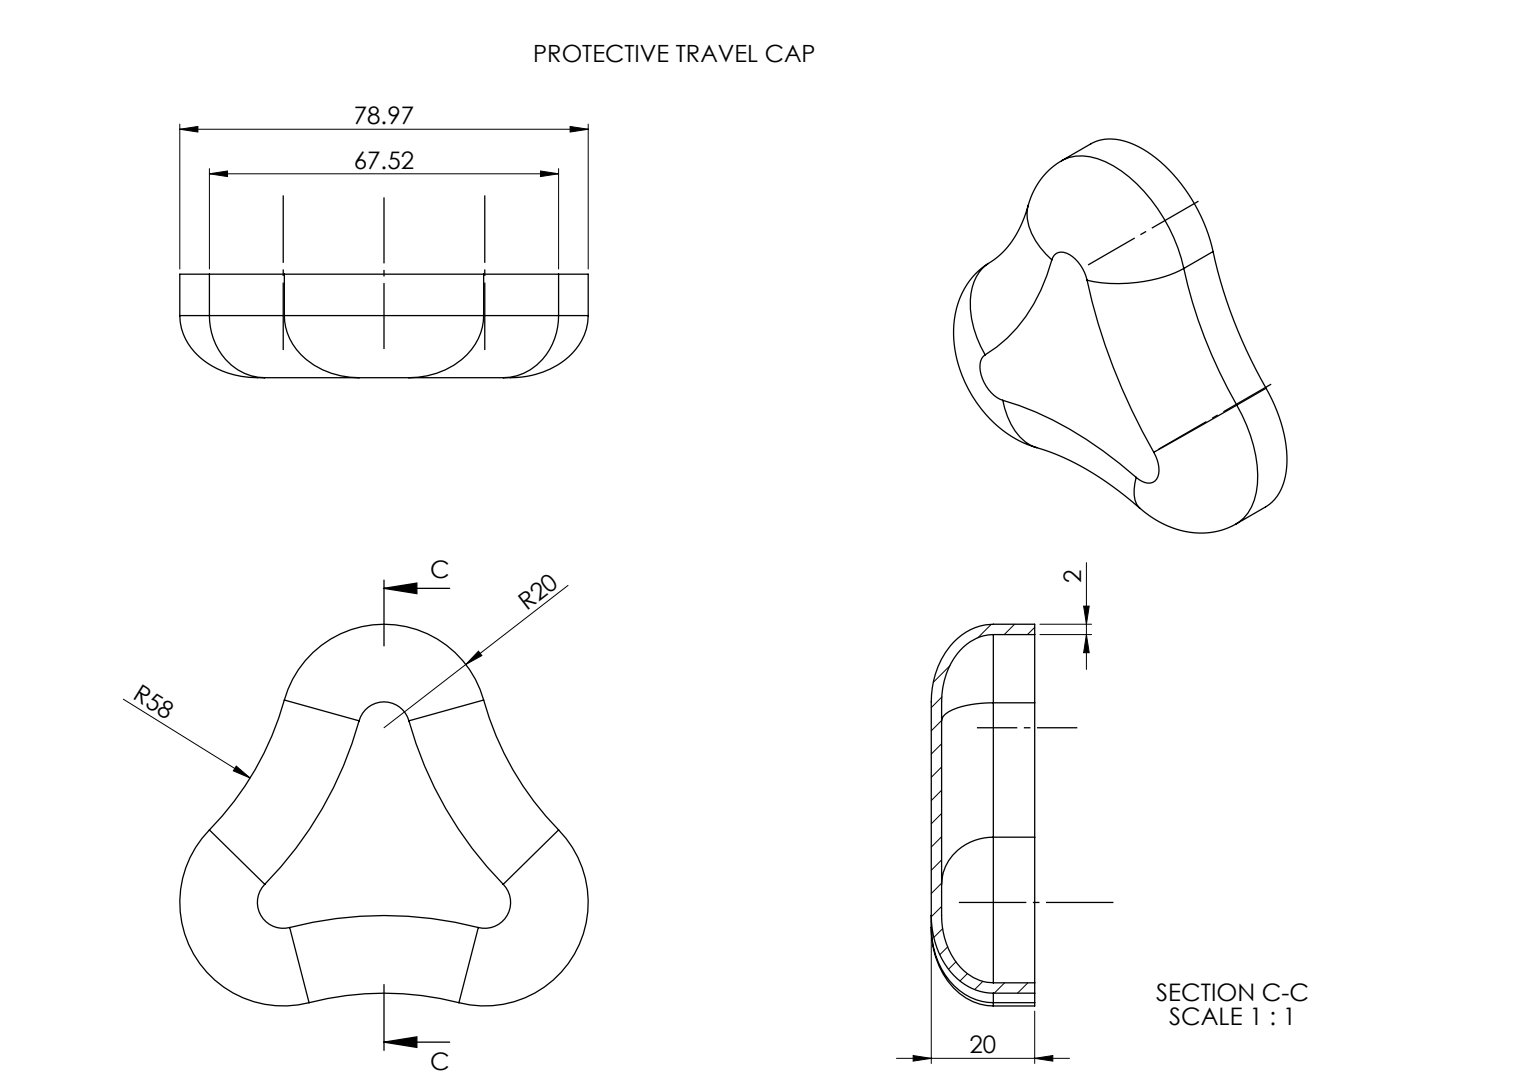
ISO-10303-21;
HEADER;
FILE_DESCRIPTION (('STEP AP214'),
    '1' );
FILE_NAME ('Protective Travel Cap.step',
    '2026-10-04T08:29:30',
    ( '' ),
    ( '' ),
    'SwSTEP 2.0',
    'SolidWorks 2026',
    '' );
FILE_SCHEMA (( 'AUTOMOTIVE_DESIGN' ));
ENDSEC;

DATA;
#17=CARTESIAN_POINT ( 'NONE',  ( 15.81286488304413318, 30.89881296429246760, 12.73282698324844375 ) ) ;
#18=CARTESIAN_POINT ( 'NONE',  ( 18.03924190088647705, -16.85603499720526344, 20.99999999999999645 ) ) ;
#20=CARTESIAN_POINT ( 'NONE',  ( -6.855490822441467458, 29.74656830693323073, 20.25080042701618765 ) ) ;
#37=CARTESIAN_POINT ( 'NONE',  ( -34.17506821248604609, -14.20748230372643484, 17.42190598798392642 ) ) ;
#45=CARTESIAN_POINT ( 'NONE',  ( 5.050662510305749642, -26.77689918168226768, 11.00000000000000178 ) ) ;
#48=PRODUCT_DEFINITION_CONTEXT ( 'detailed design', #8302, 'design' ) ;
#61=CARTESIAN_POINT ( 'NONE',  ( 25.28418022016654021, -25.06680681775964104, 17.42190598798393708 ) ) ;
#75=CARTESIAN_POINT ( 'NONE',  ( 32.33143948541893309, 1.358872982500734405, 11.55979286843934872 ) ) ;
#85=CARTESIAN_POINT ( 'NONE',  ( -20.14416558653889666, -20.32661669692040007, 20.50957957746029336 ) ) ;
#98=ORIENTED_EDGE ( 'NONE', *, *, #25945, .F. ) ;
#112=CARTESIAN_POINT ( 'NONE',  ( 19.16157041420283491, -20.39791322820700259, 20.50957957746027915 ) ) ;
#120=CARTESIAN_POINT ( 'NONE',  ( -33.75875814100324135, 2.759858869446477403, 22.99999999999999645 ) ) ;
#133=CARTESIAN_POINT ( 'NONE',  ( 29.92393930195780527, -26.04303208588360263, 11.00000000000002132 ) ) ;
#144=CARTESIAN_POINT ( 'NONE',  ( -35.54328883424743424, -18.34041411986772019, 13.92931973827826297 ) ) ;
#153=CARTESIAN_POINT ( 'NONE',  ( -20.57776646309937263, 11.88057900678980872, 17.42190598798392998 ) ) ;
#154=VECTOR ( 'NONE', #35200, 1000.000000000000000 ) ;
#161=CARTESIAN_POINT ( 'NONE',  ( 35.73872160561271727, -18.42674013420386459, 13.32518128616613140 ) ) ;
#182=CARTESIAN_POINT ( 'NONE',  ( -2.109373541296176047, 27.06550157850341520, 23.00000000000000000 ) ) ;
#217=CARTESIAN_POINT ( 'NONE',  ( 5.726446540400058183, 39.49945686212564055, 12.14047268033097460 ) ) ;
#221=CARTESIAN_POINT ( 'NONE',  ( 10.34254640628217992, 25.37474234120047001, 19.99202127657103389 ) ) ;
#240=CARTESIAN_POINT ( 'NONE',  ( -22.07435099023991043, -25.45711610480719145, 17.92354375535213151 ) ) ;
#256=DIRECTION ( 'NONE',  ( 0.000000000000000000, 0.000000000000000000, 1.000000000000000000 ) ) ;
#263=CARTESIAN_POINT ( 'NONE',  ( 33.08368474897510225, -6.388390677200520784, 17.92354375535212085 ) ) ;
#268=CARTESIAN_POINT ( 'NONE',  ( 4.441848239913406715, 24.85865334748807953, 21.00000000000000355 ) ) ;
#275=CARTESIAN_POINT ( 'NONE',  ( 17.89938016353245942, 22.15910768081766946, 14.53008259252595025 ) ) ;
#282=ORIENTED_EDGE ( 'NONE', *, *, #11860, .T. ) ;
#285=CARTESIAN_POINT ( 'NONE',  ( -27.67544922579230615, -7.282050787523742130, 20.50957957746029336 ) ) ;
#312=CARTESIAN_POINT ( 'NONE',  ( 27.76392016787571038, -12.00403709334112534, 20.69868183039782039 ) ) ;
#321=CARTESIAN_POINT ( 'NONE',  ( -19.26948696230206082, 27.85601271560033609, 11.00000000000000000 ) ) ;
#346=CARTESIAN_POINT ( 'NONE',  ( -15.07283634910000814, -28.35394831540519789, 13.32518128616608877 ) ) ;
#358=CARTESIAN_POINT ( 'NONE',  ( -13.22866120779437438, 26.17694675927630499, 18.42518152272108978 ) ) ;
#364=CARTESIAN_POINT ( 'NONE',  ( 15.12590024503159114, -28.14827041158712717, 13.92931973827808889 ) ) ;
#373=CARTESIAN_POINT ( 'NONE',  ( 27.36225479881369793, 10.16098284217389924, 11.00000000000000000 ) ) ;
#387=CARTESIAN_POINT ( 'NONE',  ( -8.437494165185018602, 40.76200631401457031, 11.00000000000000000 ) ) ;
#399=DIRECTION ( 'NONE',  ( -0.000000000000000000, -0.000000000000000000, -1.000000000000000000 ) ) ;
#419=CARTESIAN_POINT ( 'NONE',  ( 14.61820604905140897, 32.41591307681830614, 13.32518128616609765 ) ) ;
#423=CARTESIAN_POINT ( 'NONE',  ( 11.83264664767333052, 25.78892025138632604, 19.27171037444156454 ) ) ;
#435=CARTESIAN_POINT ( 'NONE',  ( 14.98890121934557129, -28.67928442654206833, 11.55979286843934517 ) ) ;
#440=CARTESIAN_POINT ( 'NONE',  ( -29.75773323547239002, -22.90830468393550845, 16.87380292611442201 ) ) ;
#448=CARTESIAN_POINT ( 'NONE',  ( -10.09822582592840767, -27.41751403068705883, 11.00000000001392308 ) ) ;
#464=CARTESIAN_POINT ( 'NONE',  ( 32.73576105632422184, -2.961849131989182204, 16.87380292611480215 ) ) ;
#469=CARTESIAN_POINT ( 'NONE',  ( -4.672335726382759624, 24.36080358023105674, 20.99999999999999645 ) ) ;
#484=CARTESIAN_POINT ( 'NONE',  ( -26.84751477640364214, -17.98144108585655232, 20.25080042701566896 ) ) ;
#510=CARTESIAN_POINT ( 'NONE',  ( 26.56332897235214574, -4.302820985782148000, 20.25080042701566541 ) ) ;
#534=DIRECTION ( 'NONE',  ( -0.000000000000000000, -0.000000000000000000, -1.000000000000000000 ) ) ;
#542=CARTESIAN_POINT ( 'NONE',  ( -37.14493776307941175, -9.008680429016052926, 12.73282698324853079 ) ) ;
#551=CARTESIAN_POINT ( 'NONE',  ( 9.401525468405049324, 34.87112330957724282, 16.87380292611441490 ) ) ;
#553=ORIENTED_EDGE ( 'NONE', *, *, #25998, .T. ) ;
#556=CARTESIAN_POINT ( 'NONE',  ( -26.46356280842828212, 3.031871643958657714, 17.42190598798967827 ) ) ;
#558=CARTESIAN_POINT ( 'NONE',  ( 21.42047163595253778, -15.86044052053649978, 20.99999999999999645 ) ) ;
#562=CARTESIAN_POINT ( 'NONE',  ( 34.54872031832756818, -1.828101745486344187, 13.32518128616626640 ) ) ;
#615=CARTESIAN_POINT ( 'NONE',  ( -7.591957726968746378, 38.93640765974107154, 10.99999999999981526 ) ) ;
#619=CARTESIAN_POINT ( 'NONE',  ( 4.864422697791962236, 33.03032433378086807, 19.66345542862529427 ) ) ;
#636=CARTESIAN_POINT ( 'NONE',  ( -32.97049335004036408, -4.716631976066113729, 17.42190598798392998 ) ) ;
#658=CARTESIAN_POINT ( 'NONE',  ( 28.76760616113913827, -24.40467509901337451, 16.30093088680155233 ) ) ;
#663=CARTESIAN_POINT ( 'NONE',  ( 0.6269669233416744758, 28.28960257232503395, 20.99999999999998934 ) ) ;
#670=CARTESIAN_POINT ( 'NONE',  ( 28.79337657215373980, 4.963436916934907295, 11.55979286843148302 ) ) ;
#677=CARTESIAN_POINT ( 'NONE',  ( -23.91569629078610149, -19.26019901638321130, 20.50957957746006954 ) ) ;
#680=ORIENTED_EDGE ( 'NONE', *, *, #28784, .T. ) ;
#706=CARTESIAN_POINT ( 'NONE',  ( 23.63966112704433087, -21.14828014214163687, 19.99202127657103034 ) ) ;
#743=CARTESIAN_POINT ( 'NONE',  ( -37.00900745416922177, -9.025932648522855928, 13.32518128616608699 ) ) ;
#750=CARTESIAN_POINT ( 'NONE',  ( -3.366772934462026523, 37.76190412503627414, 16.87380292611445043 ) ) ;
#753=CARTESIAN_POINT ( 'NONE',  ( -23.79662817865075652, 0.8209266586187062842, 19.66345542862912765 ) ) ;
#756=CARTESIAN_POINT ( 'NONE',  ( 23.05386822411318803, -7.747535282638377652, 23.00000000000000000 ) ) ;
#759=CARTESIAN_POINT ( 'NONE',  ( 35.99085602461089195, -18.53811353976012555, 12.14047268033102611 ) ) ;
#811=CARTESIAN_POINT ( 'NONE',  ( -13.75539757512625272, 34.17605197834731712, 12.14047268033125171 ) ) ;
#814=CARTESIAN_POINT ( 'NONE',  ( 7.971538940948045493, 30.92644086612910570, 19.66345542862527651 ) ) ;
#834=CARTESIAN_POINT ( 'NONE',  ( -35.08888820711664636, -5.671254737730515139, 15.72805884748985861 ) ) ;
#837=ORIENTED_EDGE ( 'NONE', *, *, #21012, .F. ) ;
#854=CARTESIAN_POINT ( 'NONE',  ( -17.47510495690846355, -31.20661830902342615, 11.00000000000000000 ) ) ;
#859=CARTESIAN_POINT ( 'NONE',  ( 35.14638740386845939, -7.516303343517492408, 16.30093088680192892 ) ) ;
#862=CARTESIAN_POINT ( 'NONE',  ( -14.95773623274140895, 28.45553334944834489, 16.30093088680134983 ) ) ;
#864=CARTESIAN_POINT ( 'NONE',  ( -3.456468065140321233, 26.15323006594350019, 20.99999999999998934 ) ) ;
#873=CARTESIAN_POINT ( 'NONE',  ( 14.67741354573947810, 20.96472719003773477, 18.42518152271840037 ) ) ;
#882=CARTESIAN_POINT ( 'NONE',  ( -29.20803623499946511, -13.20745421916120499, 20.25080042701566541 ) ) ;
#903=CARTESIAN_POINT ( 'NONE',  ( -24.37759566069532724, -10.08322588119026797, 23.00000000000000000 ) ) ;
#909=CARTESIAN_POINT ( 'NONE',  ( 30.28108141855193480, -11.05112898844763514, 19.99202127657103034 ) ) ;
#918=FACE_OUTER_BOUND ( 'NONE', #33899, .T. ) ;
#929=ORIENTED_EDGE ( 'NONE', *, *, #21435, .F. ) ;
#935=DIRECTION ( 'NONE',  ( -0.000000000000000000, -0.000000000000000000, -1.000000000000000000 ) ) ;
#945=CARTESIAN_POINT ( 'NONE',  ( -37.38745755834736428, -10.91949489986329347, 12.73282698324913831 ) ) ;
#952=CARTESIAN_POINT ( 'NONE',  ( -15.33540831873584587, 35.51988610398909429, 10.99999999999999822 ) ) ;
#953=CARTESIAN_POINT ( 'NONE',  ( -7.449887436100933513, 34.87105630051663496, 17.92354375535170874 ) ) ;
#958=CARTESIAN_POINT ( 'NONE',  ( -14.79097147050020311, 14.99953367534935822, 19.66345542862526585 ) ) ;
#960=CARTESIAN_POINT ( 'NONE',  ( 20.92112759555554291, -16.07000418475260162, 20.99999999999999645 ) ) ;
#963=CARTESIAN_POINT ( 'NONE',  ( 37.52525227335095082, -10.91693234368658061, 12.14047268033090532 ) ) ;
#1004=ORIENTED_EDGE ( 'NONE', *, *, #36950, .F. ) ;
#1007=CARTESIAN_POINT ( 'NONE',  ( -29.28423149095162259, -1.632116715639065463, 18.42518152272108978 ) ) ;
#1021=CARTESIAN_POINT ( 'NONE',  ( -6.977707682421693924, 31.68171018602201983, 19.66345542862527651 ) ) ;
#1034=CARTESIAN_POINT ( 'NONE',  ( 2.594149110900750621, 26.80855565015184894, 20.99999999999999289 ) ) ;
#1040=CARTESIAN_POINT ( 'NONE',  ( -35.58257249438602798, -10.95300747732907354, 16.30093088680272118 ) ) ;
#1062=CARTESIAN_POINT ( 'NONE',  ( 35.36447994912680315, -9.234655410422998756, 16.30093088680190760 ) ) ;
#1064=CARTESIAN_POINT ( 'NONE',  ( -3.569741787452771042, 38.68155838841067151, 15.72805884748945715 ) ) ;
#1067=CARTESIAN_POINT ( 'NONE',  ( -1.596172877504954402, 27.23837864096127959, 20.99999999999999645 ) ) ;
#1077=CARTESIAN_POINT ( 'NONE',  ( 17.25967040852637169, 21.92197836105680864, 15.72805884747922889 ) ) ;
#1086=CARTESIAN_POINT ( 'NONE',  ( -22.56822310031916956, -21.59793901597470978, 19.99202127657132522 ) ) ;
#1112=CARTESIAN_POINT ( 'NONE',  ( 17.92913371968424840, -21.93458435334546408, 19.99202127657079942 ) ) ;
#1135=CARTESIAN_POINT ( 'NONE',  ( -21.72603204741356109, -16.58852365944958862, 20.99999999999999645 ) ) ;
#1139=VERTEX_POINT ( 'NONE', #39839 ) ;
#1145=CARTESIAN_POINT ( 'NONE',  ( -35.38210723591855356, -3.548218742175161200, 13.32518128616608877 ) ) ;
#1154=CARTESIAN_POINT ( 'NONE',  ( -10.35750558342918737, 33.44896173339029133, 17.42190598798475065 ) ) ;
#1159=CARTESIAN_POINT ( 'NONE',  ( -9.534329713701904296, 19.05805734593735679, 20.69868183039760368 ) ) ;
#1164=CARTESIAN_POINT ( 'NONE',  ( 37.45384686740442248, -12.88771083438643927, 12.14047268033111671 ) ) ;
#1204=EDGE_LOOP ( 'NONE', ( #35292, #7584, #15851, #28195 ) ) ;
#1210=CARTESIAN_POINT ( 'NONE',  ( -32.09165771328038375, 1.123514972298483405, 13.32518128616608344 ) ) ;
#1224=CARTESIAN_POINT ( 'NONE',  ( -7.430899969937648564, 32.27804933232874873, 19.27171037444156099 ) ) ;
#1243=CARTESIAN_POINT ( 'NONE',  ( -20.67781403882173663, -27.68125770801090013, 15.72805884748939498 ) ) ;
#1260=CARTESIAN_POINT ( 'NONE',  ( -30.53342463661827821, -27.99077457432856875, 11.00000000000000178 ) ) ;
#1264=CARTESIAN_POINT ( 'NONE',  ( 32.49165476041698497, -0.9821698610445067645, 15.72805884749123351 ) ) ;
#1266=CARTESIAN_POINT ( 'NONE',  ( -13.24632657851083550, 31.48533120267438079, 16.30093088680190050 ) ) ;
#1267=CARTESIAN_POINT ( 'NONE',  ( -5.218261001347021200, -24.78318996519343997, 16.30093088680190760 ) ) ;
#1269=CARTESIAN_POINT ( 'NONE',  ( 5.067518982750386591, 26.80212859219470189, 20.94377226548378346 ) ) ;
#1274=PRODUCT_DEFINITION_SHAPE ( 'NONE', 'NONE',  #3314 ) ;
#1276=CARTESIAN_POINT ( 'NONE',  ( 19.49168883800135532, 11.25353179758032063, 18.42518152272108978 ) ) ;
#1284=CARTESIAN_POINT ( 'NONE',  ( -29.14609120334281300, -6.569533100116839108, 19.99202127657103389 ) ) ;
#1305=CARTESIAN_POINT ( 'NONE',  ( -33.75875814100331951, 2.759858869446532470, 23.00000000000000000 ) ) ;
#1311=CARTESIAN_POINT ( 'NONE',  ( 28.87886971313727003, -7.891952902956772320, 20.25080042701540251 ) ) ;
#1333=CARTESIAN_POINT ( 'NONE',  ( -24.38721429972438770, -12.23686305972948318, 20.99999999999999645 ) ) ;
#1335=CARTESIAN_POINT ( 'NONE',  ( -19.48557158514998022, -11.24999999999982414, 23.00000000000000000 ) ) ;
#1343=CARTESIAN_POINT ( 'NONE',  ( -16.87498849720621763, -29.16588574430760517, 11.55979286843870035 ) ) ;
#1351=CARTESIAN_POINT ( 'NONE',  ( -37.48557158514991272, -11.24999999999982414, 23.00000000000000000 ) ) ;
#1353=CARTESIAN_POINT ( 'NONE',  ( -1.621626408466260161, 37.48425883190013508, 17.42190598798392642 ) ) ;
#1357=CARTESIAN_POINT ( 'NONE',  ( -8.768078002824983841, 24.93711404285093991, 20.50957957746029336 ) ) ;
#1359=CARTESIAN_POINT ( 'NONE',  ( 24.08646667827959220, -13.28101593840520600, 20.99999999999999645 ) ) ;
#1364=CARTESIAN_POINT ( 'NONE',  ( 32.80061120326785584, -23.42582577749432104, 12.14047268033107407 ) ) ;
#1375=CARTESIAN_POINT ( 'NONE',  ( 17.34253826607195847, 27.32041144403996569, 11.55979286843935405 ) ) ;
#1397=ORIENTED_EDGE ( 'NONE', *, *, #13984, .F. ) ;
#1408=CARTESIAN_POINT ( 'NONE',  ( -32.28722999652026004, 1.315479119632481098, 12.14047268033097637 ) ) ;
#1417=CARTESIAN_POINT ( 'NONE',  ( -1.947644445291408566, 40.50000000000003553, 10.99999999999999822 ) ) ;
#1420=CARTESIAN_POINT ( 'NONE',  ( 13.22866120778972210, 26.17694675929306314, 18.42518152272108622 ) ) ;
#1430=ORIENTED_EDGE ( 'NONE', *, *, #13824, .F. ) ;
#1438=CARTESIAN_POINT ( 'NONE',  ( -18.89970378041276788, -27.81027634888826938, 15.72805884748982130 ) ) ;
#1464=CARTESIAN_POINT ( 'NONE',  ( 29.26100170765755948, -25.10377279866101929, 15.13084544680181942 ) ) ;
#1466=CARTESIAN_POINT ( 'NONE',  ( 6.948689594652316615, 37.54332414141804719, 15.72805884748934169 ) ) ;
#1467=CARTESIAN_POINT ( 'NONE',  ( 4.318754312355916755E-14, -23.13411080437162326, 17.92354375535250810 ) ) ;
#1469=CARTESIAN_POINT ( 'NONE',  ( 8.768078002822827344, 24.93711404285870614, 20.50957957746029692 ) ) ;
#1478=CARTESIAN_POINT ( 'NONE',  ( 24.95394407858722374, 1.780357051442290839, 18.87996532026972218 ) ) ;
#1486=CARTESIAN_POINT ( 'NONE',  ( -31.78757023779102298, -12.37085478034622810, 19.27171037444157875 ) ) ;
#1500=CARTESIAN_POINT ( 'NONE',  ( 34.33271597229073535, -24.82403720151181759, 23.00000000000093792 ) ) ;
#1511=CARTESIAN_POINT ( 'NONE',  ( 32.25947621352486294, -13.82181017473358331, 18.87996532025784546 ) ) ;
#1533=CARTESIAN_POINT ( 'NONE',  ( 10.09822582592851603, -27.41751403068707660, 11.00000000000204814 ) ) ;
#1537=CARTESIAN_POINT ( 'NONE',  ( -21.42047163595255910, -15.86044052053618003, 20.99999999999999645 ) ) ;
#1548=CARTESIAN_POINT ( 'NONE',  ( -29.92393930196035612, -26.04303208588115126, 11.55979286843952103 ) ) ;
#1561=CARTESIAN_POINT ( 'NONE',  ( -19.99288511733821139, -2.332377806177347690, 20.94377226548488125 ) ) ;
#1563=CARTESIAN_POINT ( 'NONE',  ( 23.10579450714144301, -17.79557859931273356, 20.82122704794064916 ) ) ;
#1568=CARTESIAN_POINT ( 'NONE',  ( 36.55626306615705090, -16.65168930787738688, 12.73282698324840823 ) ) ;
#1572=DIRECTION ( 'NONE',  ( -0.000000000000000000, -0.000000000000000000, -1.000000000000000000 ) ) ;
#1624=( BOUNDED_CURVE ( )  B_SPLINE_CURVE ( 2, ( #20187, #30129, #14483 ),
 .UNSPECIFIED., .F., .F. ) 
 B_SPLINE_CURVE_WITH_KNOTS ( ( 3, 3 ),
 ( 0.000000000000000000, 1.000000000000000000 ),
 .UNSPECIFIED. ) 
 CURVE ( )  GEOMETRIC_REPRESENTATION_ITEM ( )  RATIONAL_B_SPLINE_CURVE ( ( 1.000000000000000000, 0.7071067811865474617, 1.000000000000000000 ) ) 
 REPRESENTATION_ITEM ( '' )  );
#1625=CARTESIAN_POINT ( 'NONE',  ( 9.924110812760721601, 32.99075218357499750, 17.92354375535250455 ) ) ;
#1638=CARTESIAN_POINT ( 'NONE',  ( 17.42101839920123041, -19.25229542401860527, 20.69868183039781329 ) ) ;
#1643=CARTESIAN_POINT ( 'NONE',  ( -32.48135758214319679, -20.75321993593849257, 16.30093088680156299 ) ) ;
#1660=CARTESIAN_POINT ( 'NONE',  ( -14.98890121934603314, -28.67928442654204346, 11.00000000000000000 ) ) ;
#1667=CARTESIAN_POINT ( 'NONE',  ( 36.30242391553733228, -14.63578948164456683, 14.53008259254010959 ) ) ;
#1669=CARTESIAN_POINT ( 'NONE',  ( 11.65184672541106359, 34.81748849094131515, 15.13084544680210719 ) ) ;
#1670=CARTESIAN_POINT ( 'NONE',  ( 4.272934335498898793E-14, -21.05812563137664739, 19.27171037444156809 ) ) ;
#1672=CARTESIAN_POINT ( 'NONE',  ( -6.367390439426523940, 24.26983560722021949, 20.94377226548378346 ) ) ;
#1683=CARTESIAN_POINT ( 'NONE',  ( 30.57450045108190650, -0.3656520783221823279, 16.87380292611441490 ) ) ;
#1693=CARTESIAN_POINT ( 'NONE',  ( -27.14644468510475406, -3.730463242939707769, 19.99202127657103389 ) ) ;
#1706=CARTESIAN_POINT ( 'NONE',  ( 25.22779562677032672, -30.53001673900870472, 23.00000000000093792 ) ) ;
#1711=CARTESIAN_POINT ( 'NONE',  ( -23.54493052986492430, -14.21898406159475137, 23.00000000000000000 ) ) ;
#1720=CARTESIAN_POINT ( 'NONE',  ( 30.40813597975501636, -7.345136026722032696, 19.66345542862497098 ) ) ;
#1722=EDGE_LOOP ( 'NONE', ( #16171, #11373, #19448, #17460 ) ) ;
#1730=ADVANCED_FACE ( 'NONE', ( #29809 ), #39146, .F. ) ;
#1734=CYLINDRICAL_SURFACE ( 'NONE', #3431, 20.00000000000003908 ) ;
#1744=CARTESIAN_POINT ( 'NONE',  ( -22.84262768307197788, -16.00844090263207065, 21.00000000000000000 ) ) ;
#1754=CARTESIAN_POINT ( 'NONE',  ( -20.78821643698918109, -29.20280246618806430, 11.55979286843934872 ) ) ;
#1760=CARTESIAN_POINT ( 'NONE',  ( 13.82587227205762481, 37.11292025503284009, 11.00000000000000000 ) ) ;
#1765=CARTESIAN_POINT ( 'NONE',  ( -26.56332897234805301, -4.302820985777816354, 20.25080042701566541 ) ) ;
#1766=CARTESIAN_POINT ( 'NONE',  ( 18.64638308222462371, -17.01267446048655430, 20.99999999999995026 ) ) ;
#1778=FACE_OUTER_BOUND ( 'NONE', #29743, .T. ) ;
#1796=CARTESIAN_POINT ( 'NONE',  ( -24.22337021529747147, -9.561219044741108064, 22.99999999999999289 ) ) ;
#1829=CARTESIAN_POINT ( 'NONE',  ( 8.307596863005482390, 33.43166269068607477, 18.42518152272108978 ) ) ;
#1850=CARTESIAN_POINT ( 'NONE',  ( -29.60586052328872597, -25.59238499872923711, 13.92931973827819725 ) ) ;
#1875=CARTESIAN_POINT ( 'NONE',  ( 34.08416769313340211, -19.67850339273466176, 15.13084544680213739 ) ) ;
#1877=CARTESIAN_POINT ( 'NONE',  ( -5.476246462222815303, 38.75671607062959367, 14.53008259254010959 ) ) ;
#1878=CARTESIAN_POINT ( 'NONE',  ( -10.51283450064414637, -24.98199432659117747, 16.87380292611976884 ) ) ;
#1880=CARTESIAN_POINT ( 'NONE',  ( 3.486159013132950513, 30.04627872069376338, 20.69868183039781684 ) ) ;
#1888=CARTESIAN_POINT ( 'NONE',  ( 15.48226359616410086, 8.938689054910316401, 20.50957957746029336 ) ) ;
#1891=CARTESIAN_POINT ( 'NONE',  ( -3.900486991066764553, 40.17991855517990274, 11.00000000000018474 ) ) ;
#1899=CARTESIAN_POINT ( 'NONE',  ( -29.95834561893252612, -4.698932123269424999, 19.27171037444122703 ) ) ;
#1912=DIRECTION ( 'NONE',  ( -0.000000000000000000, -0.000000000000000000, -1.000000000000000000 ) ) ;
#1917=CARTESIAN_POINT ( 'NONE',  ( -25.22779562677360232, -30.53001673900768864, 11.00000000000000000 ) ) ;
#1924=CARTESIAN_POINT ( 'NONE',  ( 29.45678984391886246, -18.54179626184217611, 19.27171037444156454 ) ) ;
#1946=FACE_OUTER_BOUND ( 'NONE', #40149, .T. ) ;
#1950=CARTESIAN_POINT ( 'NONE',  ( -24.49409870380020848, -11.70597971641812407, 20.99999999999999645 ) ) ;
#1961=CARTESIAN_POINT ( 'NONE',  ( -35.07402885326980879, -20.24999999999981881, 11.00000000000000000 ) ) ;
#1965=ORIENTED_EDGE ( 'NONE', *, *, #20027, .T. ) ;
#1975=CARTESIAN_POINT ( 'NONE',  ( -25.38348611796302734, -5.460896781494596119, 20.69868183039781329 ) ) ;
#1977=CARTESIAN_POINT ( 'NONE',  ( 25.96434769773125240, -12.55439225991619701, 20.94377226548379411 ) ) ;
#2000=CARTESIAN_POINT ( 'NONE',  ( -14.48927117870118408, -30.61587158504671535, 23.00000000000000355 ) ) ;
#2049=CARTESIAN_POINT ( 'NONE',  ( -36.43809855126085750, -10.93713533239294300, 15.13084544680293497 ) ) ;
#2071=CARTESIAN_POINT ( 'NONE',  ( 36.37100582830206719, -12.78888441968064349, 15.13084544680218002 ) ) ;
#2073=CARTESIAN_POINT ( 'NONE',  ( -10.37941170769518529, 36.15788802554169479, 14.53008259254010959 ) ) ;
#2075=CARTESIAN_POINT ( 'NONE',  ( -10.35515495760927784, -25.90830221534925926, 15.72805884749706529 ) ) ;
#2077=CARTESIAN_POINT ( 'NONE',  ( -2.638259136957760820, 30.33190274691516208, 20.69868183039781329 ) ) ;
#2085=CARTESIAN_POINT ( 'NONE',  ( 12.58275666885947075, 13.96078236990229016, 20.50957957746036442 ) ) ;
#2096=CARTESIAN_POINT ( 'NONE',  ( -33.23893881994145261, -12.50319288011963081, 18.42518152272109688 ) ) ;
#2111=CARTESIAN_POINT ( 'NONE',  ( 23.19735768193459791, -14.64350930037804055, 23.00000000000000000 ) ) ;
#2115=CARTESIAN_POINT ( 'NONE',  ( -34.33271597228890215, -24.82403720151341986, 11.00000000000000000 ) ) ;
#2119=CARTESIAN_POINT ( 'NONE',  ( 29.86387254395472723, -6.221772116352023652, 19.66345542862529783 ) ) ;
#2140=CARTESIAN_POINT ( 'NONE',  ( 15.27443809246256734, -27.57253143578338594, 15.13084544680213561 ) ) ;
#2143=CARTESIAN_POINT ( 'NONE',  ( -25.35679574134486813, -6.615406304683630445, 20.82122704794080548 ) ) ;
#2153=CARTESIAN_POINT ( 'NONE',  ( -32.84658669524026919, -23.46788009898592264, 10.99999999999981881 ) ) ;
#2157=CARTESIAN_POINT ( 'NONE',  ( -23.43324262027537586, -8.134040356058612531, 20.99999999999999289 ) ) ;
#2169=CARTESIAN_POINT ( 'NONE',  ( 20.82679397340719873, -18.60878629326332501, 20.82122704794080903 ) ) ;
#2188=CARTESIAN_POINT ( 'NONE',  ( 18.23649648353778474, -16.09146789626167262, 23.00000000000000000 ) ) ;
#2201=CARTESIAN_POINT ( 'NONE',  ( 18.77248996150425597, -31.35432035810270435, 11.00000000000000178 ) ) ;
#2202=MECHANICAL_DESIGN_GEOMETRIC_PRESENTATION_REPRESENTATION('',(#9960),#2829);
#2213=CARTESIAN_POINT ( 'NONE',  ( -24.77298340259705256, 8.359746025953324278, 15.13084544680308419 ) ) ;
#2232=DIRECTION ( 'NONE',  ( -0.000000000000000000, -0.000000000000000000, -1.000000000000000000 ) ) ;
#2250=ORIENTED_EDGE ( 'NONE', *, *, #9412, .T. ) ;
#2268=CARTESIAN_POINT ( 'NONE',  ( 32.59722377598627219, -23.23978988006441782, 13.32518128616629305 ) ) ;
#2270=CARTESIAN_POINT ( 'NONE',  ( 3.781581747449316744, 39.64129210796443203, 13.92931973827821146 ) ) ;
#2274=CARTESIAN_POINT ( 'NONE',  ( 5.140622461635829588, 27.93365566737693229, 20.82122704794079837 ) ) ;
#2282=CARTESIAN_POINT ( 'NONE',  ( 12.61496056324080683, 7.283250877003740520, 20.99999999999999645 ) ) ;
#2285=CARTESIAN_POINT ( 'NONE',  ( -12.44178368932702661, 35.65276919562055014, 11.00000000000005684 ) ) ;
#2295=CARTESIAN_POINT ( 'NONE',  ( -30.59707569446036501, -4.299442758149942811, 18.87996532025748309 ) ) ;
#2309=CARTESIAN_POINT ( 'NONE',  ( 23.43324262027504190, -8.134040356058543253, 23.00000000000000000 ) ) ;
#2318=CARTESIAN_POINT ( 'NONE',  ( 31.03731131719052883, -12.30244853585591969, 19.66345542862526230 ) ) ;
#2330=EDGE_CURVE ( 'NONE', #31697, #24869, #30927, .T. ) ;
#2336=CARTESIAN_POINT ( 'NONE',  ( -4.817371740575545402, 23.83900317890010001, 20.99999999999999645 ) ) ;
#2341=CARTESIAN_POINT ( 'NONE',  ( 10.10865978838830515, -27.35622988134924327, 12.14047268033177573 ) ) ;
#2342=ORIENTED_EDGE ( 'NONE', *, *, #2684, .F. ) ;
#2344=CARTESIAN_POINT ( 'NONE',  ( -26.53285431386355597, -6.841436363529350473, 20.69868183039763210 ) ) ;
#2372=CARTESIAN_POINT ( 'NONE',  ( 22.04303751225581465, -17.34387783897721746, 20.94377226548377280 ) ) ;
#2375=CARTESIAN_POINT ( 'NONE',  ( 37.51589702892713518, -12.89337557385772470, 11.00000000000017053 ) ) ;
#2387=CARTESIAN_POINT ( 'NONE',  ( 14.48927117870126580, -30.61587158504672601, 11.00000000000000000 ) ) ;
#2410=CARTESIAN_POINT ( 'NONE',  ( -27.61482536621095818, 3.986323854238359665, 15.72805884749610428 ) ) ;
#2430=CARTESIAN_POINT ( 'NONE',  ( -3.460024211650461368, 26.15060946995401281, 23.00000000000000355 ) ) ;
#2453=ORIENTED_EDGE ( 'NONE', *, *, #21012, .T. ) ;
#2458=ORIENTED_EDGE ( 'NONE', *, *, #16442, .T. ) ;
#2469=CARTESIAN_POINT ( 'NONE',  ( 34.36757128605636069, -1.941376724489949579, 13.92931973827832159 ) ) ;
#2472=CARTESIAN_POINT ( 'NONE',  ( 10.37941170769460975, 36.15788802554214953, 14.53008259254011136 ) ) ;
#2474=CARTESIAN_POINT ( 'NONE',  ( -17.21213525676645162, -20.06193531423545551, 20.50957957746029336 ) ) ;
#2476=CARTESIAN_POINT ( 'NONE',  ( 7.420252307063369024, 30.34362403113780715, 19.99202127657103745 ) ) ;
#2484=CARTESIAN_POINT ( 'NONE',  ( 20.63240589120021795, -1.802217369567702843, 20.82122704794562296 ) ) ;
#2495=CARTESIAN_POINT ( 'NONE',  ( -24.23816072143619493, -22.57437281311074528, 19.27171037444157164 ) ) ;
#2514=CARTESIAN_POINT ( 'NONE',  ( -18.77248997590677604, -31.35432035705904497, 23.00000000000094147 ) ) ;
#2519=CARTESIAN_POINT ( 'NONE',  ( 33.25367603494935764, -15.60696645161989160, 17.92354375535251521 ) ) ;
#2538=CARTESIAN_POINT ( 'NONE',  ( 4.264734420589964944E-14, -26.44091005802452798, 13.32518128616608877 ) ) ;
#2541=CARTESIAN_POINT ( 'NONE',  ( -17.83459896181207682, -17.64923967996745446, 20.94377226548378346 ) ) ;
#2551=CARTESIAN_POINT ( 'NONE',  ( -19.26948696230207858, 27.85601271560029701, 11.00000000000000000 ) ) ;
#2570=CARTESIAN_POINT ( 'NONE',  ( 27.67544922579167022, -7.282050787522788227, 20.50957957746029336 ) ) ;
#2582=CARTESIAN_POINT ( 'NONE',  ( 12.55429062395116446, 25.98950339719798563, 18.87996532025784546 ) ) ;
#2587=FILL_AREA_STYLE ('',( #24707 ) ) ;
#2600=CARTESIAN_POINT ( 'NONE',  ( 35.27612715351751405, 1.213969564528367906, 10.99999999999999822 ) ) ;
#2609=CARTESIAN_POINT ( 'NONE',  ( -20.66414367076651715, 17.76245163069309640, 11.55979286843749421 ) ) ;
#2656=CYLINDRICAL_SURFACE ( 'NONE', #9592, 58.00000000000007105 ) ;
#2662=CARTESIAN_POINT ( 'NONE',  ( 26.37421498764336292, -27.66411951031065541, 12.73282698324852902 ) ) ;
#2664=CARTESIAN_POINT ( 'NONE',  ( 16.30840571581194354, 28.99314201041919503, 13.92931973827851699 ) ) ;
#2666=CARTESIAN_POINT ( 'NONE',  ( -11.32166530368854929, -20.22988973188854800, 19.99202127657163430 ) ) ;
#2670=CARTESIAN_POINT ( 'NONE',  ( -5.569982264783402748, 31.74975025675326989, 19.99202127657043704 ) ) ;
#2678=CARTESIAN_POINT ( 'NONE',  ( 15.65370567419071079, 2.019989953579482744, 20.99999999999999645 ) ) ;
#2683=ORIENTED_EDGE ( 'NONE', *, *, #21322, .F. ) ;
#2684=EDGE_CURVE ( 'NONE', #24176, #17915, #31549, .T. ) ;
#2687=CARTESIAN_POINT ( 'NONE',  ( -23.42865034949355874, -24.48547250943464348, 18.42518152272145215 ) ) ;
#2710=VECTOR ( 'NONE', #23153, 1000.000000000000000 ) ;
#2711=CARTESIAN_POINT ( 'NONE',  ( 33.10646761238916014, -9.521241417579867417, 18.42518152272108622 ) ) ;
#2712=CIRCLE ( 'NONE', #25401, 19.99999999999993605 ) ;
#2719=CARTESIAN_POINT ( 'NONE',  ( -18.03924190088572388, -16.85603499720483001, 20.99999999999999645 ) ) ;
#2731=CARTESIAN_POINT ( 'NONE',  ( 10.09822582592846096, -27.41751403068768056, 11.55979286844081244 ) ) ;
#2734=CARTESIAN_POINT ( 'NONE',  ( -20.67756819927166134, -17.78966421867582781, 20.94377226548369109 ) ) ;
#2760=CARTESIAN_POINT ( 'NONE',  ( 21.85869495253959371, -19.21667513322869780, 20.69868183039798737 ) ) ;
#2761=CARTESIAN_POINT ( 'NONE',  ( 19.48557158514982746, -11.25000000000009415, 3.000000000000000000 ) ) ;
#2793=CARTESIAN_POINT ( 'NONE',  ( -30.82617745331405246, -24.12092658898454189, 14.53008259254011492 ) ) ;
#2803=CARTESIAN_POINT ( 'NONE',  ( -20.60789226802554808, 17.73598670051888604, 12.14047268032921956 ) ) ;
#2820=ORIENTED_EDGE ( 'NONE', *, *, #6864, .F. ) ;
#2829=( GEOMETRIC_REPRESENTATION_CONTEXT ( 3 ) GLOBAL_UNCERTAINTY_ASSIGNED_CONTEXT ( ( #10802 ) ) GLOBAL_UNIT_ASSIGNED_CONTEXT ( ( #25494, #37301, #31402 ) ) REPRESENTATION_CONTEXT ( 'NONE', 'WORKASPACE' ) );
#2833=FACE_OUTER_BOUND ( 'NONE', #21196, .T. ) ;
#2864=CARTESIAN_POINT ( 'NONE',  ( 1.940950748631622647, 40.43805239114133343, 12.14047268033097815 ) ) ;
#2865=CARTESIAN_POINT ( 'NONE',  ( 6.008588623656380356, -15.38567963534269900, 20.94377226548378701 ) ) ;
#2868=CARTESIAN_POINT ( 'NONE',  ( -8.231369907346209658, 29.48764348321983420, 19.99202127657101258 ) ) ;
#2885=CARTESIAN_POINT ( 'NONE',  ( -28.60197298176802860, -19.58586899272916781, 19.27171037444157520 ) ) ;
#2903=EDGE_LOOP ( 'NONE', ( #37586, #21867, #5252, #24338, #553 ) ) ;
#2907=CARTESIAN_POINT ( 'NONE',  ( 24.28032989564875876, -12.76774640304083164, 21.00000000000001066 ) ) ;
#2908=CARTESIAN_POINT ( 'NONE',  ( 25.04152548477498996, -24.48861404543278653, 17.92354375535251521 ) ) ;
#2919=( BOUNDED_SURFACE ( )  B_SPLINE_SURFACE ( 2, 3, ( 
 ( #5150, #20799, #20193, #8194, #20601, #32999, #29930, #2111, #5348, #38674, #29330, #8596, #10847, #20993, #30136, #14695, #2309, #27086 ),
 ( #23239, #39475, #35632, #11654, #1706, #33401, #5542, #1500, #7790, #32589, #4748, #17155, #14086, #21385, #30542, #18152, #15288, #33792 ),
 ( #17953, #12639, #12042, #28073, #6138, #30338, #27676, #34380, #3097, #18343, #27479, #40063, #8802, #15492, #24630, #33594, #31130, #36825 ) ),
 .UNSPECIFIED., .F., .F., .F. ) 
 B_SPLINE_SURFACE_WITH_KNOTS ( ( 3, 3 ),
 ( 4, 2, 2, 2, 2, 2, 2, 2, 4 ),
 ( 0.000000000000000000, 1.000000000000000000 ),
 ( 4.459899766721548531, 4.784821457936484279, 5.109743149151420027, 5.434664840366355776, 5.759586531581291524, 6.084508222796227273, 6.409429914011163021, 6.734351605226098769, 7.059273296441033629 ),
 .UNSPECIFIED. ) 
 GEOMETRIC_REPRESENTATION_ITEM ( )  RATIONAL_B_SPLINE_SURFACE ( (
 ( 1.000000000000000000, 1.000000000000000000, 1.000000000000000000, 1.000000000000000000, 1.000000000000000000, 1.000000000000000000, 1.000000000000000000, 1.000000000000000000, 1.000000000000000000, 1.000000000000000000, 1.000000000000000000, 1.000000000000000000, 1.000000000000000000, 1.000000000000000000, 1.000000000000000000, 1.000000000000000000, 1.000000000000000000, 1.000000000000000000),
 ( 0.7071067811865474617, 0.7071067811865474617, 0.7071067811865474617, 0.7071067811865474617, 0.7071067811865475727, 0.7071067811865475727, 0.7071067811865475727, 0.7071067811865475727, 0.7071067811865474617, 0.7071067811865474617, 0.7071067811865474617, 0.7071067811865474617, 0.7071067811865474617, 0.7071067811865474617, 0.7071067811865474617, 0.7071067811865474617, 0.7071067811865475727, 0.7071067811865475727),
 ( 1.000000000000000000, 1.000000000000000000, 1.000000000000000000, 1.000000000000000000, 1.000000000000000000, 1.000000000000000000, 1.000000000000000000, 1.000000000000000000, 1.000000000000000000, 1.000000000000000000, 1.000000000000000000, 1.000000000000000000, 1.000000000000000000, 1.000000000000000000, 1.000000000000000000, 1.000000000000000000, 1.000000000000000000, 1.000000000000000000) ) ) 
 REPRESENTATION_ITEM ( '' )  SURFACE ( )  );
#2922=CARTESIAN_POINT ( 'NONE',  ( 25.55085611915419364, 8.900480655592511781, 12.73282698324917384 ) ) ;
#2930=ORIENTED_EDGE ( 'NONE', *, *, #20002, .F. ) ;
#2932=CARTESIAN_POINT ( 'NONE',  ( -24.40183261524807889, -16.82966968839920341, 20.82122704794079837 ) ) ;
#2943=CARTESIAN_POINT ( 'NONE',  ( -14.98890121934612019, -28.67928442654180898, 11.00000000000000000 ) ) ;
#2962=CARTESIAN_POINT ( 'NONE',  ( 24.76266088601874671, -18.72941319223726353, 20.50957957746007310 ) ) ;
#2979=CARTESIAN_POINT ( 'NONE',  ( 6.143904198944455608, -13.77689918168226235, 23.00000000000000000 ) ) ;
#2991=CARTESIAN_POINT ( 'NONE',  ( 27.14644468510626396, -3.730463242941437940, 19.99202127657103745 ) ) ;
#2996=CARTESIAN_POINT ( 'NONE',  ( -36.96658581397586119, -12.84323481469905204, 13.92931973827791836 ) ) ;
#3005=FACE_OUTER_BOUND ( 'NONE', #22440, .T. ) ;
#3008=CARTESIAN_POINT ( 'NONE',  ( 20.91702953749078020, -16.07165331220364735, 23.00000000000000355 ) ) ;
#3030=CARTESIAN_POINT ( 'NONE',  ( 3.456468065140020141, 26.15323006594238464, 23.00000000000000000 ) ) ;
#3050=DIRECTION ( 'NONE',  ( -0.000000000000000000, -0.000000000000000000, -1.000000000000000000 ) ) ;
#3059=CARTESIAN_POINT ( 'NONE',  ( -14.61820604905143384, 32.41591307681827061, 13.32518128616608699 ) ) ;
#3060=CARTESIAN_POINT ( 'NONE',  ( 11.59681349796545824, -18.61320969074927945, 20.50957957745985993 ) ) ;
#3062=CARTESIAN_POINT ( 'NONE',  ( 11.11100267139549658, 25.58833710557466290, 19.66345542862528362 ) ) ;
#3068=CARTESIAN_POINT ( 'NONE',  ( -15.87271491999997863, 26.91186955879524945, 15.72805884748939498 ) ) ;
#3083=CARTESIAN_POINT ( 'NONE',  ( -27.81120771500161837, -23.04947625254830967, 17.92354375535251876 ) ) ;
#3097=CARTESIAN_POINT ( 'NONE',  ( 35.72300736400885057, -23.12593624637960588, 11.00000000000000000 ) ) ;
#3109=CARTESIAN_POINT ( 'NONE',  ( 31.91928157790820109, -18.42860581134451792, 17.92354375535250810 ) ) ;
#3130=CARTESIAN_POINT ( 'NONE',  ( -27.09004689510899766, -14.60731774717074138, 20.69868183039799803 ) ) ;
#3141=ORIENTED_EDGE ( 'NONE', *, *, #7856, .F. ) ;
#3158=EDGE_CURVE ( 'NONE', #10973, #10557, #6006, .T. ) ;
#3160=CARTESIAN_POINT ( 'NONE',  ( 20.97602320185162839, -19.42790811720868049, 20.69868183039782750 ) ) ;
#3170=CARTESIAN_POINT ( 'NONE',  ( -27.36225479880417311, 10.16098284219050107, 11.00000000000000000 ) ) ;
#3195=CARTESIAN_POINT ( 'NONE',  ( -34.92340065173439712, -3.770459477548423699, 14.53008259254011136 ) ) ;
#3207=CARTESIAN_POINT ( 'NONE',  ( -12.60925743039346969, 20.19802119783879490, 19.66345542862530493 ) ) ;
#3216=CIRCLE ( 'NONE', #25910, 58.00000000000007816 ) ;
#3218=CARTESIAN_POINT ( 'NONE',  ( 8.859192577249610068, 12.20922670554003631, 23.00000000000000000 ) ) ;
#3231=CARTESIAN_POINT ( 'NONE',  ( -4.441848239913464447, 24.85865334748893929, 23.00000000000000000 ) ) ;
#3261=CARTESIAN_POINT ( 'NONE',  ( -1.435176708165770409E-13, 40.16401087634232425, 13.32518128616608699 ) ) ;
#3264=CARTESIAN_POINT ( 'NONE',  ( -1.073573824165845014, 32.41755745572908154, 20.25080042701565830 ) ) ;
#3281=CARTESIAN_POINT ( 'NONE',  ( -32.73577250672335026, -2.961872765701405008, 16.87380292611397081 ) ) ;
#3305=CARTESIAN_POINT ( 'NONE',  ( 32.69618749603090890, -17.08296528845530560, 17.92354375535250810 ) ) ;
#3314=PRODUCT_DEFINITION ( 'UNKNOWN', '', #28786, #48 ) ;
#3317=CARTESIAN_POINT ( 'NONE',  ( 25.26292323896833381, 8.700328014641888430, 13.92931973827844416 ) ) ;
#3328=CARTESIAN_POINT ( 'NONE',  ( -27.24589624691908440, -6.395450141004457301, 20.50957957746007665 ) ) ;
#3353=CARTESIAN_POINT ( 'NONE',  ( 26.96432039561798533, -11.11241571815020279, 20.82122704794079837 ) ) ;
#3386=CARTESIAN_POINT ( 'NONE',  ( -15.03860650580583780, -28.48662463501947428, 12.73282698324853257 ) ) ;
#3396=CARTESIAN_POINT ( 'NONE',  ( -16.89748511972594258, 9.755767582500416424, 19.99202127657103389 ) ) ;
#3403=CARTESIAN_POINT ( 'NONE',  ( 36.80210562958740184, -14.73639196410467100, 13.32518128616608877 ) ) ;
#3412=DIRECTION ( 'NONE',  ( -1.000000000000000000, 0.000000000000000000, 0.000000000000000000 ) ) ;
#3425=CARTESIAN_POINT ( 'NONE',  ( 8.437494165184368455, 40.76200631401353291, 22.99999999999999645 ) ) ;
#3431=AXIS2_PLACEMENT_3D ( 'NONE', #20422, #36457, #11077 ) ;
#3438=CARTESIAN_POINT ( 'NONE',  ( -35.48105285891828231, 0.8254987174888869239, 11.00000000000000355 ) ) ;
#3444=EDGE_CURVE ( 'NONE', #8510, #20949, #25043, .T. ) ;
#3459=CARTESIAN_POINT ( 'NONE',  ( 5.638963013753452991, 39.23975437003361577, 13.32518128616608877 ) ) ;
#3460=DIRECTION ( 'NONE',  ( 1.000000000000000000, 0.000000000000000000, 0.000000000000000000 ) ) ;
#3463=CARTESIAN_POINT ( 'NONE',  ( 12.17657648715484164, 27.34841683166593640, 18.87996532025935892 ) ) ;
#3481=CARTESIAN_POINT ( 'NONE',  ( -35.04992612853192924, -12.66836002548420304, 16.87380292611438648 ) ) ;
#3490=EDGE_LOOP ( 'NONE', ( #23406, #39452, #6688, #13183 ) ) ;
#3499=ORIENTED_EDGE ( 'NONE', *, *, #23517, .F. ) ;
#3505=CARTESIAN_POINT ( 'NONE',  ( 33.89025995733786090, -4.271010277521167353, 16.30093088680190760 ) ) ;
#3509=CARTESIAN_POINT ( 'NONE',  ( -2.109373541296185373, 27.06550157850340810, 20.99999999999999645 ) ) ;
#3525=CARTESIAN_POINT ( 'NONE',  ( -26.67038870798852557, -5.578326634890662383, 20.50957957746030402 ) ) ;
#3551=CARTESIAN_POINT ( 'NONE',  ( 27.53764137321996586, -17.13852093243014352, 20.25080042701566541 ) ) ;
#3553=EDGE_CURVE ( 'NONE', #1139, #29890, #9808, .T. ) ;
#3586=CARTESIAN_POINT ( 'NONE',  ( -32.59722377598335896, -23.23978988006665958, 13.32518128616595909 ) ) ;
#3594=CARTESIAN_POINT ( 'NONE',  ( 18.23649648353767461, -16.09146789626181118, 23.00000000000000000 ) ) ;
#3595=CARTESIAN_POINT ( 'NONE',  ( -9.401525468405969477, 34.87112330957656070, 16.87380292611441845 ) ) ;
#3599=CARTESIAN_POINT ( 'NONE',  ( -25.49469310293981295, 2.228649397504699703, 18.42518152272610266 ) ) ;
#3602=CARTESIAN_POINT ( 'NONE',  ( 23.54266556773325192, -14.22277663958715266, 23.00000000000000355 ) ) ;
#3605=CARTESIAN_POINT ( 'NONE',  ( 26.23899120466339951, -27.34191102820725661, 13.92931973827808356 ) ) ;
#3617=DIRECTION ( 'NONE',  ( 0.000000000000000000, 0.000000000000000000, 1.000000000000000000 ) ) ;
#3625=CARTESIAN_POINT ( 'NONE',  ( -17.76739295965290211, 31.93461338995447107, 11.00000000000000000 ) ) ;
#3657=CARTESIAN_POINT ( 'NONE',  ( -12.20958131808417235, 35.40723086407943754, 13.32518128616661812 ) ) ;
#3659=CARTESIAN_POINT ( 'NONE',  ( -4.817371740575545402, 23.83900317890010001, 23.00000000000000000 ) ) ;
#3660=CARTESIAN_POINT ( 'NONE',  ( 6.761248272851016594, 33.72770196150386823, 18.87996532025785257 ) ) ;
#3678=CARTESIAN_POINT ( 'NONE',  ( -34.35058160602017097, -9.363338975649535101, 17.42190598798392998 ) ) ;
#3702=CARTESIAN_POINT ( 'NONE',  ( 18.91633830555523943, -27.33967421372791406, 16.30093088680201419 ) ) ;
#3705=CARTESIAN_POINT ( 'NONE',  ( -3.833852081710641624, 25.75497152300895820, 20.99999999999999645 ) ) ;
#3710=CARTESIAN_POINT ( 'NONE',  ( 25.66376117785140565, 8.978964872295907895, 12.14047268033175797 ) ) ;
#3719=CARTESIAN_POINT ( 'NONE',  ( -27.41073561697751515, -13.75826678483051424, 20.69868183039780618 ) ) ;
#3744=CARTESIAN_POINT ( 'NONE',  ( 16.60464863832688565, -22.41657912773190375, 19.66345542862528362 ) ) ;
#3782=CARTESIAN_POINT ( 'NONE',  ( -36.34524575547219882, -5.221887369237684595, 12.73282698324894824 ) ) ;
#3790=CARTESIAN_POINT ( 'NONE',  ( 3.366772934462163747, 37.76190412503621729, 16.87380292611444688 ) ) ;
#3795=CARTESIAN_POINT ( 'NONE',  ( -11.83264664767723318, 25.78892025137227151, 19.27171037444156809 ) ) ;
#3803=CARTESIAN_POINT ( 'NONE',  ( 34.83525826321752561, -1.648928274806286565, 11.55979286843933984 ) ) ;
#3836=DIRECTION ( 'NONE',  ( -0.000000000000000000, -0.000000000000000000, -1.000000000000000000 ) ) ;
#3837=CARTESIAN_POINT ( 'NONE',  ( -36.90323640188874066, -1.335463057344152604, 10.99999999999999822 ) ) ;
#3847=CARTESIAN_POINT ( 'NONE',  ( -32.33143948541797386, 1.358872982501903248, 11.00000000000000000 ) ) ;
#3850=B_SPLINE_SURFACE_WITH_KNOTS ( 'NONE', 3, 3, ( 
 ( #8903, #24540, #12344, #36532, #34087, #33503, #30644 ),
 ( #33300, #39575, #11951, #39772, #2609, #36936, #11751 ),
 ( #39971, #5645, #18055, #30447, #2803, #15196, #12150 ),
 ( #27586, #9101, #24732, #24135, #21095, #37132, #21488 ),
 ( #17860, #27188, #23939, #14995, #24340, #36738, #30241 ),
 ( #33893, #6046, #6245, #14600, #21295, #15395, #18450 ),
 ( #33700, #5851, #18253, #30839, #9304, #27788, #40172 ),
 ( #21687, #30038, #2213, #26988, #36337, #39376, #11554 ),
 ( #8500, #2410, #14801, #25329, #6832, #31232, #19234 ),
 ( #34485, #22476, #35081, #6631, #31042, #37925, #28782 ),
 ( #37729, #9706, #10097, #25132, #28376, #18649, #27981 ),
 ( #9503, #556, #13132, #153, #22678, #19041, #31432 ),
 ( #37531, #15790, #25729, #28181, #7036, #34681, #22085 ),
 ( #10297, #3599, #21880, #15594, #13335, #34883, #358 ),
 ( #3993, #15995, #19434, #12938, #16195, #9896, #12545 ),
 ( #22276, #31827, #12737, #6440, #31628, #16394, #3795 ),
 ( #28579, #753, #38123, #25525, #958, #3207, #24936 ),
 ( #37329, #34287, #18845, #3396, #16805, #29385, #17006 ),
 ( #1765, #29189, #7235, #17212, #23088, #35488, #7648 ),
 ( #20253, #29587, #10912, #7846, #14149, #29793, #1357 ),
 ( #1975, #32651, #39129, #22878, #4400, #1159, #38527 ),
 ( #7441, #5005, #38934, #26547, #23696, #32031, #20051 ),
 ( #11109, #1561, #13945, #10702, #26130, #4605, #14352 ),
 ( #17418, #35690, #19635, #26339, #4199, #4807, #32446 ),
 ( #38733, #38327, #23493, #23297, #35283, #20458, #35889 ) ),
 .UNSPECIFIED., .F., .F., .F.,
 ( 4, 3, 3, 3, 3, 3, 3, 3, 4 ),
 ( 4, 3, 4 ),
 ( 0.000000000000000000, 0.1250000000000000000, 0.2500000000000000000, 0.3750000000000000000, 0.5000000000000000000, 0.6250000000000000000, 0.7500000000000000000, 0.8750000000000000000, 1.000000000000000000 ),
 ( 5.507097317918141499, 5.759586531581287971, 6.012075745244433556 ),
 .UNSPECIFIED. ) ;
#3858=CARTESIAN_POINT ( 'NONE',  ( -15.98961535660690636, 30.99268274074326257, 10.99999999999966249 ) ) ;
#3861=CARTESIAN_POINT ( 'NONE',  ( -5.983876423895868157, 32.43697950591384682, 19.66345542862462281 ) ) ;
#3876=ORIENTED_EDGE ( 'NONE', *, *, #6864, .T. ) ;
#3878=CARTESIAN_POINT ( 'NONE',  ( -34.49513285232489324, -12.61775564956212570, 17.42190598798391576 ) ) ;
#3895=CARTESIAN_POINT ( 'NONE',  ( -32.93563651212921428, -26.12966208807736379, 11.00000000000000533 ) ) ;
#3900=CARTESIAN_POINT ( 'NONE',  ( 34.64551053920951063, -5.829853277351126017, 16.30093088680154167 ) ) ;
#3902=CARTESIAN_POINT ( 'NONE',  ( 16.24129362380267239, 27.01431713449539629, 15.13084544680213561 ) ) ;
#3905=CARTESIAN_POINT ( 'NONE',  ( -3.503066876656364403, 27.10955750621961258, 20.99999999999998934 ) ) ;
#3909=AXIS2_PLACEMENT_3D ( 'NONE', #38539, #28793, #10712 ) ;
#3912=CARTESIAN_POINT ( 'NONE',  ( 22.19961376577536072, 12.81695298357553270, 15.13084544680213561 ) ) ;
#3921=CARTESIAN_POINT ( 'NONE',  ( -28.51362642450540719, -10.10416295265245878, 20.50957957746029336 ) ) ;
#3947=CARTESIAN_POINT ( 'NONE',  ( 28.61121519738619767, -15.27903652329876394, 20.25080042701566541 ) ) ;
#3951=CARTESIAN_POINT ( 'NONE',  ( 18.23649648353767461, -16.09146789626181118, 23.00000000000000000 ) ) ;
#3967=VERTEX_POINT ( 'NONE', #30098 ) ;
#3974=FACE_OUTER_BOUND ( 'NONE', #3490, .T. ) ;
#3982=CARTESIAN_POINT ( 'NONE',  ( -34.66558941538325200, -1.755063786819271554, 12.73282698324811513 ) ) ;
#3988=CARTESIAN_POINT ( 'NONE',  ( -19.26948696230207858, 27.85601271560029701, 11.00000000000000000 ) ) ;
#3990=CARTESIAN_POINT ( 'NONE',  ( 14.43694901005322961, 26.51279404187409838, 17.42190598798392642 ) ) ;
#3993=CARTESIAN_POINT ( 'NONE',  ( -28.78471548568728977, -2.122417091760708807, 18.87996532025784902 ) ) ;
#3999=CARTESIAN_POINT ( 'NONE',  ( 18.84787193029120544, -29.28148226148236688, 12.14047268033136007 ) ) ;
#4006=ORIENTED_EDGE ( 'NONE', *, *, #20002, .T. ) ;
#4011=DIRECTION ( 'NONE',  ( 1.000000000000000000, -2.775557561562887801E-15, 0.000000000000000000 ) ) ;
#4049=EDGE_CURVE ( 'NONE', #22892, #39914, #33946, .T. ) ;
#4051=CARTESIAN_POINT ( 'NONE',  ( -9.308285395647398985, 37.95628792398468221, 12.14047268033065485 ) ) ;
#4055=CARTESIAN_POINT ( 'NONE',  ( 7.430899969936454852, 32.27804933232965823, 19.27171037444156454 ) ) ;
#4060=AXIS2_PLACEMENT_3D ( 'NONE', #2761, #6205, #39535 ) ;
#4071=CARTESIAN_POINT ( 'NONE',  ( -2.594149110900493937, 26.80855565015070496, 20.99999999999999289 ) ) ;
#4076=CARTESIAN_POINT ( 'NONE',  ( -32.12208287523078099, -1.273987114064245585, 16.30093088680183300 ) ) ;
#4088=VERTEX_POINT ( 'NONE', #18509 ) ;
#4100=CARTESIAN_POINT ( 'NONE',  ( 22.45589477776615084, -27.55224120904853180, 15.72805884748925465 ) ) ;
#4102=CARTESIAN_POINT ( 'NONE',  ( -15.42165057838474063, 26.78649484830226157, 16.30093088680190405 ) ) ;
#4104=CARTESIAN_POINT ( 'NONE',  ( 5.870938322429559264, 25.61771427147129998, 20.94377226548379056 ) ) ;
#4110=CARTESIAN_POINT ( 'NONE',  ( 27.25314217023234775, 3.686469637062584681, 16.30093088681134006 ) ) ;
#4120=CARTESIAN_POINT ( 'NONE',  ( -31.52520841578658306, -13.67397774227592500, 19.27171037444156099 ) ) ;
#4140=CARTESIAN_POINT ( 'NONE',  ( -24.49409870380020848, -11.70597971641812407, 23.00000000000000000 ) ) ;
#4146=CARTESIAN_POINT ( 'NONE',  ( 23.32346807013517775, -20.39486175172845961, 20.25080042701565830 ) ) ;
#4163=EDGE_CURVE ( 'NONE', #14259, #28327, #11470, .T. ) ;
#4173=CARTESIAN_POINT ( 'NONE',  ( 18.84567888139521230, -29.34375185562581478, 11.00000000000044764 ) ) ;
#4184=CARTESIAN_POINT ( 'NONE',  ( -20.74852905477007781, -28.65583854707632128, 13.92931973827808712 ) ) ;
#4193=CARTESIAN_POINT ( 'NONE',  ( -1.257289260074403992E-13, 36.85721162268941242, 17.92354375535250810 ) ) ;
#4199=CARTESIAN_POINT ( 'NONE',  ( -9.576215452290691488, 12.54651180040780289, 20.99999999999999645 ) ) ;
#4202=CARTESIAN_POINT ( 'NONE',  ( 24.38721429972434152, -12.23686305972968924, 20.99999999999999645 ) ) ;
#4205=CARTESIAN_POINT ( 'NONE',  ( 31.38526299860049917, -24.75545609243360801, 11.55979286843934872 ) ) ;
#4228=CARTESIAN_POINT ( 'NONE',  ( -19.26948696230206792, 27.85601271560034320, 22.99999999999999289 ) ) ;
#4258=CARTESIAN_POINT ( 'NONE',  ( 5.746222359017512993, 39.55816310746057241, 11.00000000000000533 ) ) ;
#4259=CARTESIAN_POINT ( 'NONE',  ( 23.05386822411318803, -7.747535282638377652, 20.99999999999999645 ) ) ;
#4261=CARTESIAN_POINT ( 'NONE',  ( 5.180310612586525920, 33.71427074068280660, 19.27171037444157164 ) ) ;
#4274=CARTESIAN_POINT ( 'NONE',  ( 15.60391421430543701, -26.29546805949240351, 16.87380292611441490 ) ) ;
#4280=CARTESIAN_POINT ( 'NONE',  ( -34.31157940325302746, -4.066883398345795264, 15.72805884748939498 ) ) ;
#4299=CARTESIAN_POINT ( 'NONE',  ( -35.94977730715254438, -22.70593821294886183, 10.99999999999999822 ) ) ;
#4303=CARTESIAN_POINT ( 'NONE',  ( 22.37152845209730501, -27.08896763657755002, 16.30093088680180102 ) ) ;
#4306=CARTESIAN_POINT ( 'NONE',  ( 15.87271491999989159, 26.91186955879558695, 15.72805884748939143 ) ) ;
#4308=CARTESIAN_POINT ( 'NONE',  ( 16.60464863833278670, -22.41657912773326444, 19.66345542862528362 ) ) ;
#4310=CARTESIAN_POINT ( 'NONE',  ( 5.410216727984865415, 24.65457866814638876, 21.00000000000019540 ) ) ;
#4316=CARTESIAN_POINT ( 'NONE',  ( 21.86831431663940961, 12.62567715743453967, 15.72805884748939498 ) ) ;
#4325=CARTESIAN_POINT ( 'NONE',  ( -25.09931006221018635, -21.40067874915750323, 19.66345542862498164 ) ) ;
#4346=CARTESIAN_POINT ( 'NONE',  ( -19.30730118283917562, -16.27608008926387839, 23.00000000000000000 ) ) ;
#4350=CARTESIAN_POINT ( 'NONE',  ( 29.18902924043364422, -8.936254945821255902, 20.25080042701565475 ) ) ;
#4386=CARTESIAN_POINT ( 'NONE',  ( -37.51589702892739098, -12.89337557385636579, 11.55979286843906095 ) ) ;
#4395=CARTESIAN_POINT ( 'NONE',  ( -14.00263291006904964, 28.07534605033868402, 17.42190598798347168 ) ) ;
#4400=CARTESIAN_POINT ( 'NONE',  ( -11.82346474097917621, 13.60361205939885565, 20.69868183039782750 ) ) ;
#4409=CARTESIAN_POINT ( 'NONE',  ( 37.51589702892718492, -12.89337557385771049, 11.55979286843950860 ) ) ;
#4443=CARTESIAN_POINT ( 'NONE',  ( -20.92112759555556067, -16.07000418475134040, 21.00000000000000355 ) ) ;
#4452=CARTESIAN_POINT ( 'NONE',  ( -30.57450045107345815, -0.3656520783135126518, 16.87380292611442201 ) ) ;
#4462=CARTESIAN_POINT ( 'NONE',  ( -13.80290580123969058, 34.21636679304901918, 11.00000000000033573 ) ) ;
#4466=CARTESIAN_POINT ( 'NONE',  ( -9.006936242053182440, 32.02107499576991501, 18.87996532025859864 ) ) ;
#4469=CARTESIAN_POINT ( 'NONE',  ( 0.000000000000000000, 0.000000000000000000, 0.000000000000000000 ) ) ;
#4486=CARTESIAN_POINT ( 'NONE',  ( -33.75286824399729824, -19.48722756659376998, 15.72805884748939853 ) ) ;
#4504=CARTESIAN_POINT ( 'NONE',  ( -15.96050091527624559, -30.99544168074540806, 11.00000000000000178 ) ) ;
#4508=CARTESIAN_POINT ( 'NONE',  ( 24.32690616642214465, -27.49953951067901414, 15.13084544680245713 ) ) ;
#4509=EDGE_CURVE ( 'NONE', #16240, #10384, #34157, .T. ) ;
#4511=CARTESIAN_POINT ( 'NONE',  ( -1.732136883777231740, 38.50629078351121137, 16.30093088680190050 ) ) ;
#4513=CARTESIAN_POINT ( 'NONE',  ( 4.327222458066418466E-14, -22.50706359516090060, 18.42518152272108978 ) ) ;
#4515=CARTESIAN_POINT ( 'NONE',  ( 2.374005179830479761, 29.54744178790033260, 20.82122704794079837 ) ) ;
#4520=AXIS2_PLACEMENT_3D ( 'NONE', #37548, #37145, #3412 ) ;
#4523=CARTESIAN_POINT ( 'NONE',  ( 29.28423149095877775, -1.632116715646416472, 18.42518152272108978 ) ) ;
#4530=CARTESIAN_POINT ( 'NONE',  ( -17.92913371968332825, -21.93458435334723333, 19.99202127657105876 ) ) ;
#4550=CARTESIAN_POINT ( 'NONE',  ( -39.05366788732968786, -6.582903524762039993, 22.99999999999811351 ) ) ;
#4555=CARTESIAN_POINT ( 'NONE',  ( 30.12142568021469557, -17.39061322484706196, 19.27171037444156454 ) ) ;
#4592=CARTESIAN_POINT ( 'NONE',  ( -37.34232268491270190, -8.983628415038371173, 11.55979286843934872 ) ) ;
#4605=CARTESIAN_POINT ( 'NONE',  ( -7.976544127345993829, 18.48053530966456037, 20.94377226548371596 ) ) ;
#4613=CARTESIAN_POINT ( 'NONE',  ( 37.14493776307928385, -9.008680429015726077, 12.73282698324853435 ) ) ;
#4624=CARTESIAN_POINT ( 'NONE',  ( 27.36225479889086287, 10.16098284204021240, 10.99999999999999645 ) ) ;
#4649=ORIENTED_EDGE ( 'NONE', *, *, #5889, .T. ) ;
#4654=B_SPLINE_CURVE_WITH_KNOTS ( 'NONE', 3,
 ( #25403, #31705, #28455, #7313, #26005, #1034, #38402, #9973, #25210, #22351, #34757, #16679, #4071, #6908, #37611, #7113, #7517, #22157 ),
 .UNSPECIFIED., .F., .F.,
 ( 4, 2, 2, 2, 2, 2, 2, 2, 4 ),
 ( 0.000000000000000000, 0.1249999999999999445, 0.2499999999999999445, 0.3749999999999999445, 0.4999999999999998890, 0.6249999999999997780, 0.7499999999999998890, 0.8749999999999998890, 1.000000000000000000 ),
 .UNSPECIFIED. ) ;
#4666=CARTESIAN_POINT ( 'NONE',  ( -13.22866120779009336, 26.17694675929174153, 18.42518152272108622 ) ) ;
#4672=CARTESIAN_POINT ( 'NONE',  ( -32.33143948541797386, 1.358872982501903248, 11.00000000000000000 ) ) ;
#4681=ADVANCED_FACE ( 'NONE', ( #28192 ), #29142, .T. ) ;
#4683=EDGE_CURVE ( 'NONE', #4972, #12781, #2712, .T. ) ;
#4686=CARTESIAN_POINT ( 'NONE',  ( -30.37673449013114890, -23.61083502489086428, 15.72805884748940031 ) ) ;
#4711=CARTESIAN_POINT ( 'NONE',  ( 33.75286824399746166, -19.48722756659364919, 15.72805884748939498 ) ) ;
#4714=CARTESIAN_POINT ( 'NONE',  ( -9.968062119478286576, 35.61660815598440166, 15.72805884748939853 ) ) ;
#4715=CARTESIAN_POINT ( 'NONE',  ( -10.93513760491349274, -22.50092802249447033, 18.87996532025975327 ) ) ;
#4717=CARTESIAN_POINT ( 'NONE',  ( -6.606256860318982405, 26.00827479057969072, 20.82122704794080548 ) ) ;
#4724=CARTESIAN_POINT ( 'NONE',  ( 21.05742987670727118, 12.15751280775815424, 16.87380292611441490 ) ) ;
#4733=CARTESIAN_POINT ( 'NONE',  ( -29.86387254395543778, -6.221772116353116111, 19.66345542862528717 ) ) ;
#4739=EDGE_LOOP ( 'NONE', ( #2342, #7493, #38067, #10112 ) ) ;
#4748=CARTESIAN_POINT ( 'NONE',  ( 38.66460482714355607, -17.32098561216399446, 22.99999999999999645 ) ) ;
#4759=CARTESIAN_POINT ( 'NONE',  ( 28.09977684436853806, -21.02662082632513574, 18.87996532025785967 ) ) ;
#4781=CARTESIAN_POINT ( 'NONE',  ( -24.96922908923108508, -9.289876063515562166, 21.00000000000004619 ) ) ;
#4792=CARTESIAN_POINT ( 'NONE',  ( -37.09709568333396845, -7.051483854460184553, 10.99999999999968026 ) ) ;
#4797=ADVANCED_FACE ( 'NONE', ( #21500 ), #18462, .F. ) ;
#4807=CARTESIAN_POINT ( 'NONE',  ( -7.205739717619530360, 18.19477196585663137, 20.99999999999999645 ) ) ;
#4808=CARTESIAN_POINT ( 'NONE',  ( 23.43324262027548599, -8.134040356058102716, 20.99999999999999645 ) ) ;
#4812=CARTESIAN_POINT ( 'NONE',  ( 35.68447701591248489, -3.401722300707758162, 11.00000000000000000 ) ) ;
#4862=CARTESIAN_POINT ( 'NONE',  ( -9.991731067009840928, 30.98181186424739408, 18.87996532025781704 ) ) ;
#4874=B_SPLINE_CURVE_WITH_KNOTS ( 'NONE', 3,
 ( #26550, #20054, #20460, #11111, #19143, #31141, #22377, #28483, #37637, #9406, #2907, #28286, #27686, #21786, #31535, #16098, #37036, #12448 ),
 .UNSPECIFIED., .F., .F.,
 ( 4, 2, 2, 2, 2, 2, 2, 2, 4 ),
 ( 0.000000000000000000, 0.1250000000000000000, 0.2500000000000000000, 0.3750000000000000000, 0.5000000000000000000, 0.6250000000000000000, 0.7500000000000000000, 0.8750000000000000000, 1.000000000000000000 ),
 .UNSPECIFIED. ) ;
#4876=CARTESIAN_POINT ( 'NONE',  ( 16.05557028316289703, -24.54483004364954368, 18.42518152272108978 ) ) ;
#4877=B_SPLINE_CURVE_WITH_KNOTS ( 'NONE', 3,
 ( #23107, #25747, #25545, #4624, #19653, #35506 ),
 .UNSPECIFIED., .F., .F.,
 ( 4, 2, 4 ),
 ( 0.000000000000000000, 0.5000000000000000000, 1.000000000000000000 ),
 .UNSPECIFIED. ) ;
#4883=CARTESIAN_POINT ( 'NONE',  ( -34.59909889755191159, -19.97579906222007295, 13.92931973827808534 ) ) ;
#4885=ADVANCED_FACE ( 'NONE', ( #23306 ), #34894, .T. ) ;
#4909=CARTESIAN_POINT ( 'NONE',  ( 18.88617201209933683, -28.19481557848324726, 15.13084544680231502 ) ) ;
#4911=CARTESIAN_POINT ( 'NONE',  ( -1.888379873391735186, 39.95159812444025249, 13.92931973827808534 ) ) ;
#4913=CARTESIAN_POINT ( 'NONE',  ( 16.05557028316878387, -24.54483004365089371, 18.42518152272108978 ) ) ;
#4917=CARTESIAN_POINT ( 'NONE',  ( 0.9851783940329167377, 31.60047892813805248, 20.50957957746028626 ) ) ;
#4926=CARTESIAN_POINT ( 'NONE',  ( 6.462764152049920163, 17.91932574229958419, 20.99999999999999645 ) ) ;
#4937=CARTESIAN_POINT ( 'NONE',  ( -20.32014898129551739, -22.75198622026924511, 19.66345542862528717 ) ) ;
#4948=ORIENTED_EDGE ( 'NONE', *, *, #9412, .F. ) ;
#4956=CARTESIAN_POINT ( 'NONE',  ( -14.48927117870124093, -30.61587158504648443, 22.99999999999999289 ) ) ;
#4962=CARTESIAN_POINT ( 'NONE',  ( 32.23453252384990719, -8.210301902000198382, 18.87996532025784191 ) ) ;
#4972=VERTEX_POINT ( 'NONE', #30756 ) ;
#4994=CARTESIAN_POINT ( 'NONE',  ( -28.24711154207075481, -27.09388640670391979, 11.00000000000006573 ) ) ;
#5005=CARTESIAN_POINT ( 'NONE',  ( -20.63240589125325641, -1.802217369530700442, 20.82122704794238999 ) ) ;
#5006=CARTESIAN_POINT ( 'NONE',  ( 25.16128423893353627, -12.39270898182871328, 20.99999999999999645 ) ) ;
#5009=CARTESIAN_POINT ( 'NONE',  ( 32.33143948541781043, 1.358872982501757143, 11.55979286843934872 ) ) ;
#5059=ORIENTED_EDGE ( 'NONE', *, *, #5820, .F. ) ;
#5061=ORIENTED_EDGE ( 'NONE', *, *, #5889, .F. ) ;
#5075=CARTESIAN_POINT ( 'NONE',  ( -3.831203748877743731, 25.75875950449070118, 23.00000000000000000 ) ) ;
#5086=CARTESIAN_POINT ( 'NONE',  ( -35.19094867589920028, -3.640833979052929603, 13.92931973827808889 ) ) ;
#5103=CARTESIAN_POINT ( 'NONE',  ( -24.45973306916671319, -28.60230771035024233, 10.99999999999987033 ) ) ;
#5111=CARTESIAN_POINT ( 'NONE',  ( 35.98781724630865142, -12.75392035872628860, 15.72805884748942873 ) ) ;
#5113=CARTESIAN_POINT ( 'NONE',  ( -5.381339405376368568, 38.47497618056175384, 15.13084544680213561 ) ) ;
#5114=CARTESIAN_POINT ( 'NONE',  ( 5.304193131309242304, -23.76115801358234947, 17.42190598798392998 ) ) ;
#5117=CARTESIAN_POINT ( 'NONE',  ( -6.949287954459967942, 25.26733242291857451, 20.82122704794066692 ) ) ;
#5126=CARTESIAN_POINT ( 'NONE',  ( 11.11100267139158859, 25.58833710558854690, 19.66345542862528362 ) ) ;
#5136=CARTESIAN_POINT ( 'NONE',  ( -19.04855072600353338, -23.59522350949000469, 19.27171037444189139 ) ) ;
#5150=CARTESIAN_POINT ( 'NONE',  ( 18.23649648353767461, -16.09146789626181118, 23.00000000000000000 ) ) ;
#5159=CARTESIAN_POINT ( 'NONE',  ( 28.78471548569268279, -2.122417091766370945, 18.87996532025785257 ) ) ;
#5175=DIRECTION ( 'NONE',  ( -0.000000000000000000, -0.000000000000000000, -1.000000000000000000 ) ) ;
#5180=CARTESIAN_POINT ( 'NONE',  ( -10.10865978838755908, -27.35622988135655476, 12.14047268034456017 ) ) ;
#5184=CARTESIAN_POINT ( 'NONE',  ( -19.96384346486619066, -17.84145166816490047, 20.94377226548378346 ) ) ;
#5195=CARTESIAN_POINT ( 'NONE',  ( -37.34232268491268769, -8.983628415038266368, 11.00000000000000000 ) ) ;
#5210=CARTESIAN_POINT ( 'NONE',  ( 20.67756474496276908, -17.78966446931796952, 20.94377226548379056 ) ) ;
#5214=CARTESIAN_POINT ( 'NONE',  ( 33.69589222704783538, -0.03122585499640089662, 11.00000000000003730 ) ) ;
#5241=CARTESIAN_POINT ( 'NONE',  ( 23.09341954621653414, -31.04079623342705574, 11.00000000000000000 ) ) ;
#5252=ORIENTED_EDGE ( 'NONE', *, *, #25945, .T. ) ;
#5280=CARTESIAN_POINT ( 'NONE',  ( 17.83459896181130944, -17.64923967996766052, 20.94377226548378701 ) ) ;
#5284=CARTESIAN_POINT ( 'NONE',  ( -34.99622266290882777, -18.09877784578709026, 15.13084544680241272 ) ) ;
#5308=CARTESIAN_POINT ( 'NONE',  ( 26.00889624226716990, -26.79364542773732083, 15.13084544680213384 ) ) ;
#5310=CARTESIAN_POINT ( 'NONE',  ( 13.38235399890562682, 33.85943911868815093, 13.92931973827816883 ) ) ;
#5313=CARTESIAN_POINT ( 'NONE',  ( -4.288075229729694016, 29.62123851723948675, 20.69868183039744025 ) ) ;
#5315=EDGE_LOOP ( 'NONE', ( #39821, #10489, #17426, #25936 ) ) ;
#5322=CARTESIAN_POINT ( 'NONE',  ( 21.27192666511442098, -1.272056932922072114, 20.69868183040414422 ) ) ;
#5325=CARTESIAN_POINT ( 'NONE',  ( 15.98959510862178668, 30.99271259066394180, 10.99999999999987743 ) ) ;
#5333=CARTESIAN_POINT ( 'NONE',  ( -30.32526513704001303, -2.692717509695762512, 18.42518152272108622 ) ) ;
#5348=CARTESIAN_POINT ( 'NONE',  ( 23.54493052986452284, -14.21898406159493788, 23.00000000000000000 ) ) ;
#5352=CARTESIAN_POINT ( 'NONE',  ( -38.42882785865669604, -4.479089857567689847, 11.00000000000000000 ) ) ;
#5357=CARTESIAN_POINT ( 'NONE',  ( 17.49459433713328593, -24.91609123032452899, 18.42518152272071674 ) ) ;
#5364=CARTESIAN_POINT ( 'NONE',  ( -17.21213525677265821, -20.06193531423681975, 20.50957957746029692 ) ) ;
#5378=CARTESIAN_POINT ( 'NONE',  ( 10.29072928255106234, -26.28675887227032248, 15.13084544680038235 ) ) ;
#5381=CARTESIAN_POINT ( 'NONE',  ( -24.79273775960151482, -6.040746354374424421, 20.82122704794080192 ) ) ;
#5396=CARTESIAN_POINT ( 'NONE',  ( -24.49409870380021204, -11.70597971641812407, 20.99999999999999645 ) ) ;
#5410=CARTESIAN_POINT ( 'NONE',  ( 25.12105899710777024, -7.724472287617720312, 20.94377226548389004 ) ) ;
#5413=CARTESIAN_POINT ( 'NONE',  ( 20.78821643698968913, -29.20280246618838049, 11.00000000000000000 ) ) ;
#5442=CARTESIAN_POINT ( 'NONE',  ( 39.59914439537040209, -10.88071518964973805, 11.00000000000000178 ) ) ;
#5469=CARTESIAN_POINT ( 'NONE',  ( -1.078765555139302945, 27.41260393370252402, 23.00000000000000000 ) ) ;
#5475=CARTESIAN_POINT ( 'NONE',  ( 13.82587226056095986, 37.11292026376941777, 23.00000000000000000 ) ) ;
#5485=ORIENTED_EDGE ( 'NONE', *, *, #29461, .F. ) ;
#5501=CARTESIAN_POINT ( 'NONE',  ( 24.49773858737317767, -28.07267629079924731, 13.92931973827831627 ) ) ;
#5503=CARTESIAN_POINT ( 'NONE',  ( -3.781581747449368258, 39.64129210796443914, 13.92931973827819903 ) ) ;
#5506=CARTESIAN_POINT ( 'NONE',  ( -4.721973484739690363, 30.34170004520404262, 20.50957957745984217 ) ) ;
#5516=CARTESIAN_POINT ( 'NONE',  ( 13.32438941869560800, 7.692839817671511149, 20.94377226548378346 ) ) ;
#5529=CARTESIAN_POINT ( 'NONE',  ( -16.41753675003402790, -23.14183271658250973, 19.27171037444156454 ) ) ;
#5539=ORIENTED_EDGE ( 'NONE', *, *, #22163, .T. ) ;
#5542=CARTESIAN_POINT ( 'NONE',  ( 31.08218589456564018, -27.68808744834087321, 22.99999999999905853 ) ) ;
#5553=CARTESIAN_POINT ( 'NONE',  ( 34.49513285232596616, -12.61775564956195872, 17.42190598798392642 ) ) ;
#5556=AXIS2_PLACEMENT_3D ( 'NONE', #22014, #31953, #10023 ) ;
#5561=CARTESIAN_POINT ( 'NONE',  ( -16.80389827882203235, -21.64427909825945662, 19.99202127657104100 ) ) ;
#5573=CARTESIAN_POINT ( 'NONE',  ( 15.07283634910031189, -28.35394831540551763, 13.32518128616608877 ) ) ;
#5576=CARTESIAN_POINT ( 'NONE',  ( -25.74508372771330755, -9.012464122874943584, 20.94377226548387938 ) ) ;
#5598=CYLINDRICAL_SURFACE ( 'NONE', #18614, 59.99999999999995737 ) ;
#5605=CARTESIAN_POINT ( 'NONE',  ( 23.05386822411317027, -7.747535282638454035, 20.99999999999999645 ) ) ;
#5645=CARTESIAN_POINT ( 'NONE',  ( -28.74551992321994831, 4.923758765708712737, 12.14047268033756666 ) ) ;
#5647=FACE_OUTER_BOUND ( 'NONE', #8545, .T. ) ;
#5704=CARTESIAN_POINT ( 'NONE',  ( 15.03860650580494074, -28.48662463501965192, 12.73282698324853257 ) ) ;
#5706=CARTESIAN_POINT ( 'NONE',  ( -8.747212233150712279, 37.02488667718797899, 15.13084544680138954 ) ) ;
#5710=CARTESIAN_POINT ( 'NONE',  ( 8.883663045967715277, 28.52602195317101064, 19.99202127657103745 ) ) ;
#5719=CARTESIAN_POINT ( 'NONE',  ( 7.976544127178703647, 18.48053530960098811, 20.94377226548381898 ) ) ;
#5730=CARTESIAN_POINT ( 'NONE',  ( -16.05557028316514945, -24.54483004364971777, 18.42518152272108622 ) ) ;
#5750=CARTESIAN_POINT ( 'NONE',  ( -31.08218589456761549, -27.68808744834008451, 23.00000000000000000 ) ) ;
#5756=CARTESIAN_POINT ( 'NONE',  ( 22.07432851697283382, -25.45711773545401613, 17.92354375535248323 ) ) ;
#5761=CARTESIAN_POINT ( 'NONE',  ( 1.596172877504872689, 27.23837864096129735, 21.00000000000000355 ) ) ;
#5774=CARTESIAN_POINT ( 'NONE',  ( -6.462764152204139023, 17.91932574235843134, 20.99999999999999289 ) ) ;
#5778=CARTESIAN_POINT ( 'NONE',  ( -15.12590024502445374, -28.14827041158513055, 13.92931973827808889 ) ) ;
#5781=CARTESIAN_POINT ( 'NONE',  ( -27.79678266235375617, -11.09703717633735742, 20.69868183039817211 ) ) ;
#5790=CARTESIAN_POINT ( 'NONE',  ( -20.57674455326939267, 23.15285302515659893, 11.00000000000000000 ) ) ;
#5801=CARTESIAN_POINT ( 'NONE',  ( 15.01946716906679136, 1.539419383720357137, 23.00000000000000355 ) ) ;
#5809=CARTESIAN_POINT ( 'NONE',  ( 22.68370119258272766, -18.87043823706619250, 20.69868183039780263 ) ) ;
#5820=EDGE_CURVE ( 'NONE', #17915, #20949, #16274, .T. ) ;
#5827=CARTESIAN_POINT ( 'NONE',  ( -14.48927117870118408, -30.61587158504671180, 11.00000000000000000 ) ) ;
#5847=ORIENTED_EDGE ( 'NONE', *, *, #39443, .T. ) ;
#5851=CARTESIAN_POINT ( 'NONE',  ( -28.14004025859599878, 4.421764093230089010, 14.53008259254716705 ) ) ;
#5852=ORIENTED_EDGE ( 'NONE', *, *, #31991, .F. ) ;
#5884=CARTESIAN_POINT ( 'NONE',  ( -39.48557158258395816, -9.956519981528337837, 11.00000000000000178 ) ) ;
#5889=EDGE_CURVE ( 'NONE', #24176, #25190, #11467, .T. ) ;
#5905=CARTESIAN_POINT ( 'NONE',  ( 14.73160032165944777, 32.49283138996950981, 12.73282698324854145 ) ) ;
#5907=CARTESIAN_POINT ( 'NONE',  ( 12.28720923547795429, -14.55658080553756406, 20.99999999999999645 ) ) ;
#5909=CARTESIAN_POINT ( 'NONE',  ( 6.000734348600325063, 30.39614672895685032, 20.25080042701566896 ) ) ;
#5927=CARTESIAN_POINT ( 'NONE',  ( -28.09977684436795187, -21.02662082632541285, 18.87996532025785257 ) ) ;
#5952=CARTESIAN_POINT ( 'NONE',  ( 32.40618899211592918, -4.990034233201372516, 17.92354375535250810 ) ) ;
#5957=CARTESIAN_POINT ( 'NONE',  ( -35.70677476034837383, -3.361263978139850117, 11.00000000000007994 ) ) ;
#5961=CARTESIAN_POINT ( 'NONE',  ( 17.34253826607180216, 27.32041144404034227, 11.00000000000000000 ) ) ;
#5973=CARTESIAN_POINT ( 'NONE',  ( -26.86294352747613345, -10.31366695439962911, 20.82122704794079837 ) ) ;
#5999=CARTESIAN_POINT ( 'NONE',  ( 20.14416558653905298, -20.32661669692072692, 20.50957957746028626 ) ) ;
#6006=CIRCLE ( 'NONE', #4060, 20.00000000000002842 ) ;
#6018=CARTESIAN_POINT ( 'NONE',  ( -9.762440214479841671, -29.39637225272702281, 11.00000000000000000 ) ) ;
#6035=CARTESIAN_POINT ( 'NONE',  ( -36.79828514077309620, -9.052677438811558730, 13.92931973827808712 ) ) ;
#6046=CARTESIAN_POINT ( 'NONE',  ( -28.36971490935763640, 4.612181732483940699, 13.92931973828524406 ) ) ;
#6059=CARTESIAN_POINT ( 'NONE',  ( 4.817371740575477013, 23.83900317890016751, 23.00000000000000000 ) ) ;
#6073=CARTESIAN_POINT ( 'NONE',  ( 2.594149110900750177, 26.80855565015185249, 23.00000000000000000 ) ) ;
#6098=CARTESIAN_POINT ( 'NONE',  ( 14.98890121934609532, -28.67928442654220333, 23.00000000000000000 ) ) ;
#6102=CARTESIAN_POINT ( 'NONE',  ( 10.68781676061647978, 36.56370694841956492, 13.32518128616609054 ) ) ;
#6103=CARTESIAN_POINT ( 'NONE',  ( 4.336808689942017736E-14, -13.77689918168226235, 20.99999999999999645 ) ) ;
#6105=CARTESIAN_POINT ( 'NONE',  ( -10.34254640628272348, 25.37474234119852667, 19.99202127657103389 ) ) ;
#6115=EDGE_CURVE ( 'NONE', #16240, #30744, #35148, .T. ) ;
#6125=CARTESIAN_POINT ( 'NONE',  ( -32.10122455788158646, -20.47530094824154645, 16.87380292611404897 ) ) ;
#6138=CARTESIAN_POINT ( 'NONE',  ( 25.22779562677136767, -30.53001673900894630, 11.00000000000000000 ) ) ;
#6151=CARTESIAN_POINT ( 'NONE',  ( 17.31264644460116031, -26.16430884515622424, 17.42190598798342194 ) ) ;
#6165=CARTESIAN_POINT ( 'NONE',  ( 18.50792845150514765, 22.38468038560473872, 12.73282698322912410 ) ) ;
#6175=CARTESIAN_POINT ( 'NONE',  ( -27.31543141964105104, -5.069059863655038356, 20.25080042701567606 ) ) ;
#6196=ORIENTED_EDGE ( 'NONE', *, *, #36702, .T. ) ;
#6202=CARTESIAN_POINT ( 'NONE',  ( -14.48927117870122316, -30.61587158504648087, 11.00000000000000000 ) ) ;
#6203=CARTESIAN_POINT ( 'NONE',  ( 19.19128484611995944, -19.55740768895475767, 20.69868183039780618 ) ) ;
#6205=DIRECTION ( 'NONE',  ( 0.000000000000000000, 0.000000000000000000, 1.000000000000000000 ) ) ;
#6231=CARTESIAN_POINT ( 'NONE',  ( 27.71565130972689772, -3.171757977843684628, 19.66345542862528717 ) ) ;
#6236=CARTESIAN_POINT ( 'NONE',  ( -34.34163329534256803, -19.82715122747743308, 14.53008259254010959 ) ) ;
#6245=CARTESIAN_POINT ( 'NONE',  ( -25.26292323897049030, 8.700328014641360852, 13.92931973827939096 ) ) ;
#6252=B_SPLINE_CURVE_WITH_KNOTS ( 'NONE', 3,
 ( #27422, #5884, #18289, #6873, #25768, #10336, #3837, #3438, #37967, #6674 ),
 .UNSPECIFIED., .F., .F.,
 ( 4, 2, 2, 2, 4 ),
 ( 0.7014326804499604329, 0.7760745103374703247, 0.8507163402249802164, 0.9253581701124901082, 1.000000000000000000 ),
 .UNSPECIFIED. ) ;
#6258=ADVANCED_FACE ( 'NONE', ( #11769 ), #11376, .T. ) ;
#6259=LINE ( 'NONE', #6645, #7377 ) ;
#6297=CARTESIAN_POINT ( 'NONE',  ( 14.84499459426748835, 32.56974970312070639, 12.14047268033098348 ) ) ;
#6301=CARTESIAN_POINT ( 'NONE',  ( 3.426866961292364788, 32.67295397237175081, 19.99202127657103034 ) ) ;
#6308=DIRECTION ( 'NONE',  ( 0.000000000000000000, 0.000000000000000000, 1.000000000000000000 ) ) ;
#6319=CARTESIAN_POINT ( 'NONE',  ( -22.18736851772318275, -26.07761132199846443, 17.42190598798353562 ) ) ;
#6337=VERTEX_POINT ( 'NONE', #36756 ) ;
#6345=CARTESIAN_POINT ( 'NONE',  ( 31.84188463419212312, -5.263436490337560336, 18.42518152272108978 ) ) ;
#6368=CARTESIAN_POINT ( 'NONE',  ( -27.36681752352253127, -15.80023946406859636, 20.50957957746028626 ) ) ;
#6369=DIRECTION ( 'NONE',  ( -0.000000000000000000, -0.000000000000000000, -1.000000000000000000 ) ) ;
#6395=CARTESIAN_POINT ( 'NONE',  ( 24.27776115474282648, -18.04224162735242842, 20.69868183039762854 ) ) ;
#6431=CARTESIAN_POINT ( 'NONE',  ( -16.90387162101869478, -28.96785393638790396, 12.73282698324800499 ) ) ;
#6440=CARTESIAN_POINT ( 'NONE',  ( -18.23687175285704853, 10.52906281568731472, 19.27171037444156454 ) ) ;
#6447=CARTESIAN_POINT ( 'NONE',  ( 36.59387134601873726, -14.69446750445110794, 13.92931973827808712 ) ) ;
#6466=CARTESIAN_POINT ( 'NONE',  ( -13.82587226055908758, 37.11292026377122255, 11.00000000000000000 ) ) ;
#6495=CARTESIAN_POINT ( 'NONE',  ( -3.887054626305479932, 40.11907545043342083, 12.14047268033113802 ) ) ;
#6499=CARTESIAN_POINT ( 'NONE',  ( -8.489237591500351954, 31.47375793095005037, 19.27171037444226798 ) ) ;
#6516=CARTESIAN_POINT ( 'NONE',  ( -32.69618749603004915, -17.08296528845537665, 17.92354375535288469 ) ) ;
#6541=CARTESIAN_POINT ( 'NONE',  ( 34.71804043165853670, -14.31680059899166757, 16.87380292611441845 ) ) ;
#6546=DIRECTION ( 'NONE',  ( -0.000000000000000000, -0.000000000000000000, -1.000000000000000000 ) ) ;
#6547=CARTESIAN_POINT ( 'NONE',  ( 2.109373541296156063, 27.06550157850343652, 21.00000000000000355 ) ) ;
#6558=EDGE_CURVE ( 'NONE', #17265, #4972, #17662, .T. ) ;
#6562=CARTESIAN_POINT ( 'NONE',  ( -29.18902924043318237, -8.936254945823375095, 20.25080042701515737 ) ) ;
#6588=CARTESIAN_POINT ( 'NONE',  ( 29.65273330788082262, -7.615246293903670249, 19.99202127657073902 ) ) ;
#6620=CARTESIAN_POINT ( 'NONE',  ( -32.18944385490189575, 1.219497045964027748, 12.73282698324853079 ) ) ;
#6627=CARTESIAN_POINT ( 'NONE',  ( -6.176557290856002247, -13.77694981160526844, 23.00000000000000355 ) ) ;
#6628=CARTESIAN_POINT ( 'NONE',  ( 3.246717519899792403, 37.21789761807038133, 17.42190598798394774 ) ) ;
#6631=CARTESIAN_POINT ( 'NONE',  ( -21.46287209667396922, 12.39159498259534686, 16.30093088680190405 ) ) ;
#6641=CARTESIAN_POINT ( 'NONE',  ( 33.82738586796132552, -21.73727074213809729, 13.32518128616604791 ) ) ;
#6643=VECTOR ( 'NONE', #18502, 1000.000000000000000 ) ;
#6645=CARTESIAN_POINT ( 'NONE',  ( -14.98890121934603314, -28.67928442654204346, 23.00000000000000000 ) ) ;
#6646=CARTESIAN_POINT ( 'NONE',  ( 23.05386822411319159, -7.747535282638377652, 23.00000000000000000 ) ) ;
#6660=CARTESIAN_POINT ( 'NONE',  ( 8.437494165185171369, 40.76200631401452767, 11.00000000000000000 ) ) ;
#6674=CARTESIAN_POINT ( 'NONE',  ( -33.75875814100324845, 2.759858869446484064, 11.00000000000000000 ) ) ;
#6688=ORIENTED_EDGE ( 'NONE', *, *, #16721, .F. ) ;
#6692=CARTESIAN_POINT ( 'NONE',  ( 9.308285395644954718, 37.95628792398655094, 12.14047268033102256 ) ) ;
#6694=CARTESIAN_POINT ( 'NONE',  ( -23.05386822411323422, -7.747535282638357224, 23.00000000000000000 ) ) ;
#6695=CARTESIAN_POINT ( 'NONE',  ( -1.329271672591240128, 34.78122644969442945, 19.27171037444156454 ) ) ;
#6713=CARTESIAN_POINT ( 'NONE',  ( -23.78889779961598450, -25.69434382178283371, 17.42190598798429590 ) ) ;
#6737=CARTESIAN_POINT ( 'NONE',  ( 31.01938180032263048, -21.79666295253546338, 16.87380292611479859 ) ) ;
#6741=CARTESIAN_POINT ( 'NONE',  ( -4.441848239913461782, 24.85865334748894284, 20.99999999999999645 ) ) ;
#6750=CARTESIAN_POINT ( 'NONE',  ( 23.18947492591164661, 13.38844959084105568, 11.55979286843934872 ) ) ;
#6758=CARTESIAN_POINT ( 'NONE',  ( -23.32346807013534828, -20.39486175172809013, 20.25080042701566541 ) ) ;
#6784=CARTESIAN_POINT ( 'NONE',  ( 29.77970073067787027, -14.50783476829474594, 19.99202127657104811 ) ) ;
#6808=CARTESIAN_POINT ( 'NONE',  ( 37.58754968649119377, -10.91577297561529036, 10.99999999999992717 ) ) ;
#6820=CARTESIAN_POINT ( 'NONE',  ( -32.28722999652134007, 1.315479119631538074, 12.14047268033097282 ) ) ;
#6829=CARTESIAN_POINT ( 'NONE',  ( 1.621626408465995040, 37.48425883190013508, 17.42190598798392642 ) ) ;
#6832=CARTESIAN_POINT ( 'NONE',  ( -19.27886458632313094, 17.11073565397887819, 15.72805884748862404 ) ) ;
#6839=CARTESIAN_POINT ( 'NONE',  ( 29.80853493429485468, -25.87953118561181753, 12.73282698324837092 ) ) ;
#6844=CARTESIAN_POINT ( 'NONE',  ( 18.74997338758756271, -3.362744936767421589, 23.00000000000000000 ) ) ;
#6860=CARTESIAN_POINT ( 'NONE',  ( -4.331888854854716975, 42.14502281367647640, 23.00000000000000000 ) ) ;
#6864=EDGE_CURVE ( 'NONE', #16240, #18297, #15654, .T. ) ;
#6873=CARTESIAN_POINT ( 'NONE',  ( -38.86091370594022010, -6.124650435543221860, 11.00000000000000000 ) ) ;
#6892=CARTESIAN_POINT ( 'NONE',  ( -12.44178368932711543, 35.65276919562048619, 11.55979286843954057 ) ) ;
#6895=CARTESIAN_POINT ( 'NONE',  ( -10.16357496796715054, 29.39421982382238596, 19.27171037444156454 ) ) ;
#6908=CARTESIAN_POINT ( 'NONE',  ( -3.456468065140303025, 26.15323006594351440, 21.00000000000000000 ) ) ;
#6914=CARTESIAN_POINT ( 'NONE',  ( -31.75251099004362132, -1.565804367082550996, 16.87380292611436872 ) ) ;
#6930=CARTESIAN_POINT ( 'NONE',  ( -25.01235460169770519, -30.53116334361912365, 10.99999999999999822 ) ) ;
#6936=CARTESIAN_POINT ( 'NONE',  ( 35.58257249438514691, -10.95300747732849977, 16.30093088680188629 ) ) ;
#6939=CARTESIAN_POINT ( 'NONE',  ( -13.63376536442988396, 31.74814110635680464, 15.72805884748939143 ) ) ;
#6942=CARTESIAN_POINT ( 'NONE',  ( -2.787905735463278134, 28.53453732066314430, 20.94377226548378701 ) ) ;
#6946=CARTESIAN_POINT ( 'NONE',  ( 28.78471548569376282, -2.122417091767359931, 18.87996532025784546 ) ) ;
#6954=CARTESIAN_POINT ( 'NONE',  ( -26.19533169775672476, -16.15700992729037466, 20.69868183039762144 ) ) ;
#6976=CARTESIAN_POINT ( 'NONE',  ( -23.43324262027536875, -8.134040356058614307, 23.00000000000000000 ) ) ;
#6981=CARTESIAN_POINT ( 'NONE',  ( 17.81343984362198540, -22.72844136247426761, 19.66345542862503137 ) ) ;
#7010=CARTESIAN_POINT ( 'NONE',  ( 32.33143948541787438, 1.358872982501792226, 2.999999999999999112 ) ) ;
#7021=CARTESIAN_POINT ( 'NONE',  ( -37.52525227335131319, -10.91693234368756649, 12.14047268033150573 ) ) ;
#7031=CARTESIAN_POINT ( 'NONE',  ( -11.00933375873403541, 31.84550678200677609, 17.92354375535249389 ) ) ;
#7036=CARTESIAN_POINT ( 'NONE',  ( -17.35626706996358237, 16.20628521381909337, 17.92354375535225586 ) ) ;
#7038=CARTESIAN_POINT ( 'NONE',  ( 19.30730118283918983, -16.27608008926518579, 20.99999999999999645 ) ) ;
#7041=CARTESIAN_POINT ( 'NONE',  ( 20.78373334066920108, -29.14101728923875356, 12.14047268033096927 ) ) ;
#7095=CARTESIAN_POINT ( 'NONE',  ( 3.900486991066101972, 40.17991855518010880, 11.00000000000020250 ) ) ;
#7101=CARTESIAN_POINT ( 'NONE',  ( -9.543723562658518844, 28.97375833662206901, 19.66345542862528362 ) ) ;
#7113=CARTESIAN_POINT ( 'NONE',  ( -4.441848239913464447, 24.85865334748893929, 20.99999999999999645 ) ) ;
#7119=CARTESIAN_POINT ( 'NONE',  ( -18.91631044952799812, -27.33967623494412535, 16.30093088680231972 ) ) ;
#7141=CARTESIAN_POINT ( 'NONE',  ( 32.97049335003973169, -4.716631976065183807, 17.42190598798392998 ) ) ;
#7143=CARTESIAN_POINT ( 'NONE',  ( -12.27395423108443673, 32.91881889271085981, 16.30093088680193603 ) ) ;
#7149=CARTESIAN_POINT ( 'NONE',  ( -1.848241319495560253, 27.98666583367183947, 20.99999999999999645 ) ) ;
#7154=CARTESIAN_POINT ( 'NONE',  ( 21.00262217607745896, 5.738642561615682425, 19.27171037444140111 ) ) ;
#7164=CARTESIAN_POINT ( 'NONE',  ( -27.10945576260561651, -19.90266412673942398, 19.66345542862529072 ) ) ;
#7190=CARTESIAN_POINT ( 'NONE',  ( 22.79731396823020262, -22.36677566318291710, 19.66345542862563178 ) ) ;
#7197=CARTESIAN_POINT ( 'NONE',  ( -7.962467718762158420, 24.71319220551422191, 20.69868183039781329 ) ) ;
#7212=CARTESIAN_POINT ( 'NONE',  ( 32.33143948541787438, 1.358872982501792226, 11.00000000000000000 ) ) ;
#7223=CARTESIAN_POINT ( 'NONE',  ( -16.92376161250139788, -28.83147800495276769, 13.32518128616562869 ) ) ;
#7232=CARTESIAN_POINT ( 'NONE',  ( -1.553811836244973321, 36.85721162268941242, 17.92354375535250810 ) ) ;
#7235=CARTESIAN_POINT ( 'NONE',  ( -19.05502067201149075, 4.384649331638460268, 20.25080042701565830 ) ) ;
#7237=CARTESIAN_POINT ( 'NONE',  ( 19.84741737732757016, -16.23688957394130838, 20.99999999999999645 ) ) ;
#7240=CARTESIAN_POINT ( 'NONE',  ( 26.45121176803958107, -27.84758587393105600, 11.55979286843934695 ) ) ;
#7293=CARTESIAN_POINT ( 'NONE',  ( -9.340438144419696442, 38.00965938231844632, 11.55979286843914799 ) ) ;
#7297=CARTESIAN_POINT ( 'NONE',  ( 1.248251703783664679, 34.03222469610384593, 19.66345542862528362 ) ) ;
#7313=CARTESIAN_POINT ( 'NONE',  ( 3.833852081710638071, 25.75497152300991033, 21.00000000000000355 ) ) ;
#7318=CARTESIAN_POINT ( 'NONE',  ( -34.21349446591933940, -17.75307084757253051, 16.30093088680225222 ) ) ;
#7341=CARTESIAN_POINT ( 'NONE',  ( 35.11176058605620653, -10.96173827525856481, 16.87380292611440424 ) ) ;
#7344=CARTESIAN_POINT ( 'NONE',  ( -11.06388406389812751, 34.19581601475828592, 16.30093088680271052 ) ) ;
#7347=CARTESIAN_POINT ( 'NONE',  ( -2.594149110900493493, 26.80855565015070852, 20.99999999999998934 ) ) ;
#7355=CARTESIAN_POINT ( 'NONE',  ( 23.22986302874564046, 7.287013008514754198, 17.42190598798376300 ) ) ;
#7364=CARTESIAN_POINT ( 'NONE',  ( -28.59012753014036790, -4.062670752122675921, 19.66345542862530493 ) ) ;
#7373=ADVANCED_FACE ( 'NONE', ( #32818 ), #1734, .T. ) ;
#7377=VECTOR ( 'NONE', #12951, 1000.000000000000000 ) ;
#7391=CARTESIAN_POINT ( 'NONE',  ( 28.07442828530308176, -16.20877872786445195, 20.25080042701566541 ) ) ;
#7402=CYLINDRICAL_SURFACE ( 'NONE', #37640, 57.99999999999995737 ) ;
#7425=CARTESIAN_POINT ( 'NONE',  ( -14.98890121934590347, -28.67928442654175214, 11.55979286843934872 ) ) ;
#7435=CARTESIAN_POINT ( 'NONE',  ( -6.320269494896706419, 36.18253918181394369, 17.42190598798392287 ) ) ;
#7441=CARTESIAN_POINT ( 'NONE',  ( -24.79273775960036019, -6.040746354373381699, 20.82122704794079837 ) ) ;
#7443=DIRECTION ( 'NONE',  ( -1.000000000000000000, 0.000000000000000000, 0.000000000000000000 ) ) ;
#7447=CARTESIAN_POINT ( 'NONE',  ( 14.98890121934557307, -28.67928442654207188, 11.55979286843934872 ) ) ;
#7474=CARTESIAN_POINT ( 'NONE',  ( -20.39213822642799201, -16.19729952584802035, 22.99999999999999645 ) ) ;
#7493=ORIENTED_EDGE ( 'NONE', *, *, #29461, .T. ) ;
#7501=CARTESIAN_POINT ( 'NONE',  ( 16.82090372984156801, 29.19711159930561450, 11.55979286843845877 ) ) ;
#7504=CARTESIAN_POINT ( 'NONE',  ( -12.55429062395159079, 25.98950339719647218, 18.87996532025784546 ) ) ;
#7517=CARTESIAN_POINT ( 'NONE',  ( -4.672335726382761401, 24.36080358023105674, 20.99999999999999645 ) ) ;
#7524=CARTESIAN_POINT ( 'NONE',  ( -22.37155630812419105, -27.08896561536066372, 16.30093088680148838 ) ) ;
#7550=CARTESIAN_POINT ( 'NONE',  ( 35.45120626212618475, -5.541700984529022378, 15.13084544680181587 ) ) ;
#7552=CARTESIAN_POINT ( 'NONE',  ( -9.684793793942127138, 35.24386573278048473, 16.30093088680190760 ) ) ;
#7553=CARTESIAN_POINT ( 'NONE',  ( 10.60610353952458773, -24.43405348869776006, 17.42190598798185164 ) ) ;
#7555=CARTESIAN_POINT ( 'NONE',  ( 3.998720052559921356, 27.76176938167571961, 20.94377226548378346 ) ) ;
#7563=CARTESIAN_POINT ( 'NONE',  ( 14.43694901004736586, 26.51279404189499900, 17.42190598798392998 ) ) ;
#7571=CARTESIAN_POINT ( 'NONE',  ( -24.71109915376977284, -20.69862126830784277, 19.99202127657074612 ) ) ;
#7584=ORIENTED_EDGE ( 'NONE', *, *, #16442, .F. ) ;
#7592=CARTESIAN_POINT ( 'NONE',  ( -36.53988293555860878, -0.5802930328944716498, 22.99999999999905853 ) ) ;
#7597=CARTESIAN_POINT ( 'NONE',  ( 23.22759628179494484, -23.81077309377013762, 18.87996532025824337 ) ) ;
#7621=CARTESIAN_POINT ( 'NONE',  ( 22.73075399258359397, -29.06185307675098883, 10.99999999999956124 ) ) ;
#7632=CARTESIAN_POINT ( 'NONE',  ( -22.71963042674493138, -29.00054972838716338, 12.14047268033060156 ) ) ;
#7648=CARTESIAN_POINT ( 'NONE',  ( -9.555312204555107769, 25.15592819202021246, 20.25080042701566541 ) ) ;
#7650=CARTESIAN_POINT ( 'NONE',  ( 24.49409870379991716, -11.70597971641857526, 20.99999999999999645 ) ) ;
#7655=CARTESIAN_POINT ( 'NONE',  ( 36.53369576860747259, -5.154516326609281052, 11.55979286843935760 ) ) ;
#7707=CARTESIAN_POINT ( 'NONE',  ( -3.900486991066871578, 40.17991855517983879, 11.00000000000019007 ) ) ;
#7711=CARTESIAN_POINT ( 'NONE',  ( 10.52848948537593721, 31.43736604633500065, 18.42518152272110044 ) ) ;
#7729=CARTESIAN_POINT ( 'NONE',  ( -15.37000524125038048, -27.20210912714571805, 15.72805884748939498 ) ) ;
#7751=CARTESIAN_POINT ( 'NONE',  ( 20.72701401736302529, -28.35932241216985972, 14.53008259254010959 ) ) ;
#7753=CARTESIAN_POINT ( 'NONE',  ( 15.75274587708552154, 28.77197995862663760, 15.13084544680308063 ) ) ;
#7754=CARTESIAN_POINT ( 'NONE',  ( -16.23042486172771248, -23.86708630543029130, 18.87996532025784902 ) ) ;
#7756=CARTESIAN_POINT ( 'NONE',  ( 0.8051564177163211822, 29.93655406406124797, 20.82122704794079837 ) ) ;
#7757=VECTOR ( 'NONE', #5175, 1000.000000000000000 ) ;
#7766=CARTESIAN_POINT ( 'NONE',  ( 31.72789954390927392, 0.7664678198816438082, 14.53008259254011136 ) ) ;
#7776=CARTESIAN_POINT ( 'NONE',  ( -29.36302367423271065, -15.61102309902027585, 19.99202127657132877 ) ) ;
#7790=CARTESIAN_POINT ( 'NONE',  ( 35.72300736400854504, -23.12593624637943179, 22.99999999999999289 ) ) ;
#7799=VERTEX_POINT ( 'NONE', #23161 ) ;
#7802=CARTESIAN_POINT ( 'NONE',  ( 17.59613548593226540, -24.21943298483269302, 18.87996532025752217 ) ) ;
#7833=CARTESIAN_POINT ( 'NONE',  ( -32.33143948541798096, 1.358872982501892590, 11.00000000000000000 ) ) ;
#7846=CARTESIAN_POINT ( 'NONE',  ( -15.48226359616454495, 8.938689054909644938, 20.50957957746029336 ) ) ;
#7847=CARTESIAN_POINT ( 'NONE',  ( 25.43307211745627328, -8.368469763667489403, 20.94377226548379411 ) ) ;
#7852=CARTESIAN_POINT ( 'NONE',  ( 22.73075399258386398, -29.06185307675093199, 10.99999999999955769 ) ) ;
#7856=EDGE_CURVE ( 'NONE', #17014, #18163, #15579, .T. ) ;
#7908=CARTESIAN_POINT ( 'NONE',  ( -12.17657648715623608, 27.34841683166460058, 18.87996532025750085 ) ) ;
#7926=CARTESIAN_POINT ( 'NONE',  ( -33.86051255203334875, -2.258496953481841096, 15.13084544680166665 ) ) ;
#7941=CARTESIAN_POINT ( 'NONE',  ( -32.57473823703268323, -23.68076927422058731, 10.99999999999993960 ) ) ;
#7942=UNCERTAINTY_MEASURE_WITH_UNIT (LENGTH_MEASURE( 1.000000000000000082E-05 ), #36754, 'distance_accuracy_value', 'NONE');
#7949=CARTESIAN_POINT ( 'NONE',  ( 34.31157940325252298, -4.066883398345114919, 15.72805884748939853 ) ) ;
#7951=CARTESIAN_POINT ( 'NONE',  ( 14.19638663437042503, 32.12978188971815285, 14.53008259254012025 ) ) ;
#7952=CARTESIAN_POINT ( 'NONE',  ( 10.43399472913278103, -25.44514827092724829, 16.30093088679983637 ) ) ;
#7954=CARTESIAN_POINT ( 'NONE',  ( 8.084325832714235105, 26.79336336920809813, 20.50957957746030047 ) ) ;
#7960=VECTOR ( 'NONE', #1912, 1000.000000000000000 ) ;
#7962=CARTESIAN_POINT ( 'NONE',  ( 14.04126239388501496, 8.106726622871901711, 20.82122704794079837 ) ) ;
#7972=CARTESIAN_POINT ( 'NONE',  ( -26.17288861939861988, -20.72787579792414903, 19.66345542862528362 ) ) ;
#7993=CARTESIAN_POINT ( 'NONE',  ( -29.22254794994760729, -28.85350742528338586, 22.99999999999905853 ) ) ;
#7999=CARTESIAN_POINT ( 'NONE',  ( 23.01245512501257551, -23.08877437847652558, 19.27171037444193757 ) ) ;
#8025=CARTESIAN_POINT ( 'NONE',  ( -21.91981567634955397, -15.65087685632102499, 20.99999999999999645 ) ) ;
#8035=CARTESIAN_POINT ( 'NONE',  ( -34.10020663062397972, -21.93670956716203690, 11.00000000000017231 ) ) ;
#8049=CARTESIAN_POINT ( 'NONE',  ( 22.70288158165702086, -17.06695585772177992, 20.94377226548368043 ) ) ;
#8107=CARTESIAN_POINT ( 'NONE',  ( -4.383143208095260590, 35.51174355874280053, 18.42518152272109333 ) ) ;
#8111=( LENGTH_UNIT ( ) NAMED_UNIT ( * ) SI_UNIT ( .MILLI., .METRE. ) );
#8127=CARTESIAN_POINT ( 'NONE',  ( -26.23899120466318280, -27.34191102820705055, 13.92931973827808534 ) ) ;
#8153=CARTESIAN_POINT ( 'NONE',  ( 18.87563634320844130, -28.49365729390225965, 14.53008259254033163 ) ) ;
#8156=CARTESIAN_POINT ( 'NONE',  ( -10.19952947928024933, 35.92118758406519419, 15.13084544680213384 ) ) ;
#8157=CARTESIAN_POINT ( 'NONE',  ( 5.178899460637698127, -25.25135431486990711, 15.72805884748939853 ) ) ;
#8159=CARTESIAN_POINT ( 'NONE',  ( 1.610977985362757936, 29.80447555512223445, 20.82122704794079482 ) ) ;
#8170=CARTESIAN_POINT ( 'NONE',  ( 7.164929079092710928, 24.49151390637290149, 20.82122704794079837 ) ) ;
#8180=CARTESIAN_POINT ( 'NONE',  ( -21.83517059620288236, -24.14399886393494299, 18.87996532025750795 ) ) ;
#8194=CARTESIAN_POINT ( 'NONE',  ( 20.38753357181587234, -16.19769905861744519, 23.00000000000000000 ) ) ;
#8199=CARTESIAN_POINT ( 'NONE',  ( -34.33271597228865346, -24.82403720151219417, 23.00000000000000000 ) ) ;
#8206=CARTESIAN_POINT ( 'NONE',  ( 30.59706755222660135, -4.299425952516082283, 18.87996532025822916 ) ) ;
#8207=AXIS2_PLACEMENT_3D ( 'NONE', #26275, #13886, #32175 ) ;
#8226=CARTESIAN_POINT ( 'NONE',  ( -5.067385705950865571, -26.57793081542402547, 12.73282698324853257 ) ) ;
#8229=AXIS2_PLACEMENT_3D ( 'NONE', #28619, #3836, #16237 ) ;
#8230=CARTESIAN_POINT ( 'NONE',  ( -24.51396478725073536, -11.15767879383071737, 20.99999999999999645 ) ) ;
#8239=CARTESIAN_POINT ( 'NONE',  ( -31.34430980808800626, -24.70897660846286570, 12.14047268033097282 ) ) ;
#8253=CARTESIAN_POINT ( 'NONE',  ( 21.72603204741341898, -16.58852365944996166, 20.99999999999999645 ) ) ;
#8258=AXIS2_PLACEMENT_3D ( 'NONE', #21779, #256, #25032 ) ;
#8259=CIRCLE ( 'NONE', #12149, 17.99999999999993250 ) ;
#8287=CARTESIAN_POINT ( 'NONE',  ( 25.22779561345564758, -30.53001674459726189, 11.00000000000000178 ) ) ;
#8295=B_SPLINE_CURVE_WITH_KNOTS ( 'NONE', 3,
 ( #22171, #21771, #45, #16283, #448, #9985 ),
 .UNSPECIFIED., .F., .F.,
 ( 4, 2, 4 ),
 ( 0.000000000000000000, 0.5000000000000000000, 1.000000000000000000 ),
 .UNSPECIFIED. ) ;
#8296=VERTEX_POINT ( 'NONE', #19063 ) ;
#8300=B_SPLINE_CURVE_WITH_KNOTS ( 'NONE', 3,
 ( #26737, #24484, #5801, #29985, #36292, #33253 ),
 .UNSPECIFIED., .F., .F.,
 ( 4, 2, 4 ),
 ( 0.000000000000000000, 0.5000000000000000000, 1.000000000000000000 ),
 .UNSPECIFIED. ) ;
#8302=APPLICATION_CONTEXT ( 'automotive_design' ) ;
#8318=CARTESIAN_POINT ( 'NONE',  ( 17.34253826607184479, 27.32041144404033162, 11.00000000000000000 ) ) ;
#8339=CARTESIAN_POINT ( 'NONE',  ( -36.37100582830133533, -12.78888441968056000, 15.13084544680203258 ) ) ;
#8354=CARTESIAN_POINT ( 'NONE',  ( -35.04557732017523364, -20.40215588137732894, 10.99999999999994138 ) ) ;
#8362=CARTESIAN_POINT ( 'NONE',  ( 29.43343111547206448, -25.34807889869614073, 14.53008259253982892 ) ) ;
#8364=CARTESIAN_POINT ( 'NONE',  ( -3.717128218779113702, 39.34929362537324948, 14.53008259254020551 ) ) ;
#8365=CARTESIAN_POINT ( 'NONE',  ( 4.276224980513730623E-14, -25.25135431486990711, 15.72805884748939853 ) ) ;
#8367=CARTESIAN_POINT ( 'NONE',  ( 2.905187527479470067, 31.12430299512154264, 20.50957957746028626 ) ) ;
#8378=CARTESIAN_POINT ( 'NONE',  ( 11.08993573033173696, 19.63476728479018973, 20.25080042701548777 ) ) ;
#8389=CARTESIAN_POINT ( 'NONE',  ( -32.48980236688448997, -6.600743665353513201, 18.42518152272148413 ) ) ;
#8414=CARTESIAN_POINT ( 'NONE',  ( 16.05557028316289347, -24.54483004364954368, 18.42518152272108622 ) ) ;
#8433=CARTESIAN_POINT ( 'NONE',  ( -5.050662510305666153, -26.77689918168226058, 11.00000000000000000 ) ) ;
#8437=CARTESIAN_POINT ( 'NONE',  ( -24.20198940123846398, -6.620595927252818313, 20.94377226548378701 ) ) ;
#8461=CARTESIAN_POINT ( 'NONE',  ( 22.36336935241927293, -18.10715803802170498, 20.82122704794078771 ) ) ;
#8500=CARTESIAN_POINT ( 'NONE',  ( -31.24272016124701068, 0.2902395683534709780, 15.72805884748939853 ) ) ;
#8510=VERTEX_POINT ( 'NONE', #23513 ) ;
#8540=B_SPLINE_CURVE_WITH_KNOTS ( 'NONE', 3,
 ( #13416, #435, #31508, #25810, #38205, #32109, #10377, #4274, #10779, #4876, #36366, #32926, #14020, #29860, #1638, #5280, #20328, #16884 ),
 .UNSPECIFIED., .F., .F.,
 ( 4, 2, 2, 2, 2, 2, 2, 2, 4 ),
 ( 0.000000000000000000, 0.1250000000000000000, 0.2500000000000000000, 0.3750000000000000000, 0.5000000000000000000, 0.6250000000000000000, 0.7500000000000000000, 0.8750000000000000000, 1.000000000000000000 ),
 .UNSPECIFIED. ) ;
#8545=EDGE_LOOP ( 'NONE', ( #15980, #6196, #4006, #35706 ) ) ;
#8556=CARTESIAN_POINT ( 'NONE',  ( 35.54328883424830110, -18.34041411986698478, 13.92931973827811909 ) ) ;
#8558=CARTESIAN_POINT ( 'NONE',  ( -1.387327393066717074E-13, 39.65430245495500117, 14.53008259254011136 ) ) ;
#8561=CARTESIAN_POINT ( 'NONE',  ( -1.971557875515829616, 31.43880600153361371, 20.50957957746028271 ) ) ;
#8563=VERTEX_POINT ( 'NONE', #11330 ) ;
#8568=CARTESIAN_POINT ( 'NONE',  ( 24.79273775960175996, -6.040746354374877392, 20.82122704794079837 ) ) ;
#8580=CARTESIAN_POINT ( 'NONE',  ( -29.77271197308770212, -3.128983846831010496, 18.87996532025785967 ) ) ;
#8596=CARTESIAN_POINT ( 'NONE',  ( 24.49409870379991716, -11.70597971641860191, 23.00000000000000000 ) ) ;
#8607=CARTESIAN_POINT ( 'NONE',  ( 22.18734415243709179, -26.07761308992911964, 17.42190598798388379 ) ) ;
#8627=CARTESIAN_POINT ( 'NONE',  ( 18.23649648353767461, -16.09146789626181118, 23.00000000000000000 ) ) ;
#8631=CARTESIAN_POINT ( 'NONE',  ( -15.03860650580051761, -28.48662463501835163, 12.73282698324853257 ) ) ;
#8632=ORIENTED_EDGE ( 'NONE', *, *, #17283, .T. ) ;
#8634=CARTESIAN_POINT ( 'NONE',  ( -25.82310832280115775, -13.25591304976905427, 20.94377226548378346 ) ) ;
#8647=CARTESIAN_POINT ( 'NONE',  ( -18.76090689389219435, -16.22676322417297357, 21.00000000000000000 ) ) ;
#8662=CARTESIAN_POINT ( 'NONE',  ( 25.03753813966995168, -13.00734255224419655, 20.99999999999999645 ) ) ;
#8664=CARTESIAN_POINT ( 'NONE',  ( 34.83525826321753271, -1.648928274806267025, 10.99999999999992006 ) ) ;
#8693=CARTESIAN_POINT ( 'NONE',  ( 31.08218588373089020, -27.68808745788718895, 11.00000000000000178 ) ) ;
#8720=( NAMED_UNIT ( * ) SI_UNIT ( $, .STERADIAN. ) SOLID_ANGLE_UNIT ( ) );
#8722=CARTESIAN_POINT ( 'NONE',  ( 19.48557158514982746, -11.25000000000009415, 23.00000000000000000 ) ) ;
#8736=FACE_OUTER_BOUND ( 'NONE', #5315, .T. ) ;
#8741=ADVANCED_FACE ( 'NONE', ( #17640 ), #32236, .T. ) ;
#8757=ORIENTED_EDGE ( 'NONE', *, *, #16309, .T. ) ;
#8759=CARTESIAN_POINT ( 'NONE',  ( 27.98024382195362136, -26.61114576561526590, 13.92931973827785086 ) ) ;
#8761=CARTESIAN_POINT ( 'NONE',  ( 12.06278152636307865, 35.25200209733485934, 13.92931973827804626 ) ) ;
#8763=CARTESIAN_POINT ( 'NONE',  ( -12.28720923544494248, -14.55658080566520418, 20.99999999999999645 ) ) ;
#8765=CARTESIAN_POINT ( 'NONE',  ( -7.604803157139289560, 28.95581125563456126, 20.25080042701564764 ) ) ;
#8772=CARTESIAN_POINT ( 'NONE',  ( 16.18987435794473839, 9.347228318705804284, 20.25080042701566541 ) ) ;
#8786=CARTESIAN_POINT ( 'NONE',  ( -29.45678984391951616, -18.54179626184216545, 19.27171037444122703 ) ) ;
#8802=CARTESIAN_POINT ( 'NONE',  ( 39.59914439355202376, -10.88071517532279309, 11.00000000000000000 ) ) ;
#8806=CARTESIAN_POINT ( 'NONE',  ( -16.58691282011820078, -31.15705289669412181, 11.00000000000000000 ) ) ;
#8811=CARTESIAN_POINT ( 'NONE',  ( 31.72869323525675966, -3.591677789202227800, 17.92354375535289890 ) ) ;
#8826=MANIFOLD_SOLID_BREP ( 'Shell1', #26159 ) ;
#8832=CARTESIAN_POINT ( 'NONE',  ( 5.050662510307052600, -26.77689918168226058, 11.55979286843934872 ) ) ;
#8835=CARTESIAN_POINT ( 'NONE',  ( -22.36336935241945767, -18.10715803802132484, 20.82122704794079837 ) ) ;
#8861=CARTESIAN_POINT ( 'NONE',  ( 26.86294352747594516, -10.31366695439891679, 20.82122704794079837 ) ) ;
#8877=CARTESIAN_POINT ( 'NONE',  ( -14.48927117870118408, -30.61587158504671535, 22.99999999999999645 ) ) ;
#8887=CARTESIAN_POINT ( 'NONE',  ( 31.94006737154955644, 0.9747213384812106751, 13.92931973827808712 ) ) ;
#8891=CARTESIAN_POINT ( 'NONE',  ( 37.88915196488844117, -19.37406374111511198, 11.00000000000000000 ) ) ;
#8903=CARTESIAN_POINT ( 'NONE',  ( -32.33143948541790991, 1.358872982501832860, 11.00000000000000000 ) ) ;
#8962=CARTESIAN_POINT ( 'NONE',  ( 7.450289500751110516, 38.62958991718475943, 13.32518128616595199 ) ) ;
#8965=CARTESIAN_POINT ( 'NONE',  ( 18.23649648353778474, -16.09146789626167262, 20.99999999999999645 ) ) ;
#8968=CARTESIAN_POINT ( 'NONE',  ( 8.231377095499450292, 29.48763288632292756, 19.99202127657103389 ) ) ;
#8972=CARTESIAN_POINT ( 'NONE',  ( -17.34253826607186966, 27.32041144404028188, 11.00000000000000000 ) ) ;
#8984=CARTESIAN_POINT ( 'NONE',  ( -32.65234849725306532, -15.41672394535184054, 18.42518152272107557 ) ) ;
#9007=CARTESIAN_POINT ( 'NONE',  ( 30.82027224585396397, -2.301877357437541072, 17.92354375535443722 ) ) ;
#9014=CARTESIAN_POINT ( 'NONE',  ( -15.12590024503300512, -28.14827041158709875, 13.92931973827808534 ) ) ;
#9019=B_SPLINE_SURFACE_WITH_KNOTS ( 'NONE', 3, 3, ( 
 ( #14322, #1533, #26715, #39703, #8433, #24069, #11680 ),
 ( #11481, #2731, #8832, #24267, #9029, #20632, #23868 ),
 ( #20830, #2341, #33032, #17983, #15122, #5180, #39896 ),
 ( #27511, #30373, #36064, #36462, #8226, #36662, #8631 ),
 ( #5573, #36270, #21218, #2538, #33231, #12072, #39504 ),
 ( #24462, #33433, #14522, #21023, #11876, #33629, #5778 ),
 ( #18179, #30573, #17592, #27117, #14926, #29960, #36860 ),
 ( #2140, #5378, #27314, #14727, #26915, #39303, #30168 ),
 ( #17793, #35797, #8157, #8365, #29094, #2075, #32556 ),
 ( #36201, #7952, #38438, #11213, #1267, #14254, #26646 ),
 ( #14450, #20365, #13853, #26847, #10610, #1878, #11018 ),
 ( #38841, #7553, #5114, #10813, #13651, #32959, #29495 ),
 ( #29297, #32352, #23402, #1467, #17521, #38638, #32757 ),
 ( #4913, #39034, #17320, #4513, #23200, #29695, #23798 ),
 ( #29893, #26243, #35599, #26038, #32144, #4715, #7754 ),
 ( #20159, #17119, #39236, #1670, #20562, #23603, #14050 ),
 ( #4308, #26443, #35395, #22991, #11416, #36001, #16710 ),
 ( #19957, #16915, #12206, #30505, #18309, #2666, #14659 ),
 ( #15052, #9162, #17918, #30700, #11809, #30301, #27845 ),
 ( #15255, #3060, #27245, #24794, #24195, #21354, #2474 ),
 ( #14860, #27442, #39830, #33559, #27643, #39634, #20765 ),
 ( #36592, #17722, #30898, #21151, #33161, #37191, #24397 ),
 ( #40025, #30097, #2865, #24600, #36992, #15454, #36789 ),
 ( #18, #27050, #21545, #12007, #33945, #33761, #39435 ),
 ( #8965, #5907, #33362, #6103, #18508, #8763, #12402 ) ),
 .UNSPECIFIED., .F., .F., .F.,
 ( 4, 3, 3, 3, 3, 3, 3, 3, 4 ),
 ( 4, 3, 4 ),
 ( 0.000000000000000000, 0.1250000000000000000, 0.2500000000000000000, 0.3750000000000000000, 0.5000000000000000000, 0.6250000000000000000, 0.7500000000000000000, 0.8750000000000000000, 1.000000000000000000 ),
 ( 1.318307113131750086, 1.570796326794896336, 1.823285540458042586 ),
 .UNSPECIFIED. ) ;
#9029=CARTESIAN_POINT ( 'NONE',  ( -5.050662510306967334, -26.77689918168226058, 11.55979286843934872 ) ) ;
#9032=CARTESIAN_POINT ( 'NONE',  ( -19.25011873046071642, -17.89323911765397312, 20.94377226548387583 ) ) ;
#9033=EDGE_CURVE ( 'NONE', #1139, #16240, #11422, .T. ) ;
#9060=CARTESIAN_POINT ( 'NONE',  ( 26.19533169775624160, -16.15700992729039598, 20.69868183039781329 ) ) ;
#9068=CARTESIAN_POINT ( 'NONE',  ( -33.75875814100324135, 2.759858869446476959, 11.00000000000000000 ) ) ;
#9087=CARTESIAN_POINT ( 'NONE',  ( 31.51573171626900205, 0.5582143012820770522, 15.13084544680213561 ) ) ;
#9092=CARTESIAN_POINT ( 'NONE',  ( -36.56052011373579802, -7.179325806537445231, 13.92931973827734993 ) ) ;
#9101=CARTESIAN_POINT ( 'NONE',  ( -28.63966609530878671, 4.835996017633398480, 12.73282698325538398 ) ) ;
#9114=CARTESIAN_POINT ( 'NONE',  ( 19.26948696230200397, 27.85601271560037162, 11.00000000000000000 ) ) ;
#9128=CARTESIAN_POINT ( 'NONE',  ( 3.833852081710629189, 25.75497152300991033, 23.00000000000000355 ) ) ;
#9160=CARTESIAN_POINT ( 'NONE',  ( 3.857345576530424758, 39.98449713665801397, 12.73282698324868711 ) ) ;
#9162=CARTESIAN_POINT ( 'NONE',  ( 11.45923940083702597, -19.42154971127180474, 20.25080042701502947 ) ) ;
#9164=CARTESIAN_POINT ( 'NONE',  ( 2.148627388802076599, 32.24135036777348517, 20.25080042701565475 ) ) ;
#9182=CARTESIAN_POINT ( 'NONE',  ( -33.78274305024888946, -17.56282548559296330, 16.87380292611478438 ) ) ;
#9207=CARTESIAN_POINT ( 'NONE',  ( 15.74227866053861469, -25.75916161678320648, 17.42190598798392642 ) ) ;
#9217=CARTESIAN_POINT ( 'NONE',  ( 18.17912400184410160, 22.26280294335838406, 13.92931973826196490 ) ) ;
#9228=CARTESIAN_POINT ( 'NONE',  ( -20.82679924176412811, -18.60878591099491786, 20.82122704794066337 ) ) ;
#9255=CARTESIAN_POINT ( 'NONE',  ( -38.62508484777313811, -17.24896845009202551, 11.00000000000000355 ) ) ;
#9256=CARTESIAN_POINT ( 'NONE',  ( 26.01028601707371379, -6.099477938990075288, 20.69868183039873699 ) ) ;
#9271=LINE ( 'NONE', #22442, #11663 ) ;
#9291=CARTESIAN_POINT ( 'NONE',  ( -36.01431143412934688, -5.340261033854917017, 13.92931973827854719 ) ) ;
#9304=CARTESIAN_POINT ( 'NONE',  ( -19.89620541518657859, 17.40116461633755307, 14.53008259253898693 ) ) ;
#9317=CARTESIAN_POINT ( 'NONE',  ( 20.57678504259613561, 23.15270735499986898, 22.99999999999999645 ) ) ;
#9332=CARTESIAN_POINT ( 'NONE',  ( 0.5415361484146484772, 27.50000000000004974, 23.00000000000000000 ) ) ;
#9363=CARTESIAN_POINT ( 'NONE',  ( -9.237168799398533636, 37.83823547837186396, 12.73282698324810625 ) ) ;
#9367=CARTESIAN_POINT ( 'NONE',  ( -10.03134041160988943, 26.49437744576609788, 19.99202127657076744 ) ) ;
#9372=CARTESIAN_POINT ( 'NONE',  ( -10.34254640628272348, 25.37474234119853023, 19.99202127657103745 ) ) ;
#9382=CARTESIAN_POINT ( 'NONE',  ( -31.31527935466932888, -1.911037205182263943, 17.42190598798389800 ) ) ;
#9406=CARTESIAN_POINT ( 'NONE',  ( 24.08646667827958154, -13.28101593840524153, 20.99999999999998934 ) ) ;
#9407=CARTESIAN_POINT ( 'NONE',  ( 28.56250045050212805, -21.55178514600707373, 18.42518152272109333 ) ) ;
#9412=EDGE_CURVE ( 'NONE', #18297, #7799, #4654, .T. ) ;
#9414=CARTESIAN_POINT ( 'NONE',  ( 4.672335726383261445, 24.36080358023195913, 20.99999999999999645 ) ) ;
#9431=CARTESIAN_POINT ( 'NONE',  ( -26.87422832650623405, -16.65342898056120191, 20.50957957746005889 ) ) ;
#9460=CARTESIAN_POINT ( 'NONE',  ( 18.28744585352691132, -19.47582948098743216, 20.69868183039766407 ) ) ;
#9466=DIRECTION ( 'NONE',  ( 1.000000000000000000, 0.000000000000000000, -0.000000000000000000 ) ) ;
#9467=CARTESIAN_POINT ( 'NONE',  ( -20.57678504272164943, 23.15270735504455146, 11.00000000000000000 ) ) ;
#9494=CARTESIAN_POINT ( 'NONE',  ( -35.65094714181024216, -16.36533849799707596, 15.13084544680223509 ) ) ;
#9499=CARTESIAN_POINT ( 'NONE',  ( -18.23649648353780961, -16.09146789626143814, 20.99999999999999645 ) ) ;
#9503=CARTESIAN_POINT ( 'NONE',  ( -30.17922767059062039, -0.7536324250866187624, 17.42190598798392998 ) ) ;
#9509=CARTESIAN_POINT ( 'NONE',  ( 34.11403513953423783, -2.099922846023814849, 14.53008259254038848 ) ) ;
#9518=EDGE_CURVE ( 'NONE', #3967, #18163, #8540, .T. ) ;
#9562=CARTESIAN_POINT ( 'NONE',  ( 16.76301160834832871, 29.17407194212043464, 12.14047268033043103 ) ) ;
#9566=CARTESIAN_POINT ( 'NONE',  ( -10.24445352883136984, 27.94073041968543691, 19.66345542862531204 ) ) ;
#9583=CARTESIAN_POINT ( 'NONE',  ( -34.90004137879623158, -9.293601764824154898, 16.87380292611441490 ) ) ;
#9592=AXIS2_PLACEMENT_3D ( 'NONE', #37380, #24782, #15042 ) ;
#9609=CARTESIAN_POINT ( 'NONE',  ( 20.61005271883062306, -26.74738414229423000, 16.87380292611441845 ) ) ;
#9612=DIRECTION ( 'NONE',  ( -0.000000000000000000, -0.000000000000000000, -1.000000000000000000 ) ) ;
#9623=CARTESIAN_POINT ( 'NONE',  ( 20.66414367076000858, 17.76245163070478839, 11.55979286843843390 ) ) ;
#9633=CARTESIAN_POINT ( 'NONE',  ( -28.41077021456755958, -6.925791943820290619, 20.25080042701566541 ) ) ;
#9662=CARTESIAN_POINT ( 'NONE',  ( 27.85940672053917311, -14.94704994757669780, 20.50957957746029336 ) ) ;
#9687=CARTESIAN_POINT ( 'NONE',  ( 33.69589222704784248, -0.03122585499641188089, 11.00000000000003908 ) ) ;
#9697=CARTESIAN_POINT ( 'NONE',  ( -33.82738586796177316, -21.73727074213755728, 13.32518128616597153 ) ) ;
#9706=CARTESIAN_POINT ( 'NONE',  ( -26.89145897433321863, 3.386615419929385418, 16.87380292612052202 ) ) ;
#9710=B_SPLINE_CURVE_WITH_KNOTS ( 'NONE', 3,
 ( #4259, #35950, #32910, #19700, #10561, #32092 ),
 .UNSPECIFIED., .F., .F.,
 ( 4, 2, 4 ),
 ( 0.000000000000000000, 0.5000000000000001110, 1.000000000000000000 ),
 .UNSPECIFIED. ) ;
#9713=CARTESIAN_POINT ( 'NONE',  ( 33.65490896085587735, -21.61118400457290534, 13.92931973827805336 ) ) ;
#9718=CARTESIAN_POINT ( 'NONE',  ( 6.462764152049920163, 17.91932574229958419, 23.00000000000000000 ) ) ;
#9730=CARTESIAN_POINT ( 'NONE',  ( 10.37659644360210542, 39.73422260060681310, 11.00000000000000000 ) ) ;
#9761=CARTESIAN_POINT ( 'NONE',  ( -14.73160032165950284, 32.49283138996943165, 12.73282698324853079 ) ) ;
#9762=DIRECTION ( 'NONE',  ( 0.000000000000000000, 0.000000000000000000, 1.000000000000000000 ) ) ;
#9764=CARTESIAN_POINT ( 'NONE',  ( 3.920592112299155829, 34.13862021880822084, 19.27171037444156809 ) ) ;
#9782=CARTESIAN_POINT ( 'NONE',  ( -33.72852460920479700, -9.442290196615397591, 17.92354375535250810 ) ) ;
#9805=CARTESIAN_POINT ( 'NONE',  ( 17.16434664249021225, -27.18154623538450565, 16.30093088680120417 ) ) ;
#9808=LINE ( 'NONE', #31540, #20852 ) ;
#9809=CARTESIAN_POINT ( 'NONE',  ( 2.787905735463452661, 28.53453732066309811, 20.94377226548378701 ) ) ;
#9817=CARTESIAN_POINT ( 'NONE',  ( 28.79337657215624802, 4.963436916936684540, 10.99999999998960654 ) ) ;
#9824=CARTESIAN_POINT ( 'NONE',  ( -28.99614216520755150, -14.25990928191762919, 20.25080042701565120 ) ) ;
#9850=CARTESIAN_POINT ( 'NONE',  ( 30.00904163739988206, -13.36872314231647607, 19.99202127657103389 ) ) ;
#9872=CARTESIAN_POINT ( 'NONE',  ( 36.53369576860742995, -5.154516326609290822, 11.00000000000008527 ) ) ;
#9883=CARTESIAN_POINT ( 'NONE',  ( -26.37421498764311778, -27.66411951031046357, 12.73282698324853257 ) ) ;
#9892=CARTESIAN_POINT ( 'NONE',  ( 13.31084379716732613, 29.56959138546320887, 17.42190598798392287 ) ) ;
#9896=CARTESIAN_POINT ( 'NONE',  ( -14.01880647376396993, 20.72057097100359968, 18.87996532025877627 ) ) ;
#9905=CARTESIAN_POINT ( 'NONE',  ( 29.72906145568107306, -25.76693493179220340, 13.32518128616587560 ) ) ;
#9927=CARTESIAN_POINT ( 'NONE',  ( 18.68934290553362132, 29.94321432092800350, 11.00000000000000000 ) ) ;
#9947=CARTESIAN_POINT ( 'NONE',  ( -23.05386822411323422, -7.747535282638357224, 20.99999999999999645 ) ) ;
#9956=CARTESIAN_POINT ( 'NONE',  ( -15.98961535660673938, 30.99268274074335494, 11.55979286843903608 ) ) ;
#9958=CARTESIAN_POINT ( 'NONE',  ( -18.72695399103857739, -3.339292870217068998, 23.00000000000000355 ) ) ;
#9959=CARTESIAN_POINT ( 'NONE',  ( -1.410291641398624174, 35.53022820328502007, 18.87996532025784546 ) ) ;
#9960=STYLED_ITEM ( 'NONE', ( #21657 ), #8826 ) ;
#9973=CARTESIAN_POINT ( 'NONE',  ( 1.082972213713614407, 27.41125570341916529, 20.99999999999998934 ) ) ;
#9978=CARTESIAN_POINT ( 'NONE',  ( -33.08367492452225633, -6.388370399452986348, 17.92354375535292021 ) ) ;
#9985=CARTESIAN_POINT ( 'NONE',  ( -14.98890121934603314, -28.67928442654204346, 11.00000000000000000 ) ) ;
#10000=CARTESIAN_POINT ( 'NONE',  ( 33.34742602403141376, -19.25314539175541384, 16.30093088680190405 ) ) ;
#10002=CARTESIAN_POINT ( 'NONE',  ( -11.38745366800335646, 34.53793118711397625, 15.72805884749017835 ) ) ;
#10004=CARTESIAN_POINT ( 'NONE',  ( 6.175735745372842089, 24.95935742585800199, 20.94377226548417781 ) ) ;
#10013=CARTESIAN_POINT ( 'NONE',  ( 20.48347041321109430, 17.67745015983098966, 12.73282698324788953 ) ) ;
#10022=CARTESIAN_POINT ( 'NONE',  ( -23.50870743262444762, -18.52420134090459314, 20.69868183039763210 ) ) ;
#10023=DIRECTION ( 'NONE',  ( 1.000000000000000000, 0.000000000000000000, 0.000000000000000000 ) ) ;
#10042=FACE_OUTER_BOUND ( 'NONE', #36056, .T. ) ;
#10049=CARTESIAN_POINT ( 'NONE',  ( 28.99614216520691912, -14.25990928191685470, 20.25080042701567606 ) ) ;
#10057=DIRECTION ( 'NONE',  ( -1.000000000000000000, 0.000000000000000000, 0.000000000000000000 ) ) ;
#10074=CARTESIAN_POINT ( 'NONE',  ( 34.10020663062358182, -21.93670956716295350, 10.99999999999994138 ) ) ;
#10084=CARTESIAN_POINT ( 'NONE',  ( -31.16314261583334044, -24.50336240592838521, 13.32518128616608699 ) ) ;
#10093=CARTESIAN_POINT ( 'NONE',  ( -12.85888779259178705, 31.22252129899196049, 16.87380292611441135 ) ) ;
#10097=CARTESIAN_POINT ( 'NONE',  ( -23.68624114773478695, 7.604278122839970955, 16.87380292611488741 ) ) ;
#10102=CARTESIAN_POINT ( 'NONE',  ( 18.84567888139518388, -29.34375185562596045, 11.55979286843977327 ) ) ;
#10112=ORIENTED_EDGE ( 'NONE', *, *, #23517, .T. ) ;
#10116=AXIS2_PLACEMENT_3D ( 'NONE', #25113, #534, #35057 ) ;
#10127=CARTESIAN_POINT ( 'NONE',  ( -15.33540832684527544, 35.51988609203762337, 22.99999999999999289 ) ) ;
#10155=ORIENTED_EDGE ( 'NONE', *, *, #30745, .T. ) ;
#10159=CARTESIAN_POINT ( 'NONE',  ( -10.85362879025592342, 36.78189293023367412, 12.14047268033097282 ) ) ;
#10163=CARTESIAN_POINT ( 'NONE',  ( 11.57511119655671372, 28.64756621199167697, 18.87996532025786678 ) ) ;
#10181=CARTESIAN_POINT ( 'NONE',  ( -35.82891851945787209, -9.175709056024100363, 15.72805884748939498 ) ) ;
#10202=CARTESIAN_POINT ( 'NONE',  ( 17.09641143070718172, -27.64751350299042443, 15.72805884748858318 ) ) ;
#10204=CARTESIAN_POINT ( 'NONE',  ( 14.97434053993231196, 30.45331253196302512, 15.13084544680209831 ) ) ;
#10206=CARTESIAN_POINT ( 'NONE',  ( -5.469228652590086170, 26.20992143183283574, 20.94377226548378346 ) ) ;
#10211=CARTESIAN_POINT ( 'NONE',  ( 28.14004025856615954, 4.421764093219024083, 14.53008259254450429 ) ) ;
#10220=CARTESIAN_POINT ( 'NONE',  ( -27.45400382858790067, -18.53605996571844727, 19.99202127657103745 ) ) ;
#10246=CARTESIAN_POINT ( 'NONE',  ( 27.10945576260617429, -19.90266412673917529, 19.66345542862529783 ) ) ;
#10282=CARTESIAN_POINT ( 'NONE',  ( -28.08361064019272391, -26.79812557672154938, 13.32518128616592001 ) ) ;
#10291=CARTESIAN_POINT ( 'NONE',  ( -4.783493507398182132, 36.70021839994218027, 17.42190598798394063 ) ) ;
#10297=CARTESIAN_POINT ( 'NONE',  ( -29.28423149095161904, -1.632116715639065241, 18.42518152272108978 ) ) ;
#10299=CARTESIAN_POINT ( 'NONE',  ( 23.19735768193471870, -14.64350930037810095, 20.99999999999999645 ) ) ;
#10302=CARTESIAN_POINT ( 'NONE',  ( 16.87498849720631711, -29.16588574430777925, 11.55979286843775000 ) ) ;
#10335=DIRECTION ( 'NONE',  ( 0.000000000000000000, 0.000000000000000000, 1.000000000000000000 ) ) ;
#10336=CARTESIAN_POINT ( 'NONE',  ( -37.50916529491303919, -2.485117785107662680, 11.00000000000000000 ) ) ;
#10358=CARTESIAN_POINT ( 'NONE',  ( -14.84499459426757184, 32.56974970312059270, 12.14047268033097282 ) ) ;
#10361=CARTESIAN_POINT ( 'NONE',  ( 6.977707682420476232, 31.68171018602294708, 19.66345542862528006 ) ) ;
#10366=EDGE_CURVE ( 'NONE', #10384, #38528, #26790, .T. ) ;
#10377=CARTESIAN_POINT ( 'NONE',  ( 15.37000524124839274, -27.20210912714562212, 15.72805884748939498 ) ) ;
#10381=CARTESIAN_POINT ( 'NONE',  ( -17.16434664248912512, -27.18154623538578107, 16.30093088680177615 ) ) ;
#10384=VERTEX_POINT ( 'NONE', #21080 ) ;
#10406=CARTESIAN_POINT ( 'NONE',  ( 34.21349446592028443, -17.75307084757209353, 16.30093088680191826 ) ) ;
#10408=CARTESIAN_POINT ( 'NONE',  ( -1.359097634403079240E-13, 39.35700678546972853, 15.13084544680213739 ) ) ;
#10410=CARTESIAN_POINT ( 'NONE',  ( 2.109751222703333706, 28.76298082888545338, 20.94377226548378346 ) ) ;
#10415=CARTESIAN_POINT ( 'NONE',  ( 18.42861860568664056, 16.71074749267215154, 16.87380292611454280 ) ) ;
#10424=CARTESIAN_POINT ( 'NONE',  ( -20.26242815737374769, -21.95648885305439180, 19.99202127657103389 ) ) ;
#10450=CARTESIAN_POINT ( 'NONE',  ( 30.13477841296669979, -9.898407001805262340, 19.99202127657102679 ) ) ;
#10458=CARTESIAN_POINT ( 'NONE',  ( -37.48557158514991272, -11.24999999999982414, 2.999999999999999112 ) ) ;
#10473=FACE_OUTER_BOUND ( 'NONE', #2903, .T. ) ;
#10485=CARTESIAN_POINT ( 'NONE',  ( -36.42486030274168485, -16.61012894281843444, 13.32518128616628950 ) ) ;
#10489=ORIENTED_EDGE ( 'NONE', *, *, #30406, .F. ) ;
#10494=CARTESIAN_POINT ( 'NONE',  ( 1.553811836244721745, 36.85721162268941242, 17.92354375535250810 ) ) ;
#10500=CYLINDRICAL_SURFACE ( 'NONE', #36798, 18.00000000000002132 ) ;
#10501=CARTESIAN_POINT ( 'NONE',  ( 23.74719310098116765, -8.578385743975788458, 23.00000000000001066 ) ) ;
#10504=CARTESIAN_POINT ( 'NONE',  ( 35.86478881511180816, -18.48242683698199329, 12.73282698324857876 ) ) ;
#10531=CARTESIAN_POINT ( 'NONE',  ( -24.49490654608537454, -11.70163678053536316, 23.00000000000000355 ) ) ;
#10539=CARTESIAN_POINT ( 'NONE',  ( -24.51396478725073180, -11.15767879383071559, 20.99999999999999645 ) ) ;
#10550=CARTESIAN_POINT ( 'NONE',  ( -24.20198940123769304, -6.620595927252166391, 20.94377226548377635 ) ) ;
#10552=ORIENTED_EDGE ( 'NONE', *, *, #4683, .T. ) ;
#10557=VERTEX_POINT ( 'NONE', #33344 ) ;
#10559=CARTESIAN_POINT ( 'NONE',  ( 5.746222359017451708, 39.55816310746059372, 11.55979286843935405 ) ) ;
#10561=CARTESIAN_POINT ( 'NONE',  ( 6.462764152049919275, 17.91932574229959130, 20.99999999999999289 ) ) ;
#10563=CARTESIAN_POINT ( 'NONE',  ( -8.307596863006601495, 33.43166269068522212, 18.42518152272108622 ) ) ;
#10583=CARTESIAN_POINT ( 'NONE',  ( -35.28408311606106906, -16.24929212132110123, 15.72805884748946426 ) ) ;
#10601=CARTESIAN_POINT ( 'NONE',  ( -20.51299636258527315, -31.28130022544801392, 10.99999999999999645 ) ) ;
#10607=CARTESIAN_POINT ( 'NONE',  ( 22.57839169151760217, -28.22498753043745978, 14.53008259253988577 ) ) ;
#10609=CARTESIAN_POINT ( 'NONE',  ( -5.259215691052897768, 38.11244126491425277, 15.72805884748939853 ) ) ;
#10610=CARTESIAN_POINT ( 'NONE',  ( -5.257622542056430426, -24.31502561551697283, 16.87380292611441845 ) ) ;
#10612=CARTESIAN_POINT ( 'NONE',  ( -4.723668461522841053E-14, 28.28960257232502684, 20.99999999999998934 ) ) ;
#10620=CARTESIAN_POINT ( 'NONE',  ( 16.81914744106122228, 21.75867863382669753, 16.30093088679352320 ) ) ;
#10629=CARTESIAN_POINT ( 'NONE',  ( -30.53792857583819398, -5.895195796384474107, 19.27171037444156809 ) ) ;
#10656=CARTESIAN_POINT ( 'NONE',  ( 22.56822310031678214, -21.59793901597642574, 19.99202127657133232 ) ) ;
#10679=CARTESIAN_POINT ( 'NONE',  ( -25.15015781185978483, -9.899056496887835621, 20.99999999999989697 ) ) ;
#10689=CARTESIAN_POINT ( 'NONE',  ( -20.78373334066888845, -29.14101728923843027, 12.14047268033097460 ) ) ;
#10702=CARTESIAN_POINT ( 'NONE',  ( -13.32438941869583005, 7.692839817671220715, 20.94377226548378346 ) ) ;
#10709=CARTESIAN_POINT ( 'NONE',  ( 36.04785107591603577, -18.56329043283703584, 11.55979286843940557 ) ) ;
#10712=DIRECTION ( 'NONE',  ( 1.000000000000000000, 0.000000000000000000, -0.000000000000000000 ) ) ;
#10750=CARTESIAN_POINT ( 'NONE',  ( -14.48927117870122316, -30.61587158504648087, 3.000000000000000000 ) ) ;
#10760=CARTESIAN_POINT ( 'NONE',  ( -17.28285333400955182, 27.30382183500235271, 12.14047268033097460 ) ) ;
#10764=CARTESIAN_POINT ( 'NONE',  ( -1.485997264023686038, 36.23016441347868977, 18.42518152272108622 ) ) ;
#10767=DIRECTION ( 'NONE',  ( 0.000000000000000000, 0.000000000000000000, 1.000000000000000000 ) ) ;
#10779=CARTESIAN_POINT ( 'NONE',  ( 15.74227866053861824, -25.75916161678321004, 17.42190598798392998 ) ) ;
#10786=CARTESIAN_POINT ( 'NONE',  ( -33.34742602403127165, -19.25314539175551332, 16.30093088680190760 ) ) ;
#10802=UNCERTAINTY_MEASURE_WITH_UNIT (LENGTH_MEASURE( 1.000000000000000082E-05 ), #25494, 'distance_accuracy_value', 'NONE');
#10810=CARTESIAN_POINT ( 'NONE',  ( 31.99827245170146739, -22.69195664478511887, 15.13084544680246246 ) ) ;
#10812=CARTESIAN_POINT ( 'NONE',  ( -3.468257360957398561, 38.22173125672347282, 16.30093088680195379 ) ) ;
#10813=CARTESIAN_POINT ( 'NONE',  ( 4.310286166645415044E-14, -23.76115801358234947, 17.42190598798392998 ) ) ;
#10815=CARTESIAN_POINT ( 'NONE',  ( 6.337050370968067448, 27.87972302178011930, 20.69868183039781329 ) ) ;
#10822=CARTESIAN_POINT ( 'NONE',  ( 13.31403195191067290, 20.45929608435098501, 19.27171037444031043 ) ) ;
#10832=CARTESIAN_POINT ( 'NONE',  ( -30.92601969764245595, -9.797982979854426233, 19.66345542862527651 ) ) ;
#10847=CARTESIAN_POINT ( 'NONE',  ( 24.51396478725026640, -11.15767879383072447, 23.00000000000000000 ) ) ;
#10859=CARTESIAN_POINT ( 'NONE',  ( 17.70478766477712185, -23.47393717365348209, 19.27171037444127677 ) ) ;
#10888=CARTESIAN_POINT ( 'NONE',  ( -25.16128423893358601, -12.39270898182848768, 20.99999999999999645 ) ) ;
#10898=CARTESIAN_POINT ( 'NONE',  ( -24.65531199400790996, -28.60128534115777654, 11.55979286843934695 ) ) ;
#10904=CARTESIAN_POINT ( 'NONE',  ( -4.331888841169210913, 42.14502281828541186, 11.00000000000000178 ) ) ;
#10912=CARTESIAN_POINT ( 'NONE',  ( -18.38177052347168683, 3.916595739930567532, 20.50957957746028271 ) ) ;
#10915=CARTESIAN_POINT ( 'NONE',  ( 23.31768133719840463, -16.68166585059941198, 20.94377226548368398 ) ) ;
#10920=CARTESIAN_POINT ( 'NONE',  ( 22.73075399258389595, -29.06185307675081830, 11.55979286843892595 ) ) ;
#10945=CARTESIAN_POINT ( 'NONE',  ( -22.38145423153888558, -15.36249082013412171, 23.00000000000000000 ) ) ;
#10971=CARTESIAN_POINT ( 'NONE',  ( 7.449887436097998084, 34.87105630051927108, 17.92354375535251521 ) ) ;
#10972=CARTESIAN_POINT ( 'NONE',  ( -14.98890121934603314, -28.67928442654204346, 11.00000000000000000 ) ) ;
#10973=VERTEX_POINT ( 'NONE', #32646 ) ;
#10990=CARTESIAN_POINT ( 'NONE',  ( -27.50471383176088480, -25.75100844545737644, 15.72805884748907879 ) ) ;
#11007=CARTESIAN_POINT ( 'NONE',  ( -16.31185170147123387, -29.02059919786648479, 10.99999999999952038 ) ) ;
#11013=CARTESIAN_POINT ( 'NONE',  ( 15.20016916874550539, -27.86040092368493504, 14.53008259254011136 ) ) ;
#11016=CARTESIAN_POINT ( 'NONE',  ( -1.415557151730355161E-13, 39.95159812444026670, 13.92931973827808712 ) ) ;
#11018=CARTESIAN_POINT ( 'NONE',  ( -15.60391421429489434, -26.29546805948952581, 16.87380292611441490 ) ) ;
#11020=CARTESIAN_POINT ( 'NONE',  ( -5.702281711626214999, 27.34093017838354456, 20.82122704794079127 ) ) ;
#11029=CARTESIAN_POINT ( 'NONE',  ( 14.97058623676333866, 26.66112013783126500, 16.87380292611441845 ) ) ;
#11039=CARTESIAN_POINT ( 'NONE',  ( -25.71034552362591796, -20.07240169439133481, 19.99202127657103389 ) ) ;
#11063=CARTESIAN_POINT ( 'NONE',  ( 31.47522604700277071, -16.54376571344620217, 18.87996532025784546 ) ) ;
#11077=DIRECTION ( 'NONE',  ( -1.000000000000000000, 0.000000000000000000, 0.000000000000000000 ) ) ;
#11087=CARTESIAN_POINT ( 'NONE',  ( -20.52988490949636713, -16.97904854937761243, 20.99999999999995026 ) ) ;
#11097=CARTESIAN_POINT ( 'NONE',  ( -35.99085602461024536, -18.53811353976085030, 12.14047268033095150 ) ) ;
#11109=CARTESIAN_POINT ( 'NONE',  ( -24.20198940123769304, -6.620595927252167279, 20.94377226548378346 ) ) ;
#11110=CARTESIAN_POINT ( 'NONE',  ( 24.05659981020950866, -7.641904207658117620, 21.00000000000024514 ) ) ;
#11111=CARTESIAN_POINT ( 'NONE',  ( 20.38753357181586878, -16.19769905861743808, 20.99999999999998934 ) ) ;
#11114=EDGE_CURVE ( 'NONE', #39423, #25190, #8300, .T. ) ;
#11166=CARTESIAN_POINT ( 'NONE',  ( 4.383143208095032328, 35.51174355874288580, 18.42518152272108978 ) ) ;
#11169=SURFACE_STYLE_USAGE ( .BOTH. , #36153 ) ;
#11172=CARTESIAN_POINT ( 'NONE',  ( 1.078807199784882265, 27.41272755941693617, 23.00000000000000355 ) ) ;
#11185=CARTESIAN_POINT ( 'NONE',  ( -34.11404923485120122, -2.099951938866391199, 14.53008259253964951 ) ) ;
#11205=B_SPLINE_CURVE_WITH_KNOTS ( 'NONE', 3,
 ( #14940, #15331, #23880, #17998, #5790, #2551 ),
 .UNSPECIFIED., .F., .F.,
 ( 4, 2, 4 ),
 ( 0.000000000000000000, 0.5000000000000000000, 1.000000000000000000 ),
 .UNSPECIFIED. ) ;
#11209=CARTESIAN_POINT ( 'NONE',  ( 33.53425769460820050, -2.462485423393242279, 15.72805884748974847 ) ) ;
#11211=CARTESIAN_POINT ( 'NONE',  ( -16.52773037515743226, 27.09393310379821074, 14.53008259254011136 ) ) ;
#11213=CARTESIAN_POINT ( 'NONE',  ( 4.272934335498898793E-14, -24.78318996519343997, 16.30093088680190760 ) ) ;
#11215=CARTESIAN_POINT ( 'NONE',  ( 6.839309919355001988, 27.13928353713056651, 20.69868183039781684 ) ) ;
#11224=CARTESIAN_POINT ( 'NONE',  ( 7.205739717458053306, 18.19477196579531153, 20.99999999999999645 ) ) ;
#11234=CARTESIAN_POINT ( 'NONE',  ( -32.58967084635843037, -11.00843821516755483, 18.87996532025856666 ) ) ;
#11254=CARTESIAN_POINT ( 'NONE',  ( -39.51968005974920572, -13.07391886567259576, 22.99999999999999289 ) ) ;
#11259=CARTESIAN_POINT ( 'NONE',  ( 31.21198460772024674, -5.568619476414755631, 18.87996532025785967 ) ) ;
#11270=ADVANCED_FACE ( 'NONE', ( #33454 ), #5598, .T. ) ;
#11289=CARTESIAN_POINT ( 'NONE',  ( -24.05659981020947669, -7.641904207658729575, 20.99999999999999645 ) ) ;
#11300=CARTESIAN_POINT ( 'NONE',  ( -28.24711154207077257, -27.09388640670392689, 11.55979286843935050 ) ) ;
#11314=CARTESIAN_POINT ( 'NONE',  ( 17.62780868050626637, -18.45076755199313112, 20.82122704794080192 ) ) ;
#11318=CARTESIAN_POINT ( 'NONE',  ( 32.33143948541780333, 1.358872982501766025, 11.00000000000000000 ) ) ;
#11330=CARTESIAN_POINT ( 'NONE',  ( -14.48927117870122316, -30.61587158504648087, 11.00000000000000000 ) ) ;
#11373=ORIENTED_EDGE ( 'NONE', *, *, #21338, .T. ) ;
#11375=CARTESIAN_POINT ( 'NONE',  ( -23.05386822411323422, -7.747535282638357224, 20.99999999999999645 ) ) ;
#11376=CYLINDRICAL_SURFACE ( 'NONE', #15027, 20.00000000000002487 ) ;
#11390=CARTESIAN_POINT ( 'NONE',  ( -31.99827245169854706, -22.69195664478721142, 15.13084544680206811 ) ) ;
#11405=CARTESIAN_POINT ( 'NONE',  ( -36.71098721002695697, -16.64818343423248237, 11.00000000000018829 ) ) ;
#11412=CARTESIAN_POINT ( 'NONE',  ( 35.63595018118459734, -14.50160624002288579, 15.72805884748939853 ) ) ;
#11415=CARTESIAN_POINT ( 'NONE',  ( 9.055806345856177941, 37.53717483670233435, 13.92931973827812620 ) ) ;
#11416=CARTESIAN_POINT ( 'NONE',  ( -5.594491472541998967, -20.30912387778604966, 19.66345542862528717 ) ) ;
#11418=CARTESIAN_POINT ( 'NONE',  ( -6.337046384719310588, 27.87972889837504553, 20.69868183039780263 ) ) ;
#11422=B_SPLINE_CURVE_WITH_KNOTS ( 'NONE', 3,
 ( #34456, #11430, #33376, #26456, #2285, #29708, #27260, #1891, #30114, #36215, #20970, #14675, #17334, #27064, #14269, #5325, #11630, #17933 ),
 .UNSPECIFIED., .F., .F.,
 ( 4, 2, 2, 2, 2, 2, 2, 2, 4 ),
 ( 0.000000000000000000, 0.1250000000000001388, 0.2500000000000001665, 0.3750000000000001665, 0.5000000000000002220, 0.6250000000000002220, 0.7500000000000001110, 0.8750000000000001110, 1.000000000000000000 ),
 .UNSPECIFIED. ) ;
#11427=CARTESIAN_POINT ( 'NONE',  ( 20.38546294303163720, 5.309590202429361305, 19.66345542862513796 ) ) ;
#11430=CARTESIAN_POINT ( 'NONE',  ( -16.82090372984274396, 29.19711159930251299, 10.99999999999914913 ) ) ;
#11437=CARTESIAN_POINT ( 'NONE',  ( -30.06493440560439012, -18.98646248983845553, 18.87996532025748664 ) ) ;
#11444=CARTESIAN_POINT ( 'NONE',  ( 17.34253826607184479, 27.32041144404033162, 11.00000000000000000 ) ) ;
#11460=CARTESIAN_POINT ( 'NONE',  ( 20.42855823444378771, -24.24606183460743480, 18.87996532025784546 ) ) ;
#11467=( BOUNDED_CURVE ( )  B_SPLINE_CURVE ( 2, ( #13201, #12613, #37995 ),
 .UNSPECIFIED., .F., .F. ) 
 B_SPLINE_CURVE_WITH_KNOTS ( ( 3, 3 ),
 ( 0.000000000000000000, 1.000000000000000000 ),
 .UNSPECIFIED. ) 
 CURVE ( )  GEOMETRIC_REPRESENTATION_ITEM ( )  RATIONAL_B_SPLINE_CURVE ( ( 1.000000000000000000, 0.7071067811865474617, 1.000000000000000000 ) ) 
 REPRESENTATION_ITEM ( '' )  );
#11470=B_SPLINE_CURVE_WITH_KNOTS ( 'NONE', 3,
 ( #3659, #31495, #22143, #34543, #9958, #6694 ),
 .UNSPECIFIED., .F., .F.,
 ( 4, 2, 4 ),
 ( 0.000000000000000000, 0.5000000000000000000, 1.000000000000000000 ),
 .UNSPECIFIED. ) ;
#11475=CARTESIAN_POINT ( 'NONE',  ( -15.00309677617817883, 1.567672476163677109, 20.99999999999998934 ) ) ;
#11481=CARTESIAN_POINT ( 'NONE',  ( 14.98890121934584663, -28.67928442654197951, 11.55979286843934872 ) ) ;
#11485=CARTESIAN_POINT ( 'NONE',  ( -18.03924190088572743, -16.85603499720482645, 20.99999999999999645 ) ) ;
#11511=CARTESIAN_POINT ( 'NONE',  ( 22.30415078909558346, -16.34589999308455432, 20.99999999999995026 ) ) ;
#11514=CARTESIAN_POINT ( 'NONE',  ( 37.58754968649115824, -10.91577297561518556, 10.99999999999992006 ) ) ;
#11529=CARTESIAN_POINT ( 'NONE',  ( -6.143904198944369455, -13.77689918168226235, 23.00000000000000000 ) ) ;
#11554=CARTESIAN_POINT ( 'NONE',  ( -16.24129362380739749, 27.01431713447837524, 15.13084544680213739 ) ) ;
#11590=ADVANCED_FACE ( 'NONE', ( #10042 ), #37443, .T. ) ;
#11594=B_SPLINE_CURVE_WITH_KNOTS ( 'NONE', 3,
 ( #34480, #18841, #6627, #19035, #31427, #3594 ),
 .UNSPECIFIED., .F., .F.,
 ( 4, 2, 4 ),
 ( 0.000000000000000000, 0.5000000000000000000, 1.000000000000000000 ),
 .UNSPECIFIED. ) ;
#11612=CARTESIAN_POINT ( 'NONE',  ( 34.78305373678702495, -20.08200543817097738, 13.32518128616608877 ) ) ;
#11614=CARTESIAN_POINT ( 'NONE',  ( -9.055806345858652406, 37.53717483670035193, 13.92931973827746717 ) ) ;
#11619=CARTESIAN_POINT ( 'NONE',  ( -7.486246565637331948E-14, 31.60047892813804538, 20.50957957746028626 ) ) ;
#11628=CARTESIAN_POINT ( 'NONE',  ( 8.755436920352806851, 18.76929632773553180, 20.82122704794083390 ) ) ;
#11630=CARTESIAN_POINT ( 'NONE',  ( 16.82090372984190907, 29.19711159930552924, 10.99999999999877787 ) ) ;
#11639=CARTESIAN_POINT ( 'NONE',  ( -29.67744882842988829, -20.56940131916892867, 18.42518152272108622 ) ) ;
#11654=CARTESIAN_POINT ( 'NONE',  ( 23.09341953181399987, -31.04079623446942193, 22.99999999999999289 ) ) ;
#11663=VECTOR ( 'NONE', #31399, 1000.000000000000000 ) ;
#11664=CARTESIAN_POINT ( 'NONE',  ( 30.53792857583748699, -5.895195796383389641, 19.27171037444157875 ) ) ;
#11676=LINE ( 'NONE', #33027, #7757 ) ;
#11680=CARTESIAN_POINT ( 'NONE',  ( -14.98890121934605268, -28.67928442654203636, 11.00000000000000000 ) ) ;
#11684=CARTESIAN_POINT ( 'NONE',  ( -27.31307357281963277, -8.451814904569179276, 20.69868183039799447 ) ) ;
#11710=CARTESIAN_POINT ( 'NONE',  ( 19.25012218476983605, -17.89323886701251354, 20.94377226548378346 ) ) ;
#11722=CARTESIAN_POINT ( 'NONE',  ( 14.43694901005322961, 26.51279404187409483, 17.42190598798392998 ) ) ;
#11751=CARTESIAN_POINT ( 'NONE',  ( -17.34253826607279692, 27.32041144403692101, 11.55979286843934872 ) ) ;
#11769=FACE_OUTER_BOUND ( 'NONE', #21696, .T. ) ;
#11781=CYLINDRICAL_SURFACE ( 'NONE', #29576, 18.00000000000003553 ) ;
#11796=ORIENTED_EDGE ( 'NONE', *, *, #4163, .T. ) ;
#11806=CARTESIAN_POINT ( 'NONE',  ( 33.02831943717437468, -0.5583946152424188458, 14.53008259254167811 ) ) ;
#11808=CARTESIAN_POINT ( 'NONE',  ( -3.652674690108859146, 39.05729514278205272, 15.13084544680221200 ) ) ;
#11809=CARTESIAN_POINT ( 'NONE',  ( -5.730292628140351674, -18.69445663741131014, 20.25080042701566541 ) ) ;
#11812=CARTESIAN_POINT ( 'NONE',  ( -6.978236406932369462, 28.42397902804928833, 20.50957957746028271 ) ) ;
#11819=CARTESIAN_POINT ( 'NONE',  ( 8.768078002820624661, 24.93711404286646527, 20.50957957746029336 ) ) ;
#11830=CARTESIAN_POINT ( 'NONE',  ( -20.37435360786956551, -23.49902402743817120, 19.27171037444156809 ) ) ;
#11850=CARTESIAN_POINT ( 'NONE',  ( -39.59914439355220850, -10.88071517532349475, 11.00000000000000000 ) ) ;
#11855=CARTESIAN_POINT ( 'NONE',  ( 31.19395790416513847, -3.926110744752351778, 18.42518152272147702 ) ) ;
#11860=EDGE_CURVE ( 'NONE', #36229, #39423, #19764, .T. ) ;
#11863=CARTESIAN_POINT ( 'NONE',  ( -37.48531001978128074, -11.24999991186452775, 11.00000000000002309 ) ) ;
#11876=CARTESIAN_POINT ( 'NONE',  ( -5.096756537559850031, -26.22849730612247754, 13.92931973827808712 ) ) ;
#11879=CARTESIAN_POINT ( 'NONE',  ( -26.17801803039915498, -8.007547698858626717, 20.82122704794079837 ) ) ;
#11897=ORIENTED_EDGE ( 'NONE', *, *, #4163, .F. ) ;
#11907=CARTESIAN_POINT ( 'NONE',  ( 25.92581632124332458, -14.96827703203057958, 20.82122704794079837 ) ) ;
#11909=EDGE_CURVE ( 'NONE', #24813, #21291, #25762, .T. ) ;
#11940=COLOUR_RGB ( '', 0.66274510, 0.83137255, 0.94901961) ;
#11951=CARTESIAN_POINT ( 'NONE',  ( -25.71480618105703542, 9.014447550988780478, 11.55979286844120324 ) ) ;
#11966=PRESENTATION_STYLE_ASSIGNMENT (( #11169 ) ) ;
#11969=CARTESIAN_POINT ( 'NONE',  ( 4.444273797880263110, 24.85496137639062297, 23.00000000000000355 ) ) ;
#12006=CARTESIAN_POINT ( 'NONE',  ( -5.726446540400362828, 39.49945686212554818, 12.14047268033097104 ) ) ;
#12007=CARTESIAN_POINT ( 'NONE',  ( 4.332433290453930557E-14, -14.56650175400723946, 20.99999999999999645 ) ) ;
#12009=CARTESIAN_POINT ( 'NONE',  ( -0.9851783940330662848, 31.60047892813803827, 20.50957957746028626 ) ) ;
#12012=CARTESIAN_POINT ( 'NONE',  ( -16.24129362380271857, 27.01431713449521510, 15.13084544680213384 ) ) ;
#12029=CARTESIAN_POINT ( 'NONE',  ( -29.28423149095540978, -1.632116715642781823, 18.42518152272108978 ) ) ;
#12042=CARTESIAN_POINT ( 'NONE',  ( 18.77248997590679735, -31.35432035705766651, 11.00000000000000000 ) ) ;
#12046=CARTESIAN_POINT ( 'NONE',  ( 33.75875814100314187, 2.759858869446413010, 23.00000000000000000 ) ) ;
#12051=CARTESIAN_POINT ( 'NONE',  ( 20.52459090776396167, -25.56956579041154498, 17.92354375535250810 ) ) ;
#12059=CARTESIAN_POINT ( 'NONE',  ( -14.98890121934603314, -28.67928442654204346, 11.00000000000000000 ) ) ;
#12072=CARTESIAN_POINT ( 'NONE',  ( -10.15481549915472570, -27.08512292516926223, 13.32518128617831010 ) ) ;
#12075=CARTESIAN_POINT ( 'NONE',  ( -19.27923559247379970, -17.06979493269815151, 21.00000000000004619 ) ) ;
#12105=CARTESIAN_POINT ( 'NONE',  ( 26.64268929643274930, -15.38216383723093550, 20.69868183039781329 ) ) ;
#12108=ORIENTED_EDGE ( 'NONE', *, *, #21156, .F. ) ;
#12129=CARTESIAN_POINT ( 'NONE',  ( -14.48927117870122316, -30.61587158504648087, 11.00000000000000000 ) ) ;
#12136=CARTESIAN_POINT ( 'NONE',  ( 36.53988292926447912, -0.5802930198997262590, 11.00000000000000178 ) ) ;
#12138=CARTESIAN_POINT ( 'NONE',  ( -18.88614099607083929, -28.19481782898740718, 15.13084544680256549 ) ) ;
#12149=AXIS2_PLACEMENT_3D ( 'NONE', #38166, #10335, #22716 ) ;
#12150=CARTESIAN_POINT ( 'NONE',  ( -17.28285333401127133, 27.30382183499614612, 12.14047268033097460 ) ) ;
#12185=EDGE_LOOP ( 'NONE', ( #19982, #30143, #13749, #14442 ) ) ;
#12204=CARTESIAN_POINT ( 'NONE',  ( -7.565838454495246168, 38.87983827381766844, 12.14047268033080584 ) ) ;
#12206=CARTESIAN_POINT ( 'NONE',  ( 5.661571401657415237, -19.51153516500234630, 19.99202127657103389 ) ) ;
#12208=CARTESIAN_POINT ( 'NONE',  ( -8.883663045967775673, 28.52602195317091827, 19.99202127657103389 ) ) ;
#12228=CARTESIAN_POINT ( 'NONE',  ( -33.67754748216002270, -6.175997133552459495, 17.42190598798435630 ) ) ;
#12251=CARTESIAN_POINT ( 'NONE',  ( 18.95259542075067927, -26.31232456688672272, 17.42190598798396550 ) ) ;
#12256=FACE_OUTER_BOUND ( 'NONE', #12185, .T. ) ;
#12262=B_SPLINE_SURFACE_WITH_KNOTS ( 'NONE', 3, 3, ( 
 ( #29768, #25904, #20431, #29164, #35465, #20228, #36067, #8230, #1950, #1333, #16982, #22855, #20635, #29359, #35260, #14325, #38710, #8025, #1537, #26719, #13715, #32627, #26105, #39104, #38504 ),
 ( #13514, #11289, #13922, #35863, #4781, #10679, #17189, #23062, #26316, #10888, #16576, #23271, #14123, #35668, #29564, #28956, #1744, #38910, #1135, #26522, #11087, #37059, #12075, #40100, #11485 ),
 ( #8437, #33235, #39899, #27317, #5576, #24072, #21027, #27120, #33436, #17797, #8634, #36465, #17987, #20833, #36665, #33824, #17595, #24465, #23871, #27708, #2734, #5184, #9032, #14527, #2541 ),
 ( #5381, #2143, #30772, #11879, #15125, #18183, #5973, #30171, #21418, #30377, #33035, #12276, #14930, #29964, #39706, #2932, #36273, #24271, #8835, #27515, #9228, #26919, #36863, #39306, #21222 ),
 ( #30576, #33632, #2344, #18378, #11684, #14731, #15321, #5781, #24663, #39507, #3719, #3130, #25062, #6954, #31758, #12470, #28107, #10022, #15527, #37846, #21811, #12669, #25259, #13261, #25653 ),
 ( #15718, #3525, #3328, #285, #19361, #22400, #3921, #37655, #37258, #38049, #34018, #22013, #6368, #9431, #27910, #34214, #18773, #677, #16319, #31163, #16121, #85, #37459, #18576, #21613 ),
 ( #24862, #6175, #34411, #9633, #34803, #6562, #18969, #28704, #31356, #882, #9824, #15921, #30963, #28305, #484, #12867, #22203, #34606, #6758, #19161, #31553, #28505, #13057, #25447, #26266 ),
 ( #1693, #29112, #26667, #1284, #29517, #35619, #20384, #14069, #32779, #38863, #32575, #7776, #16932, #20178, #10220, #29316, #11039, #7571, #35413, #1086, #25854, #10424, #17140, #4530, #23011 ),
 ( #38255, #7364, #38659, #4733, #26466, #32164, #10832, #23423, #35013, #22807, #35815, #16525, #22606, #35205, #19770, #7164, #7972, #4325, #19976, #13463, #16730, #4937, #13666, #17342, #26056 ),
 ( #29718, #38455, #1899, #10629, #19563, #14276, #32374, #31952, #1486, #4120, #13875, #23223, #28908, #8786, #2885, #15277, #18138, #23624, #2495, #32984, #15076, #11830, #5136, #36416, #5529 ),
 ( #39852, #8580, #2295, #36022, #21175, #33779, #39057, #11234, #39458, #23820, #26868, #17542, #39258, #11437, #30528, #5927, #14476, #33578, #29916, #14682, #8180, #20586, #33182, #20978, #20785 ),
 ( #12029, #5333, #36225, #18328, #8389, #27465, #14883, #17745, #2096, #17940, #8984, #30122, #27071, #24418, #11639, #24022, #33385, #36812, #30323, #2687, #27270, #39657, #24219, #36616, #5730 ),
 ( #21373, #30724, #37805, #19121, #9978, #16072, #9782, #12821, #34368, #25216, #27664, #6516, #28461, #25015, #12625, #18529, #3083, #27866, #34563, #21968, #240, #18728, #15673, #21764, #28061 ),
 ( #31516, #9382, #15877, #636, #12228, #15476, #3678, #33968, #3878, #37, #12423, #40048, #37616, #37213, #37410, #30920, #24816, #22161, #34168, #6713, #6319, #13018, #25407, #34764, #31117 ),
 ( #24619, #6914, #3281, #37012, #18923, #22356, #9583, #31312, #3481, #19316, #31712, #9182, #21568, #6125, #28264, #440, #13821, #22965, #31908, #29465, #35162, #13214, #17090, #13624, #19725 ),
 ( #16479, #4076, #32729, #26216, #25814, #26010, #19518, #1040, #38608, #38213, #35567, #7318, #10786, #1643, #23377, #28863, #14025, #23169, #38407, #13420, #7524, #38008, #7119, #10381, #35772 ),
 ( #35368, #22759, #32115, #4280, #834, #19928, #10181, #32532, #29270, #22559, #10583, #32323, #4486, #16683, #16889, #4686, #26418, #10990, #16275, #28661, #29065, #1243, #1438, #34968, #7729 ),
 ( #38812, #20133, #7926, #20336, #25607, #37319, #18638, #2049, #8339, #26617, #9494, #5284, #20740, #31027, #11390, #14426, #12534, #26821, #34076, #21477, #23772, #14226, #12138, #15584, #39009 ),
 ( #39211, #30635, #11185, #3195, #33133, #37122, #33883, #36172, #18439, #29864, #32931, #39961, #6236, #18242, #15384, #2793, #15184, #24926, #24525, #40162, #27970, #27575, #12334, #21870, #24722 ),
 ( #36926, #35974, #20535, #5086, #9291, #9092, #6035, #30829, #2996, #27773, #21675, #144, #4883, #17296, #29668, #17496, #1850, #23577, #8127, #25717, #38111, #4184, #22665, #16382, #19424 ),
 ( #28769, #38313, #13322, #1145, #12729, #13121, #743, #25121, #31420, #37518, #10485, #16185, #34473, #9697, #3586, #10084, #31816, #10282, #15983, #22466, #35068, #18835, #22072, #7223, #346 ),
 ( #6620, #34275, #3982, #28364, #3782, #19028, #542, #945, #12928, #19623, #25318, #32018, #16588, #13526, #37718, #28969, #25916, #31613, #9883, #25512, #15780, #22263, #34668, #6431, #3386 ),
 ( #6820, #19223, #28568, #31222, #37912, #28170, #34871, #7021, #29178, #20241, #29574, #11097, #35476, #23480, #39114, #8239, #17604, #39316, #35270, #23282, #7632, #10689, #16790, #23074, #20037 ),
 ( #32434, #13931, #26532, #14536, #26930, #36078, #4592, #26326, #4386, #22866, #35679, #38721, #20645, #29371, #16993, #29974, #1548, #11300, #38921, #10898, #32224, #1754, #33044, #1343, #7425 ),
 ( #7833, #14336, #19834, #32638, #17199, #4792, #5195, #38514, #26729, #14134, #13727, #35876, #1961, #8035, #2153, #20442, #32839, #4994, #23680, #17405, #29779, #26118, #36283, #27130, #2943 ) ),
 .UNSPECIFIED., .F., .F., .F.,
 ( 4, 3, 3, 3, 3, 3, 3, 3, 4 ),
 ( 4, 3, 3, 3, 3, 3, 3, 3, 4 ),
 ( 0.000000000000000000, 0.1250000000000000000, 0.2500000000000000000, 0.3750000000000000000, 0.5000000000000000000, 0.6250000000000000000, 0.7500000000000000000, 0.8750000000000000000, 1.000000000000000000 ),
 ( 2.365504664328351048, 2.690426355543287240, 3.015348046758223433, 3.340269737973159181, 3.665191429188095373, 3.990113120403031566, 4.315034811617967314, 4.639956502832903951, 4.964878194047839699 ),
 .UNSPECIFIED. ) ;
#12265=CARTESIAN_POINT ( 'NONE',  ( 17.01882136417861702, 27.23043334312144736, 13.32518128616608877 ) ) ;
#12276=CARTESIAN_POINT ( 'NONE',  ( -26.32839453010153719, -14.27099112026725081, 20.82122704794093693 ) ) ;
#12294=EDGE_CURVE ( 'NONE', #27076, #6337, #31038, .T. ) ;
#12303=CARTESIAN_POINT ( 'NONE',  ( 26.61692196988907355, -13.50708991729936592, 20.82122704794081258 ) ) ;
#12308=CARTESIAN_POINT ( 'NONE',  ( 14.48927117870123027, -30.61587158504688233, 11.00000000000000000 ) ) ;
#12311=CARTESIAN_POINT ( 'NONE',  ( -8.859192577249674017, 12.20922670551869516, 23.00000000000000000 ) ) ;
#12334=CARTESIAN_POINT ( 'NONE',  ( -18.87560410041185222, -28.49365963342004804, 14.53008259254054124 ) ) ;
#12344=CARTESIAN_POINT ( 'NONE',  ( -25.71480618105494642, 9.014447550991281588, 11.00000000000190603 ) ) ;
#12351=EDGE_LOOP ( 'NONE', ( #24394, #13812, #15354, #23006, #34029, #11796 ) ) ;
#12357=AXIS2_PLACEMENT_3D ( 'NONE', #15408, #1572, #20062 ) ;
#12372=CARTESIAN_POINT ( 'NONE',  ( -4.672335726382881305, 24.36080358023109227, 23.00000000000000000 ) ) ;
#12387=ADVANCED_FACE ( 'NONE', ( #18893 ), #2656, .F. ) ;
#12388=AXIS2_PLACEMENT_3D ( 'NONE', #16263, #6308, #19302 ) ;
#12400=CARTESIAN_POINT ( 'NONE',  ( 12.30427675147600297, 35.50736440027970531, 12.73282698324849171 ) ) ;
#12402=CARTESIAN_POINT ( 'NONE',  ( -18.23649648353769948, -16.09146789626166196, 20.99999999999999645 ) ) ;
#12405=CARTESIAN_POINT ( 'NONE',  ( -8.810143528080892850, 27.17887818198020611, 20.25080042701568317 ) ) ;
#12410=CARTESIAN_POINT ( 'NONE',  ( -17.34253826607193361, 27.32041144404004740, 11.55979286843935050 ) ) ;
#12423=CARTESIAN_POINT ( 'NONE',  ( -33.85500357264719185, -15.79720895789074575, 17.42190598798393708 ) ) ;
#12448=CARTESIAN_POINT ( 'NONE',  ( 23.05386822411318803, -7.747535282638377652, 20.99999999999999645 ) ) ;
#12449=CARTESIAN_POINT ( 'NONE',  ( 15.89892447185075497, -25.15199583021637508, 17.92354375535250810 ) ) ;
#12453=FACE_OUTER_BOUND ( 'NONE', #38291, .T. ) ;
#12459=CARTESIAN_POINT ( 'NONE',  ( 18.37899676820244110, 22.33688965558069128, 13.32518128614809605 ) ) ;
#12470=CARTESIAN_POINT ( 'NONE',  ( -24.94906875546841363, -17.45075080782938315, 20.69868183039781329 ) ) ;
#12473=EDGE_LOOP ( 'NONE', ( #2453, #12108, #30792, #26198 ) ) ;
#12498=CARTESIAN_POINT ( 'NONE',  ( 27.58732789242641203, -12.88115193908554978, 20.69868183039782394 ) ) ;
#12511=EDGE_CURVE ( 'NONE', #32321, #22892, #25688, .T. ) ;
#12531=CARTESIAN_POINT ( 'NONE',  ( -23.05386822411323422, -7.747535282638357224, 23.00000000000000000 ) ) ;
#12534=CARTESIAN_POINT ( 'NONE',  ( -29.26100170765952058, -25.10377279865925004, 15.13084544680221377 ) ) ;
#12545=CARTESIAN_POINT ( 'NONE',  ( -12.55429062395547035, 25.98950339718248870, 18.87996532025784902 ) ) ;
#12551=CARTESIAN_POINT ( 'NONE',  ( 36.01432606574135065, -5.340291233615181987, 13.92931973827784908 ) ) ;
#12571=CARTESIAN_POINT ( 'NONE',  ( 17.76739295965371923, 31.93461338995193799, 23.00000000000000711 ) ) ;
#12604=CARTESIAN_POINT ( 'NONE',  ( 15.93457153376149193, 30.96347702964845539, 12.14047268033087690 ) ) ;
#12607=CARTESIAN_POINT ( 'NONE',  ( 10.03134041160893375, 26.49437744576689724, 19.99202127657225603 ) ) ;
#12613=CARTESIAN_POINT ( 'NONE',  ( 19.26948696230200397, 27.85601271560037162, 23.00000000000000355 ) ) ;
#12625=CARTESIAN_POINT ( 'NONE',  ( -30.14286744058730250, -20.99504498967513300, 17.92354375535250099 ) ) ;
#12639=CARTESIAN_POINT ( 'NONE',  ( 16.58691282011809420, -31.15705289669448064, 11.00000000000000000 ) ) ;
#12650=CARTESIAN_POINT ( 'NONE',  ( 15.60391421430543524, -26.29546805949240351, 16.87380292611441490 ) ) ;
#12655=CARTESIAN_POINT ( 'NONE',  ( 4.137850160811998634, 25.30681243524901447, 21.00000000000000355 ) ) ;
#12660=CARTESIAN_POINT ( 'NONE',  ( 22.45707936798469717, 12.96560081831818501, 14.53008259254011136 ) ) ;
#12669=CARTESIAN_POINT ( 'NONE',  ( -20.08365402398563759, -19.49265790308138335, 20.69868183039781329 ) ) ;
#12694=CARTESIAN_POINT ( 'NONE',  ( 28.40703083259912987, -13.04618529600540811, 20.50957957746029336 ) ) ;
#12729=CARTESIAN_POINT ( 'NONE',  ( -36.21547910512273916, -5.268304678878102720, 13.32518128616653286 ) ) ;
#12737=CARTESIAN_POINT ( 'NONE',  ( -21.00262217608306869, 5.738642561619127669, 19.27171037444162494 ) ) ;
#12745=CARTESIAN_POINT ( 'NONE',  ( 31.16314261583367085, -24.50336240592831416, 13.32518128616608344 ) ) ;
#12752=CARTESIAN_POINT ( 'NONE',  ( 22.48079666814421884, 18.61591633950141755, 22.99999999999999645 ) ) ;
#12753=B_SPLINE_CURVE_WITH_KNOTS ( 'NONE', 3,
 ( #36052, #2719, #15109, #21403, #5364, #5561, #27497, #33016, #21010, #23852, #39690, #26899, #20617, #9014, #30357, #33611, #36648, #12059 ),
 .UNSPECIFIED., .F., .F.,
 ( 4, 2, 2, 2, 2, 2, 2, 2, 4 ),
 ( 0.000000000000000000, 0.1250000000000000000, 0.2500000000000000000, 0.3750000000000000000, 0.5000000000000000000, 0.6250000000000000000, 0.7500000000000000000, 0.8750000000000000000, 1.000000000000000000 ),
 .UNSPECIFIED. ) ;
#12758=CARTESIAN_POINT ( 'NONE',  ( -19.48557158514998022, -11.24999999999982414, 3.000000000000000000 ) ) ;
#12760=SHAPE_REPRESENTATION ( 'Protective Travel Cap', ( #24238 ), #31997 ) ;
#12781=VERTEX_POINT ( 'NONE', #10750 ) ;
#12799=CARTESIAN_POINT ( 'NONE',  ( -5.638963013753754971, 39.23975437003352340, 13.32518128616608521 ) ) ;
#12802=CARTESIAN_POINT ( 'NONE',  ( -5.180310612586867869, 33.71427074068270002, 19.27171037444158586 ) ) ;
#12821=CARTESIAN_POINT ( 'NONE',  ( -33.92416433109639229, -10.98373637526240643, 17.92354375535328614 ) ) ;
#12848=CARTESIAN_POINT ( 'NONE',  ( 30.57450045107875169, -0.3656520783190762014, 16.87380292611442201 ) ) ;
#12851=CARTESIAN_POINT ( 'NONE',  ( -3.025308588020407363, 26.48089285804710613, 20.99999999999998934 ) ) ;
#12858=CARTESIAN_POINT ( 'NONE',  ( 23.18947492591157555, 13.38844959084118358, 11.00000000000000000 ) ) ;
#12867=CARTESIAN_POINT ( 'NONE',  ( -26.04200899061306274, -18.69117426458536357, 20.25080042701566541 ) ) ;
#12894=CARTESIAN_POINT ( 'NONE',  ( 19.10350568547219297, -22.04057959011761625, 19.99202127657101968 ) ) ;
#12928=CARTESIAN_POINT ( 'NONE',  ( -37.31659891191868184, -12.87518290988868586, 12.73282698324829809 ) ) ;
#12935=CARTESIAN_POINT ( 'NONE',  ( -11.88159808435120013, 30.55960002361344507, 17.92354375535250810 ) ) ;
#12938=CARTESIAN_POINT ( 'NONE',  ( -18.88552629894566692, 10.90356369248249280, 18.87996532025784546 ) ) ;
#12940=CARTESIAN_POINT ( 'NONE',  ( 23.98526753813946044, -9.069922861307770035, 20.99999999999999645 ) ) ;
#12941=CARTESIAN_POINT ( 'NONE',  ( 24.37710423125464487, -10.07883586999013303, 23.00000000000000000 ) ) ;
#12945=CARTESIAN_POINT ( 'NONE',  ( 18.86510067431754933, -28.79249900932126849, 13.92931973827835002 ) ) ;
#12951=DIRECTION ( 'NONE',  ( -0.000000000000000000, -0.000000000000000000, -1.000000000000000000 ) ) ;
#12964=CARTESIAN_POINT ( 'NONE',  ( -10.37659644360395106, 39.73422260060542754, 11.00000000000000000 ) ) ;
#12996=CARTESIAN_POINT ( 'NONE',  ( -9.340438144419737299, 38.00965938231843211, 10.99999999999993605 ) ) ;
#12997=EDGE_CURVE ( 'NONE', #24869, #39423, #17010, .T. ) ;
#13000=CARTESIAN_POINT ( 'NONE',  ( 1.410291641398409679, 35.53022820328503428, 18.87996532025784546 ) ) ;
#13018=CARTESIAN_POINT ( 'NONE',  ( -20.56996978659371678, -26.19496882840758545, 17.42190598798392998 ) ) ;
#13040=CARTESIAN_POINT ( 'NONE',  ( 34.20211996652216868, -5.988425181405260034, 16.87380292611403121 ) ) ;
#13043=CARTESIAN_POINT ( 'NONE',  ( -2.442402655125509359, 27.78651631404546052, 20.99999999999999645 ) ) ;
#13057=CARTESIAN_POINT ( 'NONE',  ( -19.13252718791541440, -21.21924719729587139, 20.25080042701590699 ) ) ;
#13080=ORIENTED_EDGE ( 'NONE', *, *, #21156, .T. ) ;
#13085=CARTESIAN_POINT ( 'NONE',  ( 27.94267071599651686, -5.959630984681780319, 20.25080042701592831 ) ) ;
#13121=CARTESIAN_POINT ( 'NONE',  ( -36.76835206499502107, -7.129807841006686964, 13.32518128616540665 ) ) ;
#13128=CARTESIAN_POINT ( 'NONE',  ( -9.066401385854234718, 34.43014579340745485, 17.42190598798393353 ) ) ;
#13132=CARTESIAN_POINT ( 'NONE',  ( -23.22986302875264641, 7.287013008511430634, 17.42190598798427459 ) ) ;
#13141=CARTESIAN_POINT ( 'NONE',  ( 22.71959475104719317, -29.00055231699513669, 12.14047268033058025 ) ) ;
#13182=CARTESIAN_POINT ( 'NONE',  ( -27.14644468510207886, -3.730463242937111179, 19.99202127657103745 ) ) ;
#13183=ORIENTED_EDGE ( 'NONE', *, *, #4049, .F. ) ;
#13191=PRODUCT_CONTEXT ( 'NONE', #15056, 'mechanical' ) ;
#13192=CARTESIAN_POINT ( 'NONE',  ( 13.80292604922466460, 34.21633694312856733, 11.55979286843946774 ) ) ;
#13195=CARTESIAN_POINT ( 'NONE',  ( 9.006936242053848574, 32.02107499576887761, 18.87996532025784546 ) ) ;
#13201=CARTESIAN_POINT ( 'NONE',  ( 19.26948696230199687, 27.85601271560034675, 11.00000000000000000 ) ) ;
#13214=CARTESIAN_POINT ( 'NONE',  ( -20.61005271883044543, -26.74738414229389249, 16.87380292611441490 ) ) ;
#13234=CARTESIAN_POINT ( 'NONE',  ( -36.77472485986697137, -21.41827268707265830, 10.99999999999999645 ) ) ;
#13237=AXIS2_PLACEMENT_3D ( 'NONE', #18807, #31195, #9466 ) ;
#13239=CARTESIAN_POINT ( 'NONE',  ( 33.13500937546621117, -2.712167277691212242, 16.30093088680227709 ) ) ;
#13242=CARTESIAN_POINT ( 'NONE',  ( 8.305703523983371639, 36.29191545080498571, 16.30093088680192537 ) ) ;
#13245=CARTESIAN_POINT ( 'NONE',  ( -4.439344921102643227, 26.26892614308282603, 20.99999999999999645 ) ) ;
#13252=CARTESIAN_POINT ( 'NONE',  ( 17.92566989745171568, 16.47414500506706503, 17.42190598798409695 ) ) ;
#13261=CARTESIAN_POINT ( 'NONE',  ( -18.28744585352635355, -19.47582948098888522, 20.69868183039782394 ) ) ;
#13280=CARTESIAN_POINT ( 'NONE',  ( -21.91981567634960371, -15.65087685632114045, 23.00000000000000000 ) ) ;
#13285=CARTESIAN_POINT ( 'NONE',  ( 24.31339772227982365, -19.97941014234455537, 20.25080042701539185 ) ) ;
#13315=ORIENTED_EDGE ( 'NONE', *, *, #20103, .F. ) ;
#13322=CARTESIAN_POINT ( 'NONE',  ( -34.54873536671436085, -1.828132805472219680, 13.32518128616564468 ) ) ;
#13332=CARTESIAN_POINT ( 'NONE',  ( 8.062736477016214209, 35.88854577675294166, 16.87380292611443267 ) ) ;
#13335=CARTESIAN_POINT ( 'NONE',  ( -16.78686424248105524, 15.93842542257001327, 18.42518152272092991 ) ) ;
#13337=CARTESIAN_POINT ( 'NONE',  ( 22.38472516250422473, -15.35952186208517745, 20.99999999999999645 ) ) ;
#13343=CARTESIAN_POINT ( 'NONE',  ( 37.07075634848848011, -14.79048025366225083, 12.14047268033097460 ) ) ;
#13359=EDGE_CURVE ( 'NONE', #18163, #38528, #4874, .T. ) ;
#13398=CARTESIAN_POINT ( 'NONE',  ( -5.746222359017751025, 39.55816310746048003, 11.55979286843935228 ) ) ;
#13401=CARTESIAN_POINT ( 'NONE',  ( -10.77668768651903619, 26.79111211459810349, 19.66345542862499940 ) ) ;
#13416=CARTESIAN_POINT ( 'NONE',  ( 14.98890121934609532, -28.67928442654220333, 11.00000000000000000 ) ) ;
#13420=CARTESIAN_POINT ( 'NONE',  ( -24.08250333997145631, -26.67951267123966375, 16.30093088680225222 ) ) ;
#13442=CARTESIAN_POINT ( 'NONE',  ( 32.26342856634837375, -3.257244833652103377, 17.42190598798432077 ) ) ;
#13445=CARTESIAN_POINT ( 'NONE',  ( 13.95035364761274543, 31.96289125330678615, 15.13084544680214627 ) ) ;
#13448=CARTESIAN_POINT ( 'NONE',  ( -5.143258252870523073, 25.23120525497748545, 20.99999999999999645 ) ) ;
#13453=CARTESIAN_POINT ( 'NONE',  ( 23.68624114772789824, 7.604278122844164045, 16.87380292611428700 ) ) ;
#13463=CARTESIAN_POINT ( 'NONE',  ( -22.79731396823270018, -22.36677566318123311, 19.66345542862559981 ) ) ;
#13485=CARTESIAN_POINT ( 'NONE',  ( -24.28032989564857047, -12.76774640304084052, 23.00000000000000000 ) ) ;
#13489=CARTESIAN_POINT ( 'NONE',  ( 29.47277113412613758, -17.01611234805177730, 19.66345542862528362 ) ) ;
#13498=DIRECTION ( 'NONE',  ( -0.000000000000000000, -0.000000000000000000, -1.000000000000000000 ) ) ;
#13514=CARTESIAN_POINT ( 'NONE',  ( -23.61737546510203600, -7.194424252576976819, 20.99999999999999645 ) ) ;
#13518=DIRECTION ( 'NONE',  ( -1.000000000000000000, 0.000000000000000000, 0.000000000000000000 ) ) ;
#13526=CARTESIAN_POINT ( 'NONE',  ( -33.93864557197014165, -21.81860479675889053, 12.73282698324848283 ) ) ;
#13534=CARTESIAN_POINT ( 'NONE',  ( 17.76739296776033683, 31.93461337800236777, 11.00000000000000178 ) ) ;
#13536=CARTESIAN_POINT ( 'NONE',  ( -1.325463245115554520E-13, 37.48425883190013508, 17.42190598798392642 ) ) ;
#13542=CARTESIAN_POINT ( 'NONE',  ( 23.81569860407207884, -13.75000000000005329, 20.99999999999999645 ) ) ;
#13546=CARTESIAN_POINT ( 'NONE',  ( 28.24711154207348685, -27.09388640670305648, 11.55979286843937892 ) ) ;
#13567=CARTESIAN_POINT ( 'NONE',  ( -15.33540832684330724, 35.51988609203693414, 11.00000000000000000 ) ) ;
#13599=CARTESIAN_POINT ( 'NONE',  ( -3.900486991066758780, 40.17991855517993116, 11.55979286843953169 ) ) ;
#13602=CARTESIAN_POINT ( 'NONE',  ( 5.983876423892909635, 32.43697950591679557, 19.66345542862528362 ) ) ;
#13624=CARTESIAN_POINT ( 'NONE',  ( -17.23228185427209169, -26.71557896778001862, 16.87380292611433674 ) ) ;
#13647=CARTESIAN_POINT ( 'NONE',  ( 34.65585262756915341, -3.900084976043348917, 15.13084544680213561 ) ) ;
#13650=CARTESIAN_POINT ( 'NONE',  ( 14.63453729950972537, 30.27278626593263056, 15.72805884748936300 ) ) ;
#13651=CARTESIAN_POINT ( 'NONE',  ( -5.304193131309156151, -23.76115801358234947, 17.42190598798392998 ) ) ;
#13653=CARTESIAN_POINT ( 'NONE',  ( 1.431596709943214973, 28.99142433710780864, 20.94377226548377990 ) ) ;
#13658=CARTESIAN_POINT ( 'NONE',  ( 25.49469310289003232, 2.228649397472089788, 18.42518152273312637 ) ) ;
#13666=CARTESIAN_POINT ( 'NONE',  ( -19.07515557932271832, -22.84232221370076488, 19.66345542862558915 ) ) ;
#13687=CARTESIAN_POINT ( 'NONE',  ( -24.08646667827930443, -13.28101593840485073, 23.00000000000000000 ) ) ;
#13692=CARTESIAN_POINT ( 'NONE',  ( 27.45400382858955268, -18.53605996571758752, 19.99202127657132877 ) ) ;
#13715=CARTESIAN_POINT ( 'NONE',  ( -20.38753357181593628, -16.19769905861790349, 20.99999999999999645 ) ) ;
#13727=CARTESIAN_POINT ( 'NONE',  ( -36.74707368630851789, -16.71203845619716333, 11.00000000000030553 ) ) ;
#13734=CARTESIAN_POINT ( 'NONE',  ( -17.76739296776035459, 31.93461337800233224, 11.00000000000000000 ) ) ;
#13738=CARTESIAN_POINT ( 'NONE',  ( 10.74031445979388621, 33.85370084240154398, 16.87380292611439714 ) ) ;
#13743=CARTESIAN_POINT ( 'NONE',  ( 24.28032989564876232, -12.76774640304080144, 20.99999999999999645 ) ) ;
#13747=CARTESIAN_POINT ( 'NONE',  ( 37.58754968649113692, -10.91577297561512339, 11.55979286843927234 ) ) ;
#13749=ORIENTED_EDGE ( 'NONE', *, *, #26548, .F. ) ;
#13775=CARTESIAN_POINT ( 'NONE',  ( -23.74716486098165547, -8.578626677874071405, 23.00000000000000000 ) ) ;
#13782=CARTESIAN_POINT ( 'NONE',  ( -23.74914942275198371, -8.582573258223684221, 20.99999999999999645 ) ) ;
#13799=CARTESIAN_POINT ( 'NONE',  ( -16.82090372984274396, 29.19711159930251299, 10.99999999999915090 ) ) ;
#13803=CARTESIAN_POINT ( 'NONE',  ( 5.791386747369449139, 35.03736185296642702, 18.42518152272108622 ) ) ;
#13812=ORIENTED_EDGE ( 'NONE', *, *, #17114, .T. ) ;
#13821=CARTESIAN_POINT ( 'NONE',  ( -28.49608467062484252, -24.01994641533374519, 16.87380292611445043 ) ) ;
#13824=EDGE_CURVE ( 'NONE', #28327, #23396, #22786, .T. ) ;
#13848=CARTESIAN_POINT ( 'NONE',  ( 36.20842572154669625, -9.127542156327942635, 15.13084544680213561 ) ) ;
#13851=CARTESIAN_POINT ( 'NONE',  ( -14.63455391419436324, 30.27276177228403853, 15.72805884748933103 ) ) ;
#13853=CARTESIAN_POINT ( 'NONE',  ( 5.257622542056514803, -24.31502561551697283, 16.87380292611441845 ) ) ;
#13857=CARTESIAN_POINT ( 'NONE',  ( 5.702284676859227019, 27.34092580698741060, 20.82122704794079837 ) ) ;
#13865=CARTESIAN_POINT ( 'NONE',  ( 11.83264664766892338, 25.78892025140200417, 19.27171037444156454 ) ) ;
#13875=CARTESIAN_POINT ( 'NONE',  ( -31.26284659378214670, -14.97710070420562367, 19.27171037444154322 ) ) ;
#13880=ORIENTED_EDGE ( 'NONE', *, *, #21435, .T. ) ;
#13886=DIRECTION ( 'NONE',  ( 0.000000000000000000, 0.000000000000000000, 1.000000000000000000 ) ) ;
#13901=CARTESIAN_POINT ( 'NONE',  ( 32.41210168510363587, -9.609370058583692753, 18.87996532025784191 ) ) ;
#13922=CARTESIAN_POINT ( 'NONE',  ( -24.42249458671265927, -8.161411852468820172, 20.99999999999995026 ) ) ;
#13931=CARTESIAN_POINT ( 'NONE',  ( -33.69589222704896514, -0.03122585499738908532, 11.55979286843900233 ) ) ;
#13945=CARTESIAN_POINT ( 'NONE',  ( -16.32868373051740818, 2.489249428719812585, 20.94377226548377635 ) ) ;
#13947=CARTESIAN_POINT ( 'NONE',  ( 23.79772124597061733, -17.36195373897592020, 20.82122704794065626 ) ) ;
#13951=CARTESIAN_POINT ( 'NONE',  ( 29.88800841290863630, -25.99212743943143167, 12.14047268033086624 ) ) ;
#13984=EDGE_CURVE ( 'NONE', #36229, #31697, #30068, .T. ) ;
#14007=CARTESIAN_POINT ( 'NONE',  ( 8.686999124429359398, 33.93090424204713429, 17.92354375535250810 ) ) ;
#14020=CARTESIAN_POINT ( 'NONE',  ( 16.80389827882015297, -21.64427909825937135, 19.99202127657103389 ) ) ;
#14025=CARTESIAN_POINT ( 'NONE',  ( -28.76760616114084712, -24.40467509901190724, 16.30093088680195379 ) ) ;
#14042=ORIENTED_EDGE ( 'NONE', *, *, #35746, .F. ) ;
#14047=CARTESIAN_POINT ( 'NONE',  ( 36.66879582113919867, -12.81605961719004760, 14.53008259254017709 ) ) ;
#14048=ORIENTED_EDGE ( 'NONE', *, *, #31159, .T. ) ;
#14049=CARTESIAN_POINT ( 'NONE',  ( 10.19952947927959030, 35.92118758406570578, 15.13084544680213739 ) ) ;
#14050=CARTESIAN_POINT ( 'NONE',  ( -16.41753675002347279, -23.14183271658003349, 19.27171037444156809 ) ) ;
#14053=CARTESIAN_POINT ( 'NONE',  ( 0.8947151973524753998, 30.76432767446200245, 20.69868183039781329 ) ) ;
#14060=CARTESIAN_POINT ( 'NONE',  ( 14.01880647360106380, 20.72057097093389899, 18.87996532025600871 ) ) ;
#14069=CARTESIAN_POINT ( 'NONE',  ( -30.28108141855295088, -11.05112898844792468, 19.99202127657160943 ) ) ;
#14086=CARTESIAN_POINT ( 'NONE',  ( 39.59914439355151217, -10.88071517532262256, 22.99999999999999289 ) ) ;
#14097=CARTESIAN_POINT ( 'NONE',  ( 30.77008022630325002, -17.76511410164234306, 18.87996532025784546 ) ) ;
#14123=CARTESIAN_POINT ( 'NONE',  ( -24.49951449059916442, -14.14480128616215282, 20.99999999999999645 ) ) ;
#14134=CARTESIAN_POINT ( 'NONE',  ( -37.13148535761801838, -14.80270701502662511, 11.00000000000000000 ) ) ;
#14149=CARTESIAN_POINT ( 'NONE',  ( -12.58275666885741195, 13.96078236988870280, 20.50957957746030758 ) ) ;
#14150=CARTESIAN_POINT ( 'NONE',  ( 23.78345815580435385, -15.17947280105387442, 21.00000000000004619 ) ) ;
#14153=B_SPLINE_CURVE_WITH_KNOTS ( 'NONE', 3,
 ( #7212, #9687, #37708, #9872, #16174, #6808, #19214, #32007, #31602, #10074, #22454, #133, #28559, #32828, #7621, #4173, #23671, #20026 ),
 .UNSPECIFIED., .F., .F.,
 ( 4, 2, 2, 2, 2, 2, 2, 2, 4 ),
 ( 0.000000000000000000, 0.1250000000000000833, 0.2500000000000001665, 0.3750000000000002220, 0.5000000000000003331, 0.6250000000000004441, 0.7500000000000002220, 0.8750000000000001110, 1.000000000000000000 ),
 .UNSPECIFIED. ) ;
#14208=CARTESIAN_POINT ( 'NONE',  ( 25.71480618106366833, 9.014447550976067092, 11.00000000000101785 ) ) ;
#14209=CARTESIAN_POINT ( 'NONE',  ( -12.83067079990756909, 27.60880874002097940, 18.42518152272070964 ) ) ;
#14211=ORIENTED_EDGE ( 'NONE', *, *, #26548, .T. ) ;
#14226=CARTESIAN_POINT ( 'NONE',  ( -20.70549897995557842, -28.06280627726274801, 15.13084544680213384 ) ) ;
#14251=CARTESIAN_POINT ( 'NONE',  ( 34.99622266290977279, -18.09877784578646498, 15.13084544680216048 ) ) ;
#14253=CARTESIAN_POINT ( 'NONE',  ( 10.55929393610962741, 36.39458846701859329, 13.92931973827808712 ) ) ;
#14254=CARTESIAN_POINT ( 'NONE',  ( -10.43399472912671300, -25.44514827097021836, 16.30093088680841618 ) ) ;
#14256=CARTESIAN_POINT ( 'NONE',  ( 4.499574175056302749, 28.42082499242057736, 20.82122704794079837 ) ) ;
#14259=VERTEX_POINT ( 'NONE', #32773 ) ;
#14267=CARTESIAN_POINT ( 'NONE',  ( 11.93114467671387047, 6.888449590841193348, 20.99999999999999645 ) ) ;
#14269=CARTESIAN_POINT ( 'NONE',  ( 13.80292604922475874, 34.21633694312841811, 11.00000000000012434 ) ) ;
#14276=CARTESIAN_POINT ( 'NONE',  ( -31.50169271651420644, -8.384983552476358071, 19.27171037444088597 ) ) ;
#14290=FACE_OUTER_BOUND ( 'NONE', #19139, .T. ) ;
#14295=CARTESIAN_POINT ( 'NONE',  ( -39.05366788733155659, -6.582903524761571923, 11.00000000000000000 ) ) ;
#14301=CARTESIAN_POINT ( 'NONE',  ( 31.08318648610487855, -11.03630075675846101, 19.66345542862528006 ) ) ;
#14316=LINE ( 'NONE', #29955, #34998 ) ;
#14322=CARTESIAN_POINT ( 'NONE',  ( 14.98890121934613440, -28.67928442654205057, 11.00000000000000000 ) ) ;
#14325=CARTESIAN_POINT ( 'NONE',  ( -22.79104142221948592, -15.00151558123136830, 21.00000000000000000 ) ) ;
#14336=CARTESIAN_POINT ( 'NONE',  ( -33.69589222704901488, -0.03122585499731184155, 10.99999999999963585 ) ) ;
#14352=CARTESIAN_POINT ( 'NONE',  ( -6.367390439426989346, 24.26983560721853195, 20.94377226548378346 ) ) ;
#14353=CARTESIAN_POINT ( 'NONE',  ( 24.69586183797155599, -8.725643957991929156, 20.99999999999999645 ) ) ;
#14369=CARTESIAN_POINT ( 'NONE',  ( 7.962467718761615743, 24.71319220551615814, 20.69868183039780973 ) ) ;
#14393=B_SPLINE_CURVE_WITH_KNOTS ( 'NONE', 3,
 ( #2336, #5774, #30368, #11475, #39699, #39298 ),
 .UNSPECIFIED., .F., .F.,
 ( 4, 2, 4 ),
 ( 0.000000000000000000, 0.5000000000000000000, 1.000000000000000000 ),
 .UNSPECIFIED. ) ;
#14426=CARTESIAN_POINT ( 'NONE',  ( -30.62963707967903559, -23.89786472172323073, 15.13084544680214094 ) ) ;
#14434=CIRCLE ( 'NONE', #39730, 60.00000000000006395 ) ;
#14440=CARTESIAN_POINT ( 'NONE',  ( -28.25062263172018007, -27.03061230010028382, 11.00000000000007994 ) ) ;
#14442=ORIENTED_EDGE ( 'NONE', *, *, #4509, .F. ) ;
#14447=CARTESIAN_POINT ( 'NONE',  ( 26.12394372346528471, -27.06777822797228694, 14.53008259254010959 ) ) ;
#14449=CARTESIAN_POINT ( 'NONE',  ( 11.85731412588707023, 35.03474529413809080, 14.53008259254007761 ) ) ;
#14450=CARTESIAN_POINT ( 'NONE',  ( 15.60391421431025449, -26.29546805949347998, 16.87380292611441490 ) ) ;
#14452=CARTESIAN_POINT ( 'NONE',  ( 7.531283639252310813, 27.60866748444399121, 20.50957957746029692 ) ) ;
#14465=CARTESIAN_POINT ( 'NONE',  ( 10.34254640627884214, 25.37474234121230054, 19.99202127657103389 ) ) ;
#14476=CARTESIAN_POINT ( 'NONE',  ( -27.04163063101245612, -21.95895612274718900, 18.87996532025785257 ) ) ;
#14483=CARTESIAN_POINT ( 'NONE',  ( -19.26948696230207858, 27.85601271560029701, 11.00000000000000000 ) ) ;
#14495=CARTESIAN_POINT ( 'NONE',  ( -23.09341953181405671, -31.04079623447176317, 11.00000000000000000 ) ) ;
#14501=CARTESIAN_POINT ( 'NONE',  ( 28.59012753013995223, -4.062670752121350759, 19.66345542862688944 ) ) ;
#14522=CARTESIAN_POINT ( 'NONE',  ( 5.096756537559935296, -26.22849730612247754, 13.92931973827808712 ) ) ;
#14527=CARTESIAN_POINT ( 'NONE',  ( -18.52756972024271320, -17.82802275548162285, 20.94377226548378701 ) ) ;
#14530=ORIENTED_EDGE ( 'NONE', *, *, #11860, .F. ) ;
#14536=CARTESIAN_POINT ( 'NONE',  ( -35.68447701591266963, -3.401722300707785251, 11.55979286843934872 ) ) ;
#14553=CARTESIAN_POINT ( 'NONE',  ( 22.84262768307193170, -16.00844090263227315, 20.99999999999995026 ) ) ;
#14558=CARTESIAN_POINT ( 'NONE',  ( 18.84567888139550718, -29.34375185562582899, 11.00000000000044231 ) ) ;
#14588=CARTESIAN_POINT ( 'NONE',  ( 33.75875814100317029, 2.759858869446390361, 11.00000000000000000 ) ) ;
#14600=CARTESIAN_POINT ( 'NONE',  ( -22.71454497019444574, 13.11424865306021914, 13.92931973827808889 ) ) ;
#14656=CARTESIAN_POINT ( 'NONE',  ( 24.55877074690983619, -28.27742302307296995, 13.32518128616626107 ) ) ;
#14658=CARTESIAN_POINT ( 'NONE',  ( -12.92634929828533075, 33.47249571006609870, 15.13084544680222976 ) ) ;
#14659=CARTESIAN_POINT ( 'NONE',  ( -16.80389827881347031, -21.64427909825749197, 19.99202127657103389 ) ) ;
#14661=CARTESIAN_POINT ( 'NONE',  ( 1.971557875515494329, 31.43880600153373095, 20.50957957746028271 ) ) ;
#14672=CARTESIAN_POINT ( 'NONE',  ( 19.36000459721918787, -2.857032334477533908, 21.00000000000168399 ) ) ;
#14675=CARTESIAN_POINT ( 'NONE',  ( 7.591957726969091880, 38.93640765974098628, 10.99999999999980282 ) ) ;
#14682=CARTESIAN_POINT ( 'NONE',  ( -23.22759628179758096, -23.81077309376850337, 18.87996532025820429 ) ) ;
#14695=CARTESIAN_POINT ( 'NONE',  ( 23.74914942275252727, -8.582573258223957779, 23.00000000000000000 ) ) ;
#14707=CARTESIAN_POINT ( 'NONE',  ( 27.71565130972682311, -3.171757977843712162, 19.66345542862529072 ) ) ;
#14727=CARTESIAN_POINT ( 'NONE',  ( 4.242543333974329262E-14, -25.63390596715193936, 15.13084544680213739 ) ) ;
#14731=CARTESIAN_POINT ( 'NONE',  ( -27.57147631791836062, -9.321847555863021384, 20.69868183039745091 ) ) ;
#14744=CARTESIAN_POINT ( 'NONE',  ( -23.05386822411323422, -7.747535282638357224, 20.99999999999999645 ) ) ;
#14757=CARTESIAN_POINT ( 'NONE',  ( 23.85459647502799285, -16.20858856896905209, 20.94377226548378346 ) ) ;
#14777=CARTESIAN_POINT ( 'NONE',  ( 14.48927117870126757, -30.61587158504672246, 22.99999999999999645 ) ) ;
#14780=ORIENTED_EDGE ( 'NONE', *, *, #27135, .F. ) ;
#14783=CARTESIAN_POINT ( 'NONE',  ( 14.48927117870123027, -30.61587158504688233, 11.00000000000000000 ) ) ;
#14801=CARTESIAN_POINT ( 'NONE',  ( -24.45776404695687489, 8.140618660888312874, 15.72805884749016414 ) ) ;
#14857=CARTESIAN_POINT ( 'NONE',  ( 28.08361064019556963, -26.79812557672064344, 13.32518128616591113 ) ) ;
#14859=CARTESIAN_POINT ( 'NONE',  ( -7.360725290689154932, 38.43561981343043499, 13.92931973827797165 ) ) ;
#14860=CARTESIAN_POINT ( 'NONE',  ( 17.42101839920520590, -19.25229542401946148, 20.69868183039781329 ) ) ;
#14862=CARTESIAN_POINT ( 'NONE',  ( 9.555312204552503630, 25.15592819202958808, 20.25080042701566541 ) ) ;
#14865=CARTESIAN_POINT ( 'NONE',  ( -12.55429062395158901, 25.98950339719647573, 18.87996532025784191 ) ) ;
#14873=CARTESIAN_POINT ( 'NONE',  ( 9.534329713526908279, 19.05805734587007549, 20.69868183039784881 ) ) ;
#14883=CARTESIAN_POINT ( 'NONE',  ( -33.10646761238943014, -9.521241417581261857, 18.42518152272108978 ) ) ;
#14908=CARTESIAN_POINT ( 'NONE',  ( 29.67744882843222243, -20.56940131916748626, 18.42518152272146637 ) ) ;
#14926=CARTESIAN_POINT ( 'NONE',  ( -5.121747905603520223, -25.93120163663720845, 14.53008259254011136 ) ) ;
#14930=CARTESIAN_POINT ( 'NONE',  ( -25.92581632124343471, -14.96827703203019766, 20.82122704794079482 ) ) ;
#14940=CARTESIAN_POINT ( 'NONE',  ( -33.75875814100324845, 2.759858869446484064, 11.00000000000000000 ) ) ;
#14948=DIRECTION ( 'NONE',  ( -0.000000000000000000, -0.000000000000000000, -1.000000000000000000 ) ) ;
#14955=CARTESIAN_POINT ( 'NONE',  ( 27.24589233318962656, -6.395442063035704727, 20.50957957746052429 ) ) ;
#14957=CARTESIAN_POINT ( 'NONE',  ( 26.45121176803954910, -27.84758587393107021, 10.99999999999999822 ) ) ;
#14970=SURFACE_STYLE_FILL_AREA ( #2587 ) ;
#14982=CARTESIAN_POINT ( 'NONE',  ( 25.98021325959672723, -4.875178728621328617, 20.50957957746028981 ) ) ;
#14986=CARTESIAN_POINT ( 'NONE',  ( 29.22254796326513926, -28.85350741969417854, 11.00000000000000000 ) ) ;
#14995=CARTESIAN_POINT ( 'NONE',  ( -22.89849980942928553, 13.22045502901142200, 13.32518128616608699 ) ) ;
#14998=ADVANCED_FACE ( 'NONE', ( #8736 ), #11781, .F. ) ;
#15027=AXIS2_PLACEMENT_3D ( 'NONE', #8722, #2232, #18272 ) ;
#15042=DIRECTION ( 'NONE',  ( -1.000000000000000000, 0.000000000000000000, 0.000000000000000000 ) ) ;
#15049=CARTESIAN_POINT ( 'NONE',  ( 34.92340065173399921, -3.770459477547956517, 14.53008259254010959 ) ) ;
#15051=CARTESIAN_POINT ( 'NONE',  ( 1.856244906471662182, 39.65430245495501538, 14.53008259254011314 ) ) ;
#15052=CARTESIAN_POINT ( 'NONE',  ( 17.00801676780080385, -20.85310720624926262, 20.25080042701566541 ) ) ;
#15055=CARTESIAN_POINT ( 'NONE',  ( 2.325696902088659090, 33.04389473401325006, 19.99202127657102679 ) ) ;
#15056=APPLICATION_CONTEXT ( 'automotive_design' ) ;
#15065=CARTESIAN_POINT ( 'NONE',  ( 14.06669941890381104, 14.65883224166404730, 19.99202127657115469 ) ) ;
#15076=CARTESIAN_POINT ( 'NONE',  ( -21.70015648973560118, -23.40282454538633772, 19.27171037444124480 ) ) ;
#15093=CARTESIAN_POINT ( 'NONE',  ( -38.66460482714451530, -17.32098561216439947, 11.00000000000000000 ) ) ;
#15102=CARTESIAN_POINT ( 'NONE',  ( 32.48981136421910776, -6.600762235922772447, 18.42518152272070608 ) ) ;
#15109=CARTESIAN_POINT ( 'NONE',  ( -17.83459896181207682, -17.64923967996745446, 20.94377226548377990 ) ) ;
#15122=CARTESIAN_POINT ( 'NONE',  ( -5.055868909835983693, -26.71495157282352650, 12.14047268033097460 ) ) ;
#15125=CARTESIAN_POINT ( 'NONE',  ( -26.52907865026647016, -8.732139513722060542, 20.82122704794093693 ) ) ;
#15153=CARTESIAN_POINT ( 'NONE',  ( 20.08365402398579391, -19.49265790308171731, 20.69868183039781684 ) ) ;
#15183=CARTESIAN_POINT ( 'NONE',  ( 39.05366788551321378, -6.582903510435600403, 11.00000000000000000 ) ) ;
#15184=CARTESIAN_POINT ( 'NONE',  ( -29.43343111547412150, -25.34807889869424358, 14.53008259254020551 ) ) ;
#15196=CARTESIAN_POINT ( 'NONE',  ( -18.63686013482982773, 22.43247111565169405, 12.14047268035308136 ) ) ;
#15211=B_SPLINE_CURVE_WITH_KNOTS ( 'NONE', 3,
 ( #11863, #24253, #36257, #18168, #33809, #5957, #18361, #27692, #23655, #17575 ),
 .UNSPECIFIED., .F., .F.,
 ( 4, 2, 2, 2, 4 ),
 ( 0.7014259083631586567, 0.7760694312723689370, 0.8507129541815793283, 0.9253564770907896087, 1.000000000000000000 ),
 .UNSPECIFIED. ) ;
#15253=CARTESIAN_POINT ( 'NONE',  ( -12.30427675147431010, 35.50736440028104823, 12.73282698324895534 ) ) ;
#15255=CARTESIAN_POINT ( 'NONE',  ( 17.21213525677581657, -20.06193531423786780, 20.50957957746029336 ) ) ;
#15257=CARTESIAN_POINT ( 'NONE',  ( -5.506351411279842623, 29.74560631396580490, 20.50957957746029336 ) ) ;
#15261=CARTESIAN_POINT ( 'NONE',  ( -11.11100267139600639, 25.58833710557283680, 19.66345542862528717 ) ) ;
#15277=CARTESIAN_POINT ( 'NONE',  ( -27.60461630348678241, -20.46464247653241841, 19.27171037444157164 ) ) ;
#15288=CARTESIAN_POINT ( 'NONE',  ( 35.27625572565175815, 1.213838575767484107, 23.00000000000469669 ) ) ;
#15291=CARTESIAN_POINT ( 'NONE',  ( 18.23649648353767461, -16.09146789626181118, 20.99999999999999645 ) ) ;
#15295=EDGE_CURVE ( 'NONE', #28327, #8296, #22364, .T. ) ;
#15299=CARTESIAN_POINT ( 'NONE',  ( 33.56035593554180707, -14.08372035823031077, 17.92354375535250810 ) ) ;
#15304=CARTESIAN_POINT ( 'NONE',  ( 75.15099915297797395, 43.38844959084117647, 23.00000000000000000 ) ) ;
#15310=CARTESIAN_POINT ( 'NONE',  ( 28.63966609528962337, 4.835996017632539612, 12.73282698324585560 ) ) ;
#15321=CARTESIAN_POINT ( 'NONE',  ( -27.68412949013605839, -10.20944236610018940, 20.69868183039781329 ) ) ;
#15331=CARTESIAN_POINT ( 'NONE',  ( -30.33933116650765527, 6.243556997736136260, 10.99999999999999822 ) ) ;
#15349=CARTESIAN_POINT ( 'NONE',  ( 26.24102572422061996, -17.42682220599409604, 20.50957957746051719 ) ) ;
#15354=ORIENTED_EDGE ( 'NONE', *, *, #12997, .T. ) ;
#15358=CARTESIAN_POINT ( 'NONE',  ( -23.05386822411323422, -7.747535282638357224, 23.00000000000000000 ) ) ;
#15384=CARTESIAN_POINT ( 'NONE',  ( -32.21892379115398342, -22.89377427927484021, 14.53008259254002610 ) ) ;
#15395=CARTESIAN_POINT ( 'NONE',  ( -18.17912400190525801, 22.26280294339773036, 13.92931973829419690 ) ) ;
#15408=CARTESIAN_POINT ( 'NONE',  ( -19.48557158514998022, -11.24999999999982414, 23.00000000000000000 ) ) ;
#15422=CARTESIAN_POINT ( 'NONE',  ( -2.594149110900646260, 26.80855565015090747, 23.00000000000000000 ) ) ;
#15451=CARTESIAN_POINT ( 'NONE',  ( -16.50691157469147896, 29.07214648649221900, 13.32518128616527164 ) ) ;
#15454=CARTESIAN_POINT ( 'NONE',  ( -12.01634099001141287, -16.14815750352196844, 20.94377226548377990 ) ) ;
#15456=CARTESIAN_POINT ( 'NONE',  ( 10.77668768651791886, 26.79111211459907338, 19.66345542862663720 ) ) ;
#15476=CARTESIAN_POINT ( 'NONE',  ( -34.14640338304366196, -7.754617911608441716, 17.42190598798312706 ) ) ;
#15492=CARTESIAN_POINT ( 'NONE',  ( 39.05366788733157080, -6.582903524762554248, 11.00000000000000000 ) ) ;
#15503=CARTESIAN_POINT ( 'NONE',  ( 30.32526513703937709, -2.692717509694302791, 18.42518152272298693 ) ) ;
#15517=FACE_OUTER_BOUND ( 'NONE', #22777, .T. ) ;
#15527=CARTESIAN_POINT ( 'NONE',  ( -22.68370119258293016, -18.87043823706580525, 20.69868183039781329 ) ) ;
#15551=CARTESIAN_POINT ( 'NONE',  ( 28.60147806546228821, -12.08038679647185454, 20.50957957746028626 ) ) ;
#15559=CARTESIAN_POINT ( 'NONE',  ( -30.33922525723529873, 6.243664897713534501, 23.00000000001065814 ) ) ;
#15579=B_SPLINE_CURVE_WITH_KNOTS ( 'NONE', 3,
 ( #22750, #29660, #35763, #29057, #20124, #29456 ),
 .UNSPECIFIED., .F., .F.,
 ( 4, 2, 4 ),
 ( 0.000000000000000000, 0.5000000000000000000, 1.000000000000000000 ),
 .UNSPECIFIED. ) ;
#15582=CARTESIAN_POINT ( 'NONE',  ( -33.75875814100324845, 2.759858869446484064, 11.00000000000000000 ) ) ;
#15584=CARTESIAN_POINT ( 'NONE',  ( -17.04089262280391281, -28.02826808823053284, 15.13084544680188870 ) ) ;
#15594=CARTESIAN_POINT ( 'NONE',  ( -19.49168883800204455, 11.25353179757921751, 18.42518152272108978 ) ) ;
#15608=CARTESIAN_POINT ( 'NONE',  ( -19.48557158514998022, -11.24999999999982414, 3.000000000000000000 ) ) ;
#15609=FACE_OUTER_BOUND ( 'NONE', #24468, .T. ) ;
#15616=( BOUNDED_SURFACE ( )  B_SPLINE_SURFACE ( 2, 3, ( 
 ( #9068, #37292, #3170, #28144, #9467, #321 ),
 ( #120, #15559, #24699, #27946, #18022, #37096 ),
 ( #15358, #39934, #37495, #12311, #27750, #24900 ) ),
 .UNSPECIFIED., .F., .F., .F. ) 
 B_SPLINE_SURFACE_WITH_KNOTS ( ( 3, 3 ),
 ( 4, 2, 4 ),
 ( 0.000000000000000000, 1.000000000000000000 ),
 ( 5.507097317918141499, 5.759586531581287971, 6.012075745244433556 ),
 .UNSPECIFIED. ) 
 GEOMETRIC_REPRESENTATION_ITEM ( )  RATIONAL_B_SPLINE_SURFACE ( (
 ( 1.000000000000000000, 1.000000000000000000, 1.000000000000000000, 1.000000000000000000, 1.000000000000000000, 1.000000000000000000),
 ( 0.7071067811865474617, 0.7071067811865474617, 0.7071067811865474617, 0.7071067811865474617, 0.7071067811865474617, 0.7071067811865474617),
 ( 1.000000000000000000, 1.000000000000000000, 1.000000000000000000, 1.000000000000000000, 1.000000000000000000, 1.000000000000000000) ) ) 
 REPRESENTATION_ITEM ( '' )  SURFACE ( )  );
#15622=CARTESIAN_POINT ( 'NONE',  ( 18.68934290552659760, 29.94321432092586122, 23.00000000000375522 ) ) ;
#15653=CARTESIAN_POINT ( 'NONE',  ( 16.63496159151925369, 29.12310921430783850, 12.73282698324831941 ) ) ;
#15654=B_SPLINE_CURVE_WITH_KNOTS ( 'NONE', 3,
 ( #16822, #1375, #23710, #21262, #38951, #17832, #27355, #36310, #11722, #27160, #2582, #39742, #33473, #33670, #14369, #30210, #23508, #26959 ),
 .UNSPECIFIED., .F., .F.,
 ( 4, 2, 2, 2, 2, 2, 2, 2, 4 ),
 ( 0.000000000000000000, 0.1249999999999999722, 0.2499999999999999445, 0.3749999999999998890, 0.4999999999999998890, 0.6249999999999998890, 0.7499999999999997780, 0.8749999999999997780, 1.000000000000000000 ),
 .UNSPECIFIED. ) ;
#15658=CARTESIAN_POINT ( 'NONE',  ( -9.267781094590318958, 26.19038745656696676, 20.25080042701543448 ) ) ;
#15673=CARTESIAN_POINT ( 'NONE',  ( -18.97483082528767540, -25.68201547601522350, 17.92354375535288824 ) ) ;
#15695=CARTESIAN_POINT ( 'NONE',  ( 33.85500357264645999, -15.79720895788926427, 17.42190598798393353 ) ) ;
#15708=CARTESIAN_POINT ( 'NONE',  ( 32.28722999652337933, 1.315479119629257010, 12.14047268033097460 ) ) ;
#15718=CARTESIAN_POINT ( 'NONE',  ( -25.98021325959596695, -4.875178728620359614, 20.50957957746029336 ) ) ;
#15745=CARTESIAN_POINT ( 'NONE',  ( 27.36681752352244956, -15.80023946406895341, 20.50957957746029336 ) ) ;
#15780=CARTESIAN_POINT ( 'NONE',  ( -22.69494504450977956, -28.86495990325026284, 12.73282698324813644 ) ) ;
#15790=CARTESIAN_POINT ( 'NONE',  ( -25.97912795568404576, 2.630260520731678930, 17.92354375535789046 ) ) ;
#15798=CARTESIAN_POINT ( 'NONE',  ( 36.76835206499524844, -7.129807841006594593, 13.32518128616614739 ) ) ;
#15821=CARTESIAN_POINT ( 'NONE',  ( -2.166144593658632989, 42.50000000000004974, 22.99999999999999289 ) ) ;
#15851=ORIENTED_EDGE ( 'NONE', *, *, #3553, .F. ) ;
#15855=CARTESIAN_POINT ( 'NONE',  ( 9.166052203147213362, 37.72018303276097129, 13.32518128616612962 ) ) ;
#15857=DIRECTION ( 'NONE',  ( -0.000000000000000000, -0.000000000000000000, -1.000000000000000000 ) ) ;
#15858=CARTESIAN_POINT ( 'NONE',  ( 10.78342637327578046, 29.81468131102270291, 18.87996532025786323 ) ) ;
#15877=CARTESIAN_POINT ( 'NONE',  ( -32.26343921792069835, -3.257266818579767964, 17.42190598798350365 ) ) ;
#15900=CARTESIAN_POINT ( 'NONE',  ( 25.49851591039082876, -25.57752154475394946, 16.87380292611441845 ) ) ;
#15906=CARTESIAN_POINT ( 'NONE',  ( 0.5415361484146276050, 27.50000000000005684, 20.99999999999998934 ) ) ;
#15921=CARTESIAN_POINT ( 'NONE',  ( -28.61121519738577135, -15.27903652329813333, 20.25080042701592120 ) ) ;
#15950=CARTESIAN_POINT ( 'NONE',  ( 29.20803623499950419, -13.20745421916094209, 20.25080042701566541 ) ) ;
#15956=B_SPLINE_CURVE_WITH_KNOTS ( 'NONE', 3,
 ( #26651, #23610, #17527, #7197, #26853, #9372, #15261, #14865, #33368, #21748, #33767, #3068, #12012, #24004, #27649, #27253, #12410, #8972 ),
 .UNSPECIFIED., .F., .F.,
 ( 4, 2, 2, 2, 2, 2, 2, 2, 4 ),
 ( 0.000000000000000000, 0.1250000000000000833, 0.2500000000000001665, 0.3750000000000002220, 0.5000000000000003331, 0.6250000000000004441, 0.7500000000000002220, 0.8750000000000001110, 1.000000000000000000 ),
 .UNSPECIFIED. ) ;
#15980=ORIENTED_EDGE ( 'NONE', *, *, #31958, .F. ) ;
#15983=CARTESIAN_POINT ( 'NONE',  ( -26.32119069355245955, -27.53777429989661485, 13.32518128616608877 ) ) ;
#15992=CARTESIAN_POINT ( 'NONE',  ( -10.74031445979289856, 33.85370084240260269, 16.87380292611523913 ) ) ;
#15995=CARTESIAN_POINT ( 'NONE',  ( -24.95394407863866704, 1.780357051476928243, 18.87996532026248175 ) ) ;
#16001=CARTESIAN_POINT ( 'NONE',  ( 22.67022523934590694, -28.72937257582105275, 13.32518128616577080 ) ) ;
#16013=DIRECTION ( 'NONE',  ( 1.000000000000000000, 0.000000000000000000, 0.000000000000000000 ) ) ;
#16049=CARTESIAN_POINT ( 'NONE',  ( -16.76301160834940873, 29.17407194211730825, 12.14047268033010596 ) ) ;
#16053=CARTESIAN_POINT ( 'NONE',  ( 8.489237591500947033, 31.47375793094898810, 19.27171037444156099 ) ) ;
#16072=CARTESIAN_POINT ( 'NONE',  ( -33.53288488731320882, -7.900844017968387867, 17.92354375535173361 ) ) ;
#16098=CARTESIAN_POINT ( 'NONE',  ( 23.74914942275265162, -8.582573258223918700, 21.00000000000001776 ) ) ;
#16099=CARTESIAN_POINT ( 'NONE',  ( 18.93294331123277985, -26.86907422048189176, 16.87380292611448951 ) ) ;
#16105=CARTESIAN_POINT ( 'NONE',  ( 4.791301586986472572, 25.75006569903030851, 21.00000000000000355 ) ) ;
#16111=CARTESIAN_POINT ( 'NONE',  ( 25.71480618106366478, 9.014447550976075973, 11.00000000000101963 ) ) ;
#16121=CARTESIAN_POINT ( 'NONE',  ( -21.12676971146075289, -20.25531951604057568, 20.50957957746008375 ) ) ;
#16140=CARTESIAN_POINT ( 'NONE',  ( 19.26948696230199687, 27.85601271560034675, 3.000000000000000000 ) ) ;
#16148=CARTESIAN_POINT ( 'NONE',  ( 27.14644468510662279, -3.730463242941908231, 19.99202127657103389 ) ) ;
#16166=SURFACE_STYLE_USAGE ( .BOTH. , #37107 ) ;
#16171=ORIENTED_EDGE ( 'NONE', *, *, #10366, .F. ) ;
#16174=CARTESIAN_POINT ( 'NONE',  ( 37.09709568333406082, -7.051483854461560341, 11.00000000000008527 ) ) ;
#16185=CARTESIAN_POINT ( 'NONE',  ( -35.73872160561192146, -18.42674013420461776, 13.32518128616620423 ) ) ;
#16192=CARTESIAN_POINT ( 'NONE',  ( 1.681518492368163198, 38.03812643383474779, 16.87380292611441845 ) ) ;
#16195=CARTESIAN_POINT ( 'NONE',  ( -16.15127118876187140, 15.63943246416160981, 18.87996532025774599 ) ) ;
#16198=CARTESIAN_POINT ( 'NONE',  ( 24.27939416804019856, -12.77206359138141067, 22.99999999999999645 ) ) ;
#16201=CARTESIAN_POINT ( 'NONE',  ( 36.34526107768950709, -5.221918994412432014, 12.73282698324840467 ) ) ;
#16225=CARTESIAN_POINT ( 'NONE',  ( -8.437494165184659778, 40.76200631401351160, 23.00000000000000000 ) ) ;
#16237=DIRECTION ( 'NONE',  ( 1.000000000000000000, 0.000000000000000000, 0.000000000000000000 ) ) ;
#16240=VERTEX_POINT ( 'NONE', #11444 ) ;
#16255=CARTESIAN_POINT ( 'NONE',  ( -14.89626057892329847, 32.60452476689614087, 11.00000000000000000 ) ) ;
#16259=CARTESIAN_POINT ( 'NONE',  ( 12.55429062395116446, 25.98950339719798563, 18.87996532025784546 ) ) ;
#16263=CARTESIAN_POINT ( 'NONE',  ( -1.829593030691901284E-15, 22.50000000000001066, 3.000000000000000000 ) ) ;
#16274=CIRCLE ( 'NONE', #12388, 20.00000000000003908 ) ;
#16275=CARTESIAN_POINT ( 'NONE',  ( -25.86085639997994434, -26.44089909996126408, 15.72805884748940031 ) ) ;
#16283=CARTESIAN_POINT ( 'NONE',  ( -5.050662510305666153, -26.77689918168226058, 11.00000000000000178 ) ) ;
#16297=CARTESIAN_POINT ( 'NONE',  ( 34.38615473478414231, -15.96524117249927954, 16.87380292611441490 ) ) ;
#16299=CARTESIAN_POINT ( 'NONE',  ( 11.38745366800453063, 34.53793118711288201, 15.72805884748937011 ) ) ;
#16300=CARTESIAN_POINT ( 'NONE',  ( -19.26948696230207858, 27.85601271560029701, 23.00000000000000000 ) ) ;
#16302=CARTESIAN_POINT ( 'NONE',  ( -4.568463557893644555, 27.32878864566640686, 20.94377226548398241 ) ) ;
#16309=EDGE_CURVE ( 'NONE', #14259, #8510, #1624, .T. ) ;
#16311=CARTESIAN_POINT ( 'NONE',  ( 30.17922767059877032, -0.7536324250949818504, 17.42190598798392998 ) ) ;
#16319=CARTESIAN_POINT ( 'NONE',  ( -23.00727501322622714, -19.64144336131490221, 20.50957957746029336 ) ) ;
#16346=CARTESIAN_POINT ( 'NONE',  ( 23.94831201522132602, -21.88372720616970923, 19.66345542862529783 ) ) ;
#16376=ORIENTED_EDGE ( 'NONE', *, *, #37498, .T. ) ;
#16382=CARTESIAN_POINT ( 'NONE',  ( -16.95459465864602677, -28.62006465032632363, 13.92931973827769987 ) ) ;
#16390=CARTESIAN_POINT ( 'NONE',  ( -13.82587227205766389, 37.11292025503280456, 11.00000000000000000 ) ) ;
#16391=CARTESIAN_POINT ( 'NONE',  ( -1.681518492368433426, 38.03812643383474779, 16.87380292611441135 ) ) ;
#16394=CARTESIAN_POINT ( 'NONE',  ( -13.31403195207871981, 20.45929608442119729, 19.27171037444204060 ) ) ;
#16399=CARTESIAN_POINT ( 'NONE',  ( 31.34430980808824430, -24.70897660846287636, 12.14047268033096927 ) ) ;
#16435=DIRECTION ( 'NONE',  ( 1.000000000000000000, -1.734723475976805319E-15, 0.000000000000000000 ) ) ;
#16442=EDGE_CURVE ( 'NONE', #29890, #39914, #33562, .T. ) ;
#16444=CARTESIAN_POINT ( 'NONE',  ( -23.61737546510164165, -7.194424252576709478, 20.99999999999999645 ) ) ;
#16455=CARTESIAN_POINT ( 'NONE',  ( -12.39897218486444963, 35.60749793648266603, 12.14047268033129257 ) ) ;
#16458=CARTESIAN_POINT ( 'NONE',  ( 3.681484855442201720, 33.42880943655697479, 19.66345542862528717 ) ) ;
#16479=CARTESIAN_POINT ( 'NONE',  ( -30.90861030616400029, -0.03770625498372660866, 16.30093088680191116 ) ) ;
#16504=CARTESIAN_POINT ( 'NONE',  ( 24.21699896819641040, -27.13078975446658703, 15.72805884748975558 ) ) ;
#16506=CARTESIAN_POINT ( 'NONE',  ( 13.63376536442992837, 31.74814110635675846, 15.72805884748940031 ) ) ;
#16508=CARTESIAN_POINT ( 'NONE',  ( -6.175735745372779917, 24.95935742585754014, 20.94377226548369109 ) ) ;
#16517=CARTESIAN_POINT ( 'NONE',  ( 26.89145897429045107, 3.386615419904837498, 16.87380292612509436 ) ) ;
#16525=CARTESIAN_POINT ( 'NONE',  ( -30.09689698601766850, -15.93509466225727422, 19.66345542862561757 ) ) ;
#16546=B_SPLINE_CURVE_WITH_KNOTS ( 'NONE', 3,
 ( #38999, #33119, #11969, #24360, #36757, #21317, #33723, #11172, #23564, #35959, #5469, #20522, #32916, #2430, #5075, #39392, #17684, #29853 ),
 .UNSPECIFIED., .F., .F.,
 ( 4, 2, 2, 2, 2, 2, 2, 2, 4 ),
 ( 0.000000000000000000, 0.1250000000000000000, 0.2500000000000000000, 0.3750000000000000000, 0.5000000000000000000, 0.6250000000000000000, 0.7500000000000000000, 0.8750000000000000000, 1.000000000000000000 ),
 .UNSPECIFIED. ) ;
#16551=CARTESIAN_POINT ( 'NONE',  ( 20.20329687195648560, -21.14155277498772278, 20.25080042701565830 ) ) ;
#16576=CARTESIAN_POINT ( 'NONE',  ( -25.03753813966994102, -13.00734255224434577, 20.99999999999999645 ) ) ;
#16588=CARTESIAN_POINT ( 'NONE',  ( -34.90171719354061253, -20.15051581687081139, 12.73282698324853079 ) ) ;
#16597=CARTESIAN_POINT ( 'NONE',  ( 7.775297188276389271, 35.41132985342715500, 17.42190598798394063 ) ) ;
#16603=CARTESIAN_POINT ( 'NONE',  ( 23.54493052986456547, -14.21898406159490413, 20.99999999999999645 ) ) ;
#16606=CARTESIAN_POINT ( 'NONE',  ( 34.66557409316544636, -1.755032161644171085, 12.73282698324864803 ) ) ;
#16630=CARTESIAN_POINT ( 'NONE',  ( 2.166144593658585471, 42.50000000000004974, 11.00000000000000000 ) ) ;
#16652=CARTESIAN_POINT ( 'NONE',  ( -30.17922767059062394, -0.7536324250866187624, 17.42190598798393708 ) ) ;
#16659=CARTESIAN_POINT ( 'NONE',  ( 1.947644445291113025, 40.50000000000006395, 11.00000000000000178 ) ) ;
#16662=CARTESIAN_POINT ( 'NONE',  ( 9.543723562658483317, 28.97375833662212941, 19.66345542862530138 ) ) ;
#16667=CARTESIAN_POINT ( 'NONE',  ( 17.34253826607184479, 27.32041144404033162, 23.00000000000000000 ) ) ;
#16679=CARTESIAN_POINT ( 'NONE',  ( -2.109373541296176935, 27.06550157850341876, 20.99999999999999289 ) ) ;
#16683=CARTESIAN_POINT ( 'NONE',  ( -32.86149060640480712, -21.03113892363543869, 15.72805884748907879 ) ) ;
#16706=CARTESIAN_POINT ( 'NONE',  ( 24.08250333996883441, -26.67951267124112746, 16.30093088680228774 ) ) ;
#16708=CARTESIAN_POINT ( 'NONE',  ( 1.782755275185735400, 38.97445513318768207, 15.72805884748939853 ) ) ;
#16710=CARTESIAN_POINT ( 'NONE',  ( -16.60464863831923310, -22.41657912772977213, 19.66345542862528717 ) ) ;
#16712=CARTESIAN_POINT ( 'NONE',  ( 4.439345875601470759, 26.26892473594527289, 21.00000000000000355 ) ) ;
#16719=CARTESIAN_POINT ( 'NONE',  ( 29.73172958077877581, -1.192874570370699328, 17.92354375535250810 ) ) ;
#16721=EDGE_CURVE ( 'NONE', #39914, #28188, #8259, .T. ) ;
#16730=CARTESIAN_POINT ( 'NONE',  ( -21.56514238326832000, -22.66165022683772889, 19.66345542862498519 ) ) ;
#16752=CARTESIAN_POINT ( 'NONE',  ( -18.76090689389218014, -16.22676322417297001, 23.00000000000000000 ) ) ;
#16757=CARTESIAN_POINT ( 'NONE',  ( 18.04765032505117972, -21.12132759291071693, 20.25080042701545580 ) ) ;
#16786=ORIENTED_EDGE ( 'NONE', *, *, #3444, .F. ) ;
#16790=CARTESIAN_POINT ( 'NONE',  ( -18.84783625459284906, -29.28148485008969715, 12.14047268033134763 ) ) ;
#16801=CARTESIAN_POINT ( 'NONE',  ( 14.97058623676931077, 26.66112013780997003, 16.87380292611441135 ) ) ;
#16805=CARTESIAN_POINT ( 'NONE',  ( -14.06669941890059761, 14.65883224165446208, 19.99202127657103389 ) ) ;
#16811=CARTESIAN_POINT ( 'NONE',  ( 36.93643098903794453, -14.76343610888346092, 12.73282698324853257 ) ) ;
#16822=CARTESIAN_POINT ( 'NONE',  ( 17.34253826607184479, 27.32041144404033162, 11.00000000000000000 ) ) ;
#16845=CARTESIAN_POINT ( 'NONE',  ( -20.38753357181593628, -16.19769905861789994, 21.00000000000001421 ) ) ;
#16865=CARTESIAN_POINT ( 'NONE',  ( 3.900486991066165476, 40.17991855518013011, 11.55979286843954412 ) ) ;
#16869=CARTESIAN_POINT ( 'NONE',  ( -7.884092257453602315, 32.87438847863548119, 18.87996532025784546 ) ) ;
#16884=CARTESIAN_POINT ( 'NONE',  ( 18.23649648353767461, -16.09146789626181118, 20.99999999999999645 ) ) ;
#16889=CARTESIAN_POINT ( 'NONE',  ( -31.71434132860544963, -22.43226626709165572, 15.72805884748934524 ) ) ;
#16911=CARTESIAN_POINT ( 'NONE',  ( 29.03912765165501142, -24.78940378269167866, 15.72805884748905747 ) ) ;
#16913=CARTESIAN_POINT ( 'NONE',  ( 9.968062119477529848, 35.61660815598495589, 15.72805884748939498 ) ) ;
#16915=CARTESIAN_POINT ( 'NONE',  ( 11.32166530370859547, -20.22988973179433003, 19.99202127657019901 ) ) ;
#16917=CARTESIAN_POINT ( 'NONE',  ( -5.000428297553742851, 29.07988060316462864, 20.69868183039781329 ) ) ;
#16922=CARTESIAN_POINT ( 'NONE',  ( 27.61482536617424444, 3.986323854220331420, 15.72805884749758931 ) ) ;
#16932=CARTESIAN_POINT ( 'NONE',  ( -28.78203904708374949, -16.61731799165967871, 19.99202127657103034 ) ) ;
#16952=CARTESIAN_POINT ( 'NONE',  ( -39.59914439355408433, -10.88071517532302757, 23.00000000000187583 ) ) ;
#16958=CARTESIAN_POINT ( 'NONE',  ( 25.82842257350687021, -22.71926374633472534, 18.87996532025747953 ) ) ;
#16982=CARTESIAN_POINT ( 'NONE',  ( -24.28032989564857047, -12.76774640304084052, 20.99999999999999645 ) ) ;
#16993=CARTESIAN_POINT ( 'NONE',  ( -32.84658669524019103, -23.46788009898594041, 11.55979286843917819 ) ) ;
#17006=CARTESIAN_POINT ( 'NONE',  ( -10.34254640628522992, 25.37474234118948502, 19.99202127657103389 ) ) ;
#17008=FACE_OUTER_BOUND ( 'NONE', #1722, .T. ) ;
#17010=B_SPLINE_CURVE_WITH_KNOTS ( 'NONE', 3,
 ( #37333, #21491, #18453, #18652, #3008, #30843, #40175, #37135, #3602, #19437, #16198, #22280, #28582, #12941, #37535, #10501, #25135, #756 ),
 .UNSPECIFIED., .F., .F.,
 ( 4, 2, 2, 2, 2, 2, 2, 2, 4 ),
 ( 0.000000000000000000, 0.1249999999999998335, 0.2499999999999996669, 0.3749999999999995004, 0.4999999999999993339, 0.6249999999999994449, 0.7499999999999996669, 0.8749999999999997780, 1.000000000000000000 ),
 .UNSPECIFIED. ) ;
#17013=CARTESIAN_POINT ( 'NONE',  ( 37.03648387062805369, -7.065924075331559528, 12.14047268033105098 ) ) ;
#17014=VERTEX_POINT ( 'NONE', #9499 ) ;
#17068=CARTESIAN_POINT ( 'NONE',  ( 13.41665185498674973, 27.84207739518157609, 17.92354375535403577 ) ) ;
#17090=CARTESIAN_POINT ( 'NONE',  ( -18.93291711864322480, -26.86907612099998133, 16.87380292611481991 ) ) ;
#17111=ORIENTED_EDGE ( 'NONE', *, *, #35746, .T. ) ;
#17114=EDGE_CURVE ( 'NONE', #23396, #24869, #11594, .T. ) ;
#17115=CARTESIAN_POINT ( 'NONE',  ( 32.21892379115691796, -22.89377427927269792, 14.53008259254040269 ) ) ;
#17117=STYLED_ITEM ( 'NONE', ( #11966 ), #19702 ) ;
#17118=CARTESIAN_POINT ( 'NONE',  ( -5.109761443619218468, 37.66877327392096220, 16.30093088680190760 ) ) ;
#17119=CARTESIAN_POINT ( 'NONE',  ( 11.06125417662034316, -21.75993793940401133, 19.27171037444025359 ) ) ;
#17121=CARTESIAN_POINT ( 'NONE',  ( 5.712781365378005738, 28.53852268908861589, 20.69868183039781329 ) ) ;
#17127=EDGE_CURVE ( 'NONE', #6337, #28188, #25922, .T. ) ;
#17131=CARTESIAN_POINT ( 'NONE',  ( 20.03472765055001759, 11.56705540218561268, 17.92354375535250810 ) ) ;
#17140=CARTESIAN_POINT ( 'NONE',  ( -19.10349291421378837, -22.04058051679151831, 19.99202127657131101 ) ) ;
#17155=CARTESIAN_POINT ( 'NONE',  ( 39.51968005975199105, -13.07391886567316774, 22.99999999999999645 ) ) ;
#17161=CARTESIAN_POINT ( 'NONE',  ( -23.05386822411328041, -7.747535282638268406, 23.00000000000000000 ) ) ;
#17166=CARTESIAN_POINT ( 'NONE',  ( 29.15792305772562898, -20.09428552990231509, 18.87996532025821494 ) ) ;
#17189=CARTESIAN_POINT ( 'NONE',  ( -25.22909892406959997, -10.52103384677036502, 20.99999999999999645 ) ) ;
#17199=CARTESIAN_POINT ( 'NONE',  ( -36.53368004180960327, -5.154483866377498558, 11.00000000000028955 ) ) ;
#17205=CARTESIAN_POINT ( 'NONE',  ( -18.68939205906154655, 29.94303747981212993, 11.00000000000000178 ) ) ;
#17212=CARTESIAN_POINT ( 'NONE',  ( -16.18987435794524288, 9.347228318705029793, 20.25080042701566541 ) ) ;
#17213=CARTESIAN_POINT ( 'NONE',  ( 19.90456025098515624, -17.02442174103823191, 20.99999999999999645 ) ) ;
#17218=CARTESIAN_POINT ( 'NONE',  ( 28.24711154207343000, -27.09388640670305293, 11.00000000000010481 ) ) ;
#17265=VERTEX_POINT ( 'NONE', #22672 ) ;
#17269=CIRCLE ( 'NONE', #10116, 57.99999999999995026 ) ;
#17276=CARTESIAN_POINT ( 'NONE',  ( -10.52847790146128126, 31.43738312353774234, 18.42518152272106491 ) ) ;
#17279=SHAPE_REPRESENTATION_RELATIONSHIP ( 'NONE' , 'NONE' ,  #12760, #19702 ) ;
#17283=EDGE_CURVE ( 'NONE', #8510, #24176, #21304, .T. ) ;
#17286=ORIENTED_EDGE ( 'NONE', *, *, #2330, .F. ) ;
#17296=CARTESIAN_POINT ( 'NONE',  ( -33.65490896085638184, -21.61118400457242572, 13.92931973827790770 ) ) ;
#17317=CARTESIAN_POINT ( 'NONE',  ( 33.17211272335703143, -21.25822893968285854, 15.13084544680211430 ) ) ;
#17319=CARTESIAN_POINT ( 'NONE',  ( -14.97435799694009795, 30.45328679654753756, 15.13084544680204147 ) ) ;
#17320=CARTESIAN_POINT ( 'NONE',  ( 5.409649191045219574, -22.50706359516090060, 18.42518152272108978 ) ) ;
#17322=CARTESIAN_POINT ( 'NONE',  ( -2.374005179830599666, 29.54744178790028997, 20.82122704794079837 ) ) ;
#17332=CARTESIAN_POINT ( 'NONE',  ( 8.859192577249610068, 12.20922670554003631, 20.99999999999999645 ) ) ;
#17334=CARTESIAN_POINT ( 'NONE',  ( 9.340438144417392508, 38.00965938232019425, 11.00000000000005329 ) ) ;
#17342=CARTESIAN_POINT ( 'NONE',  ( -17.81343984362097643, -22.72844136247609015, 19.66345542862531559 ) ) ;
#17351=PLANE ( 'NONE',  #8207 ) ;
#17362=CARTESIAN_POINT ( 'NONE',  ( -31.08218589456736680, -27.68808744833886948, 11.00000000000000000 ) ) ;
#17370=CARTESIAN_POINT ( 'NONE',  ( 31.82690166321389924, -6.837813000313431644, 18.87996532025749374 ) ) ;
#17405=CARTESIAN_POINT ( 'NONE',  ( -24.65531199400788509, -28.60128534115780141, 10.99999999999993427 ) ) ;
#17418=CARTESIAN_POINT ( 'NONE',  ( -23.61737546510163810, -7.194424252576709478, 20.99999999999999645 ) ) ;
#17419=CARTESIAN_POINT ( 'NONE',  ( 24.96922983059882384, -9.289877593706156844, 20.99999999999995026 ) ) ;
#17426=ORIENTED_EDGE ( 'NONE', *, *, #6115, .F. ) ;
#17434=DIRECTION ( 'NONE',  ( -1.000000000000000000, 0.000000000000000000, 0.000000000000000000 ) ) ;
#17460=ORIENTED_EDGE ( 'NONE', *, *, #13359, .T. ) ;
#17466=ORIENTED_EDGE ( 'NONE', *, *, #31958, .T. ) ;
#17477=CARTESIAN_POINT ( 'NONE',  ( 18.69515074622676565, 22.45407711375075976, 10.99999999997785949 ) ) ;
#17496=CARTESIAN_POINT ( 'NONE',  ( -31.02271782694906932, -24.34398845624585306, 13.92931973827809067 ) ) ;
#17518=CARTESIAN_POINT ( 'NONE',  ( 35.97875289183331660, -7.317948980263661696, 15.13084544680216759 ) ) ;
#17520=CARTESIAN_POINT ( 'NONE',  ( -13.95035364761271346, 31.96289125330682168, 15.13084544680213561 ) ) ;
#17521=CARTESIAN_POINT ( 'NONE',  ( -5.356921161177144342, -23.13411080437162326, 17.92354375535250810 ) ) ;
#17523=CARTESIAN_POINT ( 'NONE',  ( -1.790359260782678597, 30.61752677313652882, 20.69868183039780973 ) ) ;
#17527=CARTESIAN_POINT ( 'NONE',  ( -6.367390439426523052, 24.26983560722021238, 20.94377226548377635 ) ) ;
#17532=CARTESIAN_POINT ( 'NONE',  ( 11.82346474098068789, 13.60361205941433660, 20.69868183039785947 ) ) ;
#17542=CARTESIAN_POINT ( 'NONE',  ( -31.47522604700202109, -16.54376571344602809, 18.87996532025822205 ) ) ;
#17567=CARTESIAN_POINT ( 'NONE',  ( 32.58967084635737166, -11.00843821516718180, 18.87996532025784191 ) ) ;
#17575=CARTESIAN_POINT ( 'NONE',  ( -32.33143948541797386, 1.358872982501903248, 11.00000000000000000 ) ) ;
#17592=CARTESIAN_POINT ( 'NONE',  ( 5.121747905603605489, -25.93120163663720845, 14.53008259254011136 ) ) ;
#17595=CARTESIAN_POINT ( 'NONE',  ( -23.31768133719846503, -16.68166585059926632, 20.94377226548377990 ) ) ;
#17604=CARTESIAN_POINT ( 'NONE',  ( -29.88800841291100596, -25.99212743942916148, 12.14047268033113269 ) ) ;
#17616=ORIENTED_EDGE ( 'NONE', *, *, #7856, .T. ) ;
#17623=CARTESIAN_POINT ( 'NONE',  ( 19.27923728834097616, -17.06979480964821860, 20.99999999999999645 ) ) ;
#17640=FACE_OUTER_BOUND ( 'NONE', #12473, .T. ) ;
#17653=CARTESIAN_POINT ( 'NONE',  ( 35.72300735678889794, -23.12593625888495552, 11.00000000000000178 ) ) ;
#17662=CIRCLE ( 'NONE', #35153, 19.99999999999993605 ) ;
#17681=( NAMED_UNIT ( * ) PLANE_ANGLE_UNIT ( ) SI_UNIT ( $, .RADIAN. ) );
#17684=CARTESIAN_POINT ( 'NONE',  ( -4.671003766000858981, 24.36559561389090689, 23.00000000000000000 ) ) ;
#17718=CARTESIAN_POINT ( 'NONE',  ( 32.86149060640417474, -21.03113892363574422, 15.72805884748937721 ) ) ;
#17720=CARTESIAN_POINT ( 'NONE',  ( -5.571153519069262039, 39.03845596069744062, 13.92931973827808534 ) ) ;
#17722=CARTESIAN_POINT ( 'NONE',  ( 11.87696897078051350, -16.96707895818725831, 20.82122704794063495 ) ) ;
#17724=CARTESIAN_POINT ( 'NONE',  ( 5.506351411278700425, 29.74560631396668597, 20.50957957746029692 ) ) ;
#17726=CARTESIAN_POINT ( 'NONE',  ( 32.33143948541787438, 1.358872982501792226, 23.00000000000000000 ) ) ;
#17734=CARTESIAN_POINT ( 'NONE',  ( 17.01074486384225892, 2.963432112715942868, 20.82122704794076995 ) ) ;
#17745=CARTESIAN_POINT ( 'NONE',  ( -33.29356883319611171, -10.99541271083418614, 18.42518152272184295 ) ) ;
#17765=CARTESIAN_POINT ( 'NONE',  ( -16.58691282011878698, -31.15705289669003264, 22.99999999999999289 ) ) ;
#17770=CIRCLE ( 'NONE', #24205, 18.00000000000003553 ) ;
#17771=CARTESIAN_POINT ( 'NONE',  ( 30.76885290917950044, -8.559665202947678964, 19.66345542862528006 ) ) ;
#17793=CARTESIAN_POINT ( 'NONE',  ( 15.37000524125214440, -27.20210912714641793, 15.72805884748939498 ) ) ;
#17797=CARTESIAN_POINT ( 'NONE',  ( -25.96434769773127726, -12.55439225991604779, 20.94377226548378346 ) ) ;
#17822=CARTESIAN_POINT ( 'NONE',  ( 24.18603102892799583, -14.68777056910919576, 20.99999999999999645 ) ) ;
#17825=CARTESIAN_POINT ( 'NONE',  ( 36.04785107591604287, -18.56329043283700031, 11.00000000000005862 ) ) ;
#17832=CARTESIAN_POINT ( 'NONE',  ( 16.24129362380266883, 27.01431713449538918, 15.13084544680213206 ) ) ;
#17837=CARTESIAN_POINT ( 'NONE',  ( 4.881458130668207218, -28.77689918168226413, 22.99999999999999645 ) ) ;
#17860=CARTESIAN_POINT ( 'NONE',  ( -32.09165771328039085, 1.123514972298483627, 13.32518128616608699 ) ) ;
#17914=CARTESIAN_POINT ( 'NONE',  ( 36.79828514077289725, -9.052677438810906807, 13.92931973827808534 ) ) ;
#17915=VERTEX_POINT ( 'NONE', #16140 ) ;
#17916=CARTESIAN_POINT ( 'NONE',  ( -11.85731412588568823, 35.03474529413922056, 14.53008259254079171 ) ) ;
#17918=CARTESIAN_POINT ( 'NONE',  ( 5.730292628140436939, -18.69445663741131014, 20.25080042701566541 ) ) ;
#17920=CARTESIAN_POINT ( 'NONE',  ( -4.183427099969815544, 31.55590659971976919, 20.25080042701566185 ) ) ;
#17930=CARTESIAN_POINT ( 'NONE',  ( 24.20198940123849951, -6.620595927253059898, 20.94377226548378346 ) ) ;
#17933=CARTESIAN_POINT ( 'NONE',  ( 17.34253826607184479, 27.32041144404033162, 11.00000000000000000 ) ) ;
#17940=CARTESIAN_POINT ( 'NONE',  ( -32.94564365859725541, -13.95995841273573390, 18.42518152272108622 ) ) ;
#17953=CARTESIAN_POINT ( 'NONE',  ( 14.48927117870122494, -30.61587158504688233, 11.00000000000000000 ) ) ;
#17962=CARTESIAN_POINT ( 'NONE',  ( 21.96131288150857586, -24.83662238097890906, 18.42518152272107912 ) ) ;
#17983=CARTESIAN_POINT ( 'NONE',  ( 4.261257190324624642E-14, -26.71495157282352650, 12.14047268033097460 ) ) ;
#17987=CARTESIAN_POINT ( 'NONE',  ( -25.20894334605400999, -14.55439022682983996, 20.94377226548377990 ) ) ;
#17998=CARTESIAN_POINT ( 'NONE',  ( -22.48079666807009147, 18.61591633964213344, 10.99999999999999645 ) ) ;
#18002=CARTESIAN_POINT ( 'NONE',  ( -21.91981567634955042, -15.65087685632102499, 20.99999999999999645 ) ) ;
#18013=CARTESIAN_POINT ( 'NONE',  ( 28.51362642450516915, -10.10416295265137165, 20.50957957746028981 ) ) ;
#18016=CARTESIAN_POINT ( 'NONE',  ( 34.10020663062365287, -21.93670956716284337, 10.99999999999993960 ) ) ;
#18022=CARTESIAN_POINT ( 'NONE',  ( -20.57678504286234755, 23.15270735508189759, 22.99999999999999645 ) ) ;
#18055=CARTESIAN_POINT ( 'NONE',  ( -25.66376117784755095, 8.978964872303784261, 12.14047268033272786 ) ) ;
#18057=DIRECTION ( 'NONE',  ( -0.000000000000000000, -0.000000000000000000, -1.000000000000000000 ) ) ;
#18105=CARTESIAN_POINT ( 'NONE',  ( -18.23649648353780961, -16.09146789626143814, 23.00000000000000000 ) ) ;
#18114=CARTESIAN_POINT ( 'NONE',  ( 20.77381726376787086, -29.00435581194094325, 12.73282698324852724 ) ) ;
#18117=CARTESIAN_POINT ( 'NONE',  ( -16.03057579645021491, 28.88256098452011145, 14.53008259253939194 ) ) ;
#18120=CARTESIAN_POINT ( 'NONE',  ( 1.161969254298447884, 33.23463598332013191, 19.99202127657103034 ) ) ;
#18129=CARTESIAN_POINT ( 'NONE',  ( 7.962467718759976165, 24.71319220552188156, 20.69868183039781329 ) ) ;
#18138=CARTESIAN_POINT ( 'NONE',  ( -26.60725962520553622, -21.34341596033566901, 19.27171037444156809 ) ) ;
#18152=CARTESIAN_POINT ( 'NONE',  ( 36.53988293556055567, -0.5802930328960469453, 23.00000000000094147 ) ) ;
#18162=CARTESIAN_POINT ( 'NONE',  ( 33.72852460920453410, -9.442290196614045783, 17.92354375535250810 ) ) ;
#18163=VERTEX_POINT ( 'NONE', #15291 ) ;
#18168=CARTESIAN_POINT ( 'NONE',  ( -36.92299321678470392, -6.638097534484090012, 10.99999999999989342 ) ) ;
#18179=CARTESIAN_POINT ( 'NONE',  ( 15.20016916874808288, -27.86040092368543242, 14.53008259254010959 ) ) ;
#18183=CARTESIAN_POINT ( 'NONE',  ( -26.76156665933352130, -9.514918190648881335, 20.82122704794052126 ) ) ;
#18210=CARTESIAN_POINT ( 'NONE',  ( 26.52908095339053673, -8.732144267389724490, 20.82122704794066692 ) ) ;
#18214=ORIENTED_EDGE ( 'NONE', *, *, #12997, .F. ) ;
#18232=CARTESIAN_POINT ( 'NONE',  ( -4.881458130820804264, -28.77689918168226058, 10.99999999999999645 ) ) ;
#18236=CARTESIAN_POINT ( 'NONE',  ( 31.24272016125543772, 0.2902395683448326102, 15.72805884748939498 ) ) ;
#18242=CARTESIAN_POINT ( 'NONE',  ( -33.41351084210700151, -21.43470647212746272, 14.53008259253988399 ) ) ;
#18253=CARTESIAN_POINT ( 'NONE',  ( -25.01795332078377143, 8.530037020297342565, 14.53008259254123757 ) ) ;
#18272=DIRECTION ( 'NONE',  ( -1.000000000000000000, 0.000000000000000000, 0.000000000000000000 ) ) ;
#18289=CARTESIAN_POINT ( 'NONE',  ( -39.35969763408572675, -8.663070498340031733, 11.00000000000000355 ) ) ;
#18297=VERTEX_POINT ( 'NONE', #21778 ) ;
#18308=CARTESIAN_POINT ( 'NONE',  ( 3.887054626305054938, 40.11907545043354872, 12.14047268033114690 ) ) ;
#18309=CARTESIAN_POINT ( 'NONE',  ( -5.661571401657330860, -19.51153516500234630, 19.99202127657103389 ) ) ;
#18312=CARTESIAN_POINT ( 'NONE',  ( 4.528037020496070930, 32.30201321073025156, 19.99202127657103389 ) ) ;
#18328=CARTESIAN_POINT ( 'NONE',  ( -31.84188463419280879, -5.263436490338604834, 18.42518152272108978 ) ) ;
#18343=CARTESIAN_POINT ( 'NONE',  ( 37.88915195766846722, -19.37406375362047228, 11.00000000000000000 ) ) ;
#18353=CARTESIAN_POINT ( 'NONE',  ( 24.79887074938343616, -23.91042127310592846, 18.42518152272109688 ) ) ;
#18361=CARTESIAN_POINT ( 'NONE',  ( -35.16163374036107570, -2.327860755070493060, 10.99999999999982414 ) ) ;
#18366=CARTESIAN_POINT ( 'NONE',  ( 23.13582672293635056, 13.35747578641157851, 12.14047268033097460 ) ) ;
#18378=CARTESIAN_POINT ( 'NONE',  ( -26.92296394334159260, -7.646625634049264875, 20.69868183039781329 ) ) ;
#18406=CARTESIAN_POINT ( 'NONE',  ( 23.00727501322602819, -19.64144336131528590, 20.50957957746028626 ) ) ;
#18423=CARTESIAN_POINT ( 'NONE',  ( -12.28720923544494248, -14.55658080566520418, 23.00000000000000000 ) ) ;
#18439=CARTESIAN_POINT ( 'NONE',  ( -36.66879582113860181, -12.81605961718980602, 14.53008259253997636 ) ) ;
#18450=CARTESIAN_POINT ( 'NONE',  ( -16.81416712651596868, 27.17354907308742185, 13.92931973827808712 ) ) ;
#18453=CARTESIAN_POINT ( 'NONE',  ( 19.30289106310104685, -16.27633469853321557, 23.00000000000000000 ) ) ;
#18462=CYLINDRICAL_SURFACE ( 'NONE', #12357, 17.99999999999992895 ) ;
#18478=CARTESIAN_POINT ( 'NONE',  ( -0.5415361484146629101, 27.50000000000004974, 23.00000000000000000 ) ) ;
#18502=DIRECTION ( 'NONE',  ( -0.000000000000000000, -0.000000000000000000, -1.000000000000000000 ) ) ;
#18507=CARTESIAN_POINT ( 'NONE',  ( 1.911335737650396993, 40.16401087634233846, 13.32518128616608877 ) ) ;
#18508=CARTESIAN_POINT ( 'NONE',  ( -6.143904198944369455, -13.77689918168226235, 20.99999999999999645 ) ) ;
#18509=CARTESIAN_POINT ( 'NONE',  ( -14.98890121934603314, -28.67928442654204346, 2.999999999999999112 ) ) ;
#18511=CARTESIAN_POINT ( 'NONE',  ( 9.267781094589551572, 26.19038745656764533, 20.25080042701674543 ) ) ;
#18529=CARTESIAN_POINT ( 'NONE',  ( -28.97703757779445866, -22.02226062111172311, 17.92354375535250810 ) ) ;
#18552=CARTESIAN_POINT ( 'NONE',  ( 26.47427689499786041, -23.88731992525525172, 17.92354375535211730 ) ) ;
#18567=CARTESIAN_POINT ( 'NONE',  ( 31.94006737154954934, 0.9747213384812106751, 13.92931973827808712 ) ) ;
#18576=CARTESIAN_POINT ( 'NONE',  ( -18.16616693041741470, -20.30807083247755784, 20.50957957746031823 ) ) ;
#18606=CARTESIAN_POINT ( 'NONE',  ( 28.63766977552451465, -11.08150102882311216, 20.50957957746029336 ) ) ;
#18614=AXIS2_PLACEMENT_3D ( 'NONE', #30395, #14948, #33651 ) ;
#18638=CARTESIAN_POINT ( 'NONE',  ( -36.20842572154693073, -9.127542156328868117, 15.13084544680213384 ) ) ;
#18649=CARTESIAN_POINT ( 'NONE',  ( -16.37862447372143038, 21.59537890665771798, 16.87380292611990384 ) ) ;
#18652=CARTESIAN_POINT ( 'NONE',  ( 20.39194369155392295, -16.19744444934939764, 22.99999999999999289 ) ) ;
#18661=CARTESIAN_POINT ( 'NONE',  ( 27.36225479881668576, 10.16098284218095493, 22.99999999999999645 ) ) ;
#18675=CARTESIAN_POINT ( 'NONE',  ( 4.441848239913452900, 24.85865334748800848, 23.00000000000000355 ) ) ;
#18706=CARTESIAN_POINT ( 'NONE',  ( 10.85362879025560545, 36.78189293023390150, 12.14047268033097637 ) ) ;
#18710=CARTESIAN_POINT ( 'NONE',  ( -6.290729337819993994, 29.14951258272757073, 20.50957957746074456 ) ) ;
#18728=CARTESIAN_POINT ( 'NONE',  ( -20.52459090776379114, -25.56956579041120747, 17.92354375535250810 ) ) ;
#18752=CARTESIAN_POINT ( 'NONE',  ( 27.81120771500035005, -23.04947625254933286, 17.92354375535213862 ) ) ;
#18764=CARTESIAN_POINT ( 'NONE',  ( 20.35904855840089311, 17.61891361913472309, 13.32518128616558784 ) ) ;
#18773=CARTESIAN_POINT ( 'NONE',  ( -24.76266088601904514, -18.72941319223700773, 20.50957957746028981 ) ) ;
#18802=CARTESIAN_POINT ( 'NONE',  ( 25.50184330511968156, -18.07811769911567978, 20.50957957746029336 ) ) ;
#18807=CARTESIAN_POINT ( 'NONE',  ( -9.742785792574970571, -49.01344959084108410, 20.99999999999999645 ) ) ;
#18835=CARTESIAN_POINT ( 'NONE',  ( -20.76390118686629549, -28.86769433464280610, 13.32518128616608877 ) ) ;
#18841=CARTESIAN_POINT ( 'NONE',  ( -12.25578195141909177, -14.54847271968242595, 23.00000000000000000 ) ) ;
#18845=CARTESIAN_POINT ( 'NONE',  ( -19.72827082055129111, 4.852702923346353892, 19.99202127657103389 ) ) ;
#18851=CARTESIAN_POINT ( 'NONE',  ( 31.94006737154590070, 0.9747213384848182338, 13.92931973827809067 ) ) ;
#18856=CARTESIAN_POINT ( 'NONE',  ( 20.57678504272533004, 23.15270735503113286, 11.00000000000000000 ) ) ;
#18892=CARTESIAN_POINT ( 'NONE',  ( 75.15099915297797395, 43.38844959084117647, 3.000000000000000000 ) ) ;
#18893=FACE_OUTER_BOUND ( 'NONE', #4739, .T. ) ;
#18897=ORIENTED_EDGE ( 'NONE', *, *, #36804, .T. ) ;
#18900=CARTESIAN_POINT ( 'NONE',  ( 5.682704777076756031, 39.36960561607962461, 12.73282698324853257 ) ) ;
#18904=CARTESIAN_POINT ( 'NONE',  ( -11.11100267139600639, 25.58833710557283325, 19.66345542862528362 ) ) ;
#18923=CARTESIAN_POINT ( 'NONE',  ( -34.20210851612425529, -5.988401547694746974, 16.87380292611485899 ) ) ;
#18946=CARTESIAN_POINT ( 'NONE',  ( 31.75251099004278288, -1.565804367081077064, 16.87380292611637245 ) ) ;
#18964=CARTESIAN_POINT ( 'NONE',  ( 19.26948696230199687, 27.85601271560034675, 23.00000000000000000 ) ) ;
#18969=CARTESIAN_POINT ( 'NONE',  ( -29.32420241873618494, -10.00128497722950804, 20.25080042701566541 ) ) ;
#18995=CARTESIAN_POINT ( 'NONE',  ( 19.07517029984344958, -22.84232114558952276, 19.66345542862526230 ) ) ;
#19028=CARTESIAN_POINT ( 'NONE',  ( -36.90241796781145922, -7.097865958168809719, 12.73282698324792328 ) ) ;
#19035=CARTESIAN_POINT ( 'NONE',  ( 6.176557290856084848, -13.77684855175925804, 22.99999999999999289 ) ) ;
#19036=CARTESIAN_POINT ( 'NONE',  ( -1.350289120986974551E-13, 38.03812643383474779, 16.87380292611441490 ) ) ;
#19041=CARTESIAN_POINT ( 'NONE',  ( -15.85745926894755620, 21.40218184478837316, 17.42190598798787349 ) ) ;
#19047=CARTESIAN_POINT ( 'NONE',  ( 32.09165771328279959, 1.123514972295850178, 13.32518128616608877 ) ) ;
#19052=DIRECTION ( 'NONE',  ( 0.000000000000000000, 0.000000000000000000, 1.000000000000000000 ) ) ;
#19063=CARTESIAN_POINT ( 'NONE',  ( -33.75875814100324845, 2.759858869446484064, 11.00000000000000000 ) ) ;
#19099=CARTESIAN_POINT ( 'NONE',  ( -1.911335737650684097, 40.16401087634231004, 13.32518128616608521 ) ) ;
#19103=CARTESIAN_POINT ( 'NONE',  ( 10.16357496796713100, 29.39421982382241438, 19.27171037444158230 ) ) ;
#19121=CARTESIAN_POINT ( 'NONE',  ( -32.40618899211658288, -4.990034233202359282, 17.92354375535250810 ) ) ;
#19139=EDGE_LOOP ( 'NONE', ( #282, #18214, #17286, #1397 ) ) ;
#19143=CARTESIAN_POINT ( 'NONE',  ( 20.92112759555548251, -16.07000418475261583, 20.99999999999999645 ) ) ;
#19144=CARTESIAN_POINT ( 'NONE',  ( 32.94198380406537296, -19.01906321691718205, 16.87380292611441490 ) ) ;
#19148=CARTESIAN_POINT ( 'NONE',  ( -3.003889247184246880, 27.48891118973640602, 20.99999999999988987 ) ) ;
#19154=CARTESIAN_POINT ( 'NONE',  ( 25.71480618106328109, 9.014447550977328305, 11.55979286844026532 ) ) ;
#19161=CARTESIAN_POINT ( 'NONE',  ( -22.33353841799275941, -20.81031336111065144, 20.25080042701592120 ) ) ;
#19190=CARTESIAN_POINT ( 'NONE',  ( 29.14609120334211667, -6.569533100115761748, 19.99202127657103389 ) ) ;
#19214=CARTESIAN_POINT ( 'NONE',  ( 37.51589702892714939, -12.89337557385784550, 11.00000000000017408 ) ) ;
#19223=CARTESIAN_POINT ( 'NONE',  ( -33.64699323788562424, -0.06984207429672421863, 12.14047268033065485 ) ) ;
#19230=CARTESIAN_POINT ( 'NONE',  ( 12.40052356344507523, 30.91160080447357927, 17.42190598798393353 ) ) ;
#19234=CARTESIAN_POINT ( 'NONE',  ( -15.87271492000489559, 26.91186955877756404, 15.72805884748939498 ) ) ;
#19240=CARTESIAN_POINT ( 'NONE',  ( 35.68447701591249910, -3.401722300707781255, 11.55979286843934872 ) ) ;
#19284=CARTESIAN_POINT ( 'NONE',  ( -25.38348611796302734, -5.460896781494596119, 20.69868183039781329 ) ) ;
#19292=CARTESIAN_POINT ( 'NONE',  ( 14.89626057892310307, 32.60452476689641088, 11.55979286843934872 ) ) ;
#19295=CARTESIAN_POINT ( 'NONE',  ( 9.991741549994847205, 30.98179641005372886, 18.87996532025785967 ) ) ;
#19302=DIRECTION ( 'NONE',  ( 1.000000000000000000, 0.000000000000000000, 0.000000000000000000 ) ) ;
#19316=CARTESIAN_POINT ( 'NONE',  ( -34.71804043165838038, -14.31680059899250068, 16.87380292611441135 ) ) ;
#19343=CARTESIAN_POINT ( 'NONE',  ( 22.28716212642845917, -26.62569406410656825, 16.87380292611434385 ) ) ;
#19345=CARTESIAN_POINT ( 'NONE',  ( 8.747212233148117022, 37.02488667719009641, 15.13084544680216759 ) ) ;
#19347=CARTESIAN_POINT ( 'NONE',  ( -3.998720052560664762, 27.76176938167515118, 20.94377226548378346 ) ) ;
#19353=CARTESIAN_POINT ( 'NONE',  ( 18.23687175285641260, 10.52906281568832902, 19.27171037444156809 ) ) ;
#19361=CARTESIAN_POINT ( 'NONE',  ( -28.10500220466552790, -8.168651434043027848, 20.50957957746051363 ) ) ;
#19387=CARTESIAN_POINT ( 'NONE',  ( 29.98847540738146122, -8.745685015162887765, 19.99202127657102324 ) ) ;
#19424=CARTESIAN_POINT ( 'NONE',  ( -15.12590024503300512, -28.14827041158709520, 13.92931973827808889 ) ) ;
#19431=CARTESIAN_POINT ( 'NONE',  ( -9.924110812759902700, 32.99075218357604200, 17.92354375535331101 ) ) ;
#19434=CARTESIAN_POINT ( 'NONE',  ( -21.61978140912946955, 6.167694920803358016, 18.87996532025794849 ) ) ;
#19437=CARTESIAN_POINT ( 'NONE',  ( 24.08873164041084536, -13.27722336041302320, 22.99999999999999645 ) ) ;
#19440=CARTESIAN_POINT ( 'NONE',  ( 24.63751168576237305, -28.54157386115114292, 12.14047268033101545 ) ) ;
#19448=ORIENTED_EDGE ( 'NONE', *, *, #9518, .T. ) ;
#19483=CARTESIAN_POINT ( 'NONE',  ( -32.33143948541737700, 1.358872982502395965, 11.55979286843935050 ) ) ;
#19497=CARTESIAN_POINT ( 'NONE',  ( -3.681484855442400672, 33.42880943655691084, 19.66345542862530138 ) ) ;
#19504=CARTESIAN_POINT ( 'NONE',  ( -25.71480618105494997, 9.014447550991285141, 11.00000000000190603 ) ) ;
#19518=CARTESIAN_POINT ( 'NONE',  ( -35.36447994912705184, -9.234655410424128519, 16.30093088680190405 ) ) ;
#19541=CARTESIAN_POINT ( 'NONE',  ( 20.67781403882192848, -27.68125770801123409, 15.72805884748939853 ) ) ;
#19543=CARTESIAN_POINT ( 'NONE',  ( 11.06388406389920753, 34.19581601475721300, 16.30093088680188274 ) ) ;
#19545=CARTESIAN_POINT ( 'NONE',  ( -4.137850160812051037, 25.30681243524895052, 20.99999999999999645 ) ) ;
#19553=CARTESIAN_POINT ( 'NONE',  ( 24.37528612859215471, 1.300641855011779979, 19.27171037445292257 ) ) ;
#19563=CARTESIAN_POINT ( 'NONE',  ( -31.11751153274386184, -7.091459469499522328, 19.27171037444191271 ) ) ;
#19589=CARTESIAN_POINT ( 'NONE',  ( 25.09931006221244942, -21.40067874915650137, 19.66345542862496387 ) ) ;
#19596=EDGE_CURVE ( 'NONE', #36229, #10557, #9271, .T. ) ;
#19623=CARTESIAN_POINT ( 'NONE',  ( -36.93643098903786637, -14.76343610888389257, 12.73282698324853079 ) ) ;
#19632=CARTESIAN_POINT ( 'NONE',  ( -4.583318357746721361, 36.10598097934249040, 17.92354375535251521 ) ) ;
#19635=CARTESIAN_POINT ( 'NONE',  ( -15.65370567419120640, 2.019989953599362842, 20.99999999999999645 ) ) ;
#19637=CARTESIAN_POINT ( 'NONE',  ( 24.22138565352628348, -9.557272464391640909, 20.99999999999999645 ) ) ;
#19641=CARTESIAN_POINT ( 'NONE',  ( 16.88398162953626525, -29.10422986782303667, 12.14047268032943805 ) ) ;
#19653=CARTESIAN_POINT ( 'NONE',  ( 30.33933116650763040, 6.243556997736084746, 11.00000000000000000 ) ) ;
#19698=CARTESIAN_POINT ( 'NONE',  ( 7.591957726968924014, 38.93640765974104312, 10.99999999999980638 ) ) ;
#19700=CARTESIAN_POINT ( 'NONE',  ( 8.859192577249615397, 12.20922670554002565, 20.99999999999999645 ) ) ;
#19702=ADVANCED_BREP_SHAPE_REPRESENTATION ( '', ( #8826, #24238 ), #31997 ) ;
#19703=CARTESIAN_POINT ( 'NONE',  ( -1.248251703783856303, 34.03222469610383172, 19.66345542862528362 ) ) ;
#19725=CARTESIAN_POINT ( 'NONE',  ( -15.60391421430763437, -26.29546805949255983, 16.87380292611441490 ) ) ;
#19736=ORIENTED_EDGE ( 'NONE', *, *, #17283, .F. ) ;
#19748=CARTESIAN_POINT ( 'NONE',  ( 31.31527935466855439, -1.911037205180780019, 17.42190598798589107 ) ) ;
#19750=CARTESIAN_POINT ( 'NONE',  ( 9.684793793941290474, 35.24386573278109580, 16.30093088680190405 ) ) ;
#19752=CARTESIAN_POINT ( 'NONE',  ( 5.469228652589973372, 26.20992143183299916, 20.94377226548378701 ) ) ;
#19758=CARTESIAN_POINT ( 'NONE',  ( 22.71318823113102070, 6.927825590551851320, 17.92354375535233046 ) ) ;
#19764=( BOUNDED_CURVE ( )  B_SPLINE_CURVE ( 2, ( #39869, #12046, #36829 ),
 .UNSPECIFIED., .F., .F. ) 
 B_SPLINE_CURVE_WITH_KNOTS ( ( 3, 3 ),
 ( 0.000000000000000000, 1.000000000000000000 ),
 .UNSPECIFIED. ) 
 CURVE ( )  GEOMETRIC_REPRESENTATION_ITEM ( )  RATIONAL_B_SPLINE_CURVE ( ( 1.000000000000000000, 0.7071067811865475727, 1.000000000000000000 ) ) 
 REPRESENTATION_ITEM ( '' )  );
#19770=CARTESIAN_POINT ( 'NONE',  ( -28.04602290581260959, -19.07745245555469893, 19.66345542862529783 ) ) ;
#19796=CARTESIAN_POINT ( 'NONE',  ( 17.00801676779564886, -20.85310720624810088, 20.25080042701566541 ) ) ;
#19834=CARTESIAN_POINT ( 'NONE',  ( -34.83527399001564362, -1.648960735037901637, 10.99999999999971045 ) ) ;
#19844=CARTESIAN_POINT ( 'NONE',  ( -14.43694901005348719, 26.51279404187317112, 17.42190598798392642 ) ) ;
#19855=CARTESIAN_POINT ( 'NONE',  ( 36.74707368630884474, -16.71203845619544026, 11.55979286843918885 ) ) ;
#19904=CARTESIAN_POINT ( 'NONE',  ( -10.89111091687339083, 36.83121428896948402, 10.99999999999999467 ) ) ;
#19907=CARTESIAN_POINT ( 'NONE',  ( -2.974899668820556009, 35.98612526451936589, 18.42518152272109688 ) ) ;
#19928=CARTESIAN_POINT ( 'NONE',  ( -35.60445263620085399, -7.407141432649139823, 15.72805884748857963 ) ) ;
#19952=CARTESIAN_POINT ( 'NONE',  ( 15.27443809245941786, -27.57253143578273935, 15.13084544680213561 ) ) ;
#19955=CARTESIAN_POINT ( 'NONE',  ( 12.27396990952286160, 32.91879577929221057, 16.30093088680193958 ) ) ;
#19957=CARTESIAN_POINT ( 'NONE',  ( 16.80389827882579112, -21.64427909826065743, 19.99202127657103389 ) ) ;
#19959=CARTESIAN_POINT ( 'NONE',  ( -7.164929079094340736, 24.49151390636721715, 20.82122704794079837 ) ) ;
#19964=CARTESIAN_POINT ( 'NONE',  ( 12.55429062394625994, 25.98950339721545788, 18.87996532025784546 ) ) ;
#19976=CARTESIAN_POINT ( 'NONE',  ( -23.94831201522144326, -21.88372720616936817, 19.66345542862529072 ) ) ;
#19982=ORIENTED_EDGE ( 'NONE', *, *, #6115, .T. ) ;
#19997=CARTESIAN_POINT ( 'NONE',  ( -20.38753357181594694, -16.19769905861803139, 23.00000000000000000 ) ) ;
#20001=CARTESIAN_POINT ( 'NONE',  ( 31.83642866623112511, -11.02236948596282140, 19.27171037444156099 ) ) ;
#20002=EDGE_CURVE ( 'NONE', #8296, #17265, #11676, .T. ) ;
#20026=CARTESIAN_POINT ( 'NONE',  ( 14.98890121934609532, -28.67928442654220333, 11.00000000000000000 ) ) ;
#20027=EDGE_CURVE ( 'NONE', #7799, #32321, #14393, .T. ) ;
#20037=CARTESIAN_POINT ( 'NONE',  ( -15.00437666251166746, -28.61930095463374712, 12.14047268033097460 ) ) ;
#20051=CARTESIAN_POINT ( 'NONE',  ( -7.164929079095160525, 24.49151390636425418, 20.82122704794079837 ) ) ;
#20053=CARTESIAN_POINT ( 'NONE',  ( 18.23649648353767461, -16.09146789626181118, 20.99999999999999645 ) ) ;
#20054=CARTESIAN_POINT ( 'NONE',  ( 18.76090689389210198, -16.22676322417229500, 20.99999999999999289 ) ) ;
#20059=CARTESIAN_POINT ( 'NONE',  ( 35.50541758542747317, -3.488475578028298774, 12.73282698324852724 ) ) ;
#20062=DIRECTION ( 'NONE',  ( -1.000000000000000000, 0.000000000000000000, 0.000000000000000000 ) ) ;
#20085=CARTESIAN_POINT ( 'NONE',  ( -24.37697481792950782, -10.07885229508464953, 23.00000000000000355 ) ) ;
#20103=EDGE_CURVE ( 'NONE', #31697, #10973, #14316, .T. ) ;
#20109=CARTESIAN_POINT ( 'NONE',  ( -17.34253826607185900, 27.32041144404031030, 11.00000000000000000 ) ) ;
#20113=CARTESIAN_POINT ( 'NONE',  ( -5.791386747369965171, 35.03736185296623518, 18.42518152272108978 ) ) ;
#20115=EDGE_LOOP ( 'NONE', ( #16786, #8632, #35831, #22218 ) ) ;
#20124=CARTESIAN_POINT ( 'NONE',  ( 12.28720923547795429, -14.55658080553756584, 20.99999999999999645 ) ) ;
#20133=CARTESIAN_POINT ( 'NONE',  ( -32.79363849989120894, -0.7437118703953984333, 15.13084544680199883 ) ) ;
#20154=CARTESIAN_POINT ( 'NONE',  ( 31.71434132860828470, -22.43226626708964133, 15.72805884748975203 ) ) ;
#20156=CARTESIAN_POINT ( 'NONE',  ( 12.63299342935012959, 33.22349594678088636, 15.72805884748943939 ) ) ;
#20159=CARTESIAN_POINT ( 'NONE',  ( 16.41753675003788615, -23.14183271658374608, 19.27171037444156454 ) ) ;
#20161=CARTESIAN_POINT ( 'NONE',  ( -3.137032374298060589, 29.29040802067846982, 20.82122704794080192 ) ) ;
#20169=CARTESIAN_POINT ( 'NONE',  ( 15.87271491999413264, 26.91186955881611809, 15.72805884748939853 ) ) ;
#20178=CARTESIAN_POINT ( 'NONE',  ( -28.20105441993478834, -17.62361288429907802, 19.99202127657073191 ) ) ;
#20187=CARTESIAN_POINT ( 'NONE',  ( -4.817371740575545402, 23.83900317890010001, 23.00000000000000000 ) ) ;
#20193=CARTESIAN_POINT ( 'NONE',  ( 19.30730118283910457, -16.27608008926517513, 23.00000000000000000 ) ) ;
#20203=CARTESIAN_POINT ( 'NONE',  ( 28.60197298177003589, -19.58586899272799187, 19.27171037444191271 ) ) ;
#20228=CARTESIAN_POINT ( 'NONE',  ( -24.37759566069507855, -10.08322588119029817, 20.99999999999999645 ) ) ;
#20241=CARTESIAN_POINT ( 'NONE',  ( -37.07075634848843038, -14.79048025366256169, 12.14047268033097282 ) ) ;
#20253=CARTESIAN_POINT ( 'NONE',  ( -25.98021325959403072, -4.875178728618521973, 20.50957957746029336 ) ) ;
#20254=CARTESIAN_POINT ( 'NONE',  ( 26.04175756481604509, -10.41789154269857320, 20.94377226548378346 ) ) ;
#20293=EDGE_LOOP ( 'NONE', ( #1004, #30696, #4948, #37811, #28828, #3141 ) ) ;
#20313=CARTESIAN_POINT ( 'NONE',  ( 3.110808594360203738, 36.60201144129485584, 17.92354375535251876 ) ) ;
#20328=CARTESIAN_POINT ( 'NONE',  ( 18.03924190088524782, -16.85603499720511422, 20.99999999999998934 ) ) ;
#20336=CARTESIAN_POINT ( 'NONE',  ( -34.65585262756959395, -3.900084976043918239, 15.13084544680213561 ) ) ;
#20359=CARTESIAN_POINT ( 'NONE',  ( 31.24272016125166829, 0.2902395683485590738, 15.72805884748940031 ) ) ;
#20363=CARTESIAN_POINT ( 'NONE',  ( 17.01882136418227986, 27.23043334310844443, 13.32518128616608877 ) ) ;
#20365=CARTESIAN_POINT ( 'NONE',  ( 10.51283450065148273, -24.98199432654207897, 16.87380292611226551 ) ) ;
#20367=CARTESIAN_POINT ( 'NONE',  ( 6.978241445790387409, 28.42397159967988429, 20.50957957746029336 ) ) ;
#20375=CARTESIAN_POINT ( 'NONE',  ( 9.576215452290895769, 12.54651180042800718, 20.99999999999999645 ) ) ;
#20384=CARTESIAN_POINT ( 'NONE',  ( -30.13477841296696269, -9.898407001806557304, 19.99202127657103389 ) ) ;
#20404=CARTESIAN_POINT ( 'NONE',  ( -37.88915195766744404, -19.37406375362002464, 23.00000000000093792 ) ) ;
#20409=CARTESIAN_POINT ( 'NONE',  ( 27.04163063101144715, -21.95895612274795283, 18.87996532025750795 ) ) ;
#20422=CARTESIAN_POINT ( 'NONE',  ( -1.829593030691901284E-15, 22.50000000000001066, 23.00000000000000000 ) ) ;
#20431=CARTESIAN_POINT ( 'NONE',  ( -23.74914942275198015, -8.582573258223680668, 20.99999999999999645 ) ) ;
#20442=CARTESIAN_POINT ( 'NONE',  ( -31.38526299860031088, -24.75545609243350853, 11.00000000000000000 ) ) ;
#20458=CARTESIAN_POINT ( 'NONE',  ( -6.462764152204137247, 17.91932574235844555, 20.99999999999999645 ) ) ;
#20459=CARTESIAN_POINT ( 'NONE',  ( 24.20198940123945519, -6.620595927254128377, 20.94377226548378346 ) ) ;
#20460=CARTESIAN_POINT ( 'NONE',  ( 19.30730118283910812, -16.27608008926517869, 20.99999999999999645 ) ) ;
#20522=CARTESIAN_POINT ( 'NONE',  ( -2.113580199870562559, 27.06415334822006002, 23.00000000000000355 ) ) ;
#20535=CARTESIAN_POINT ( 'NONE',  ( -34.36758591766905369, -1.941406924250941302, 13.92931973827763059 ) ) ;
#20558=CARTESIAN_POINT ( 'NONE',  ( 34.64424588159074148, -17.94331620955155771, 15.72805884748941097 ) ) ;
#20560=CARTESIAN_POINT ( 'NONE',  ( 15.23841289164144541, 30.59360923276694777, 14.53008259254005985 ) ) ;
#20562=CARTESIAN_POINT ( 'NONE',  ( -5.531500846456688159, -21.05812563137664739, 19.27171037444156809 ) ) ;
#20566=CARTESIAN_POINT ( 'NONE',  ( -6.700679222775207610E-14, 30.76432767446199534, 20.69868183039781329 ) ) ;
#20575=CARTESIAN_POINT ( 'NONE',  ( 23.18043107533613068, 0.3100950997233969386, 19.99202127658098505 ) ) ;
#20586=CARTESIAN_POINT ( 'NONE',  ( -20.42855823444361363, -24.24606183460709374, 18.87996532025784902 ) ) ;
#20601=CARTESIAN_POINT ( 'NONE',  ( 20.92112759555542922, -16.07000418475249859, 23.00000000000000000 ) ) ;
#20611=CARTESIAN_POINT ( 'NONE',  ( 29.77271197308713724, -3.128983846829581861, 18.87996532025967511 ) ) ;
#20617=CARTESIAN_POINT ( 'NONE',  ( -15.27443809246124218, -27.57253143578281041, 15.13084544680213739 ) ) ;
#20632=CARTESIAN_POINT ( 'NONE',  ( -10.09822582592804174, -27.41751403069116222, 11.55979286845328069 ) ) ;
#20635=CARTESIAN_POINT ( 'NONE',  ( -23.81569860407211436, -13.74999999999980105, 20.99999999999999645 ) ) ;
#20645=CARTESIAN_POINT ( 'NONE',  ( -35.07402885326978037, -20.24999999999986855, 11.55979286843934872 ) ) ;
#20662=CARTESIAN_POINT ( 'NONE',  ( 24.42249384534429169, -8.161410322277701468, 21.00000000000004619 ) ) ;
#20720=CARTESIAN_POINT ( 'NONE',  ( 28.79337657215624446, 4.963436916936688093, 10.99999999998960831 ) ) ;
#20740=CARTESIAN_POINT ( 'NONE',  ( -34.08416769313322447, -19.67850339273479676, 15.13084544680213561 ) ) ;
#20744=ADVANCED_FACE ( 'NONE', ( #2833 ), #29619, .T. ) ;
#20762=CARTESIAN_POINT ( 'NONE',  ( 30.82617745331448944, -24.12092658898442110, 14.53008259254011492 ) ) ;
#20764=CARTESIAN_POINT ( 'NONE',  ( 3.717128218779132798, 39.34929362537322817, 14.53008259254021439 ) ) ;
#20765=CARTESIAN_POINT ( 'NONE',  ( -17.42101839919755690, -19.25229542401750038, 20.69868183039781329 ) ) ;
#20768=CARTESIAN_POINT ( 'NONE',  ( 7.164929079093869113, 24.49151390636890824, 20.82122704794079837 ) ) ;
#20776=CARTESIAN_POINT ( 'NONE',  ( 13.32472804388164000, 14.30980730578316873, 20.25080042701575778 ) ) ;
#20785=CARTESIAN_POINT ( 'NONE',  ( -16.23042486173915933, -23.86708630543300202, 18.87996532025784546 ) ) ;
#20799=CARTESIAN_POINT ( 'NONE',  ( 18.76090689389208066, -16.22676322417240868, 23.00000000000000000 ) ) ;
#20808=CARTESIAN_POINT ( 'NONE',  ( 21.83515197098677163, -24.14400021536937047, 18.87996532025784546 ) ) ;
#20830=CARTESIAN_POINT ( 'NONE',  ( 15.00437666251164792, -28.61930095463398160, 12.14047268033097460 ) ) ;
#20833=CARTESIAN_POINT ( 'NONE',  ( -24.85114452701394328, -15.17411596029591969, 20.94377226548368398 ) ) ;
#20852=VECTOR ( 'NONE', #6546, 1000.000000000000000 ) ;
#20860=CARTESIAN_POINT ( 'NONE',  ( 24.40183261524840574, -16.82966968839916433, 20.82122704794079837 ) ) ;
#20886=CARTESIAN_POINT ( 'NONE',  ( 25.38348611796500975, -5.460896781496693109, 20.69868183039781329 ) ) ;
#20897=EDGE_LOOP ( 'NONE', ( #4649, #30539, #14530, #5485 ) ) ;
#20923=CARTESIAN_POINT ( 'NONE',  ( -1.082972213713690346, 27.41125570341915463, 23.00000000000000000 ) ) ;
#20949=VERTEX_POINT ( 'NONE', #36120 ) ;
#20951=CARTESIAN_POINT ( 'NONE',  ( 36.96658581397633014, -12.84323481469944994, 13.92931973827817238 ) ) ;
#20953=CARTESIAN_POINT ( 'NONE',  ( -8.901509289504682343, 37.28103075694416901, 14.53008259253942924 ) ) ;
#20956=CARTESIAN_POINT ( 'NONE',  ( -2.148627388802350158, 32.24135036777339991, 20.25080042701565475 ) ) ;
#20968=CARTESIAN_POINT ( 'NONE',  ( 16.32868373051637079, 2.489249428701628464, 20.94377226548377280 ) ) ;
#20970=CARTESIAN_POINT ( 'NONE',  ( 3.900486991066248077, 40.17991855518007327, 11.00000000000019718 ) ) ;
#20978=CARTESIAN_POINT ( 'NONE',  ( -17.59613548593113208, -24.21943298483451201, 18.87996532025787033 ) ) ;
#20993=CARTESIAN_POINT ( 'NONE',  ( 24.37759566069541250, -10.08322588119074936, 23.00000000000000000 ) ) ;
#20998=CARTESIAN_POINT ( 'NONE',  ( -29.22254794994711702, -28.85350742528316204, 11.00000000000000000 ) ) ;
#21004=CARTESIAN_POINT ( 'NONE',  ( 31.65150718622346915, -20.14649908112952303, 17.42190598798391932 ) ) ;
#21010=CARTESIAN_POINT ( 'NONE',  ( -16.05557028316514945, -24.54483004364972132, 18.42518152272108978 ) ) ;
#21012=EDGE_CURVE ( 'NONE', #23396, #8563, #26545, .T. ) ;
#21023=CARTESIAN_POINT ( 'NONE',  ( 4.234589283516844012E-14, -26.22849730612247754, 13.92931973827808712 ) ) ;
#21027=CARTESIAN_POINT ( 'NONE',  ( -26.04175756481620496, -10.41789154269907058, 20.94377226548378346 ) ) ;
#21040=CARTESIAN_POINT ( 'NONE',  ( -19.30730118283921470, -16.27608008926401340, 21.00000000000001421 ) ) ;
#21054=CARTESIAN_POINT ( 'NONE',  ( 25.74508523780477987, -9.012467239717258494, 20.94377226548369819 ) ) ;
#21056=CARTESIAN_POINT ( 'NONE',  ( 32.84658669524301189, -23.46788009898371641, 10.99999999999997335 ) ) ;
#21057=VECTOR ( 'NONE', #13498, 1000.000000000000000 ) ;
#21080=CARTESIAN_POINT ( 'NONE',  ( 32.33143948541787438, 1.358872982501792226, 11.00000000000000000 ) ) ;
#21095=CARTESIAN_POINT ( 'NONE',  ( -20.48347041321339290, 17.67745015982535861, 12.73282698324691609 ) ) ;
#21148=CARTESIAN_POINT ( 'NONE',  ( 33.43067318719201353, -0.2406684815405015221, 13.32518128616727537 ) ) ;
#21150=CARTESIAN_POINT ( 'NONE',  ( 5.571153519068981375, 39.03845596069754009, 13.92931973827808889 ) ) ;
#21151=CARTESIAN_POINT ( 'NONE',  ( 4.309332716386178631E-14, -16.21345324574345170, 20.82122704794080192 ) ) ;
#21153=CARTESIAN_POINT ( 'NONE',  ( 3.166027244385917427, 31.89862848374664495, 20.25080042701565830 ) ) ;
#21156=EDGE_CURVE ( 'NONE', #31697, #8563, #25295, .T. ) ;
#21164=CARTESIAN_POINT ( 'NONE',  ( 17.69280599716815416, 3.437614796730258160, 20.69868183039776710 ) ) ;
#21175=CARTESIAN_POINT ( 'NONE',  ( -31.82689352098154600, -6.837796194681720507, 18.87996532025821850 ) ) ;
#21194=CARTESIAN_POINT ( 'NONE',  ( -37.88915195766834643, -19.37406375362053979, 11.00000000000000000 ) ) ;
#21196=EDGE_LOOP ( 'NONE', ( #5061, #19736, #31440, #30642 ) ) ;
#21200=CARTESIAN_POINT ( 'NONE',  ( 17.40362039086722135, -25.54020003774037662, 17.92354375535206756 ) ) ;
#21204=CARTESIAN_POINT ( 'NONE',  ( 3.025308588020339862, 26.48089285804714876, 20.99999999999999645 ) ) ;
#21218=CARTESIAN_POINT ( 'NONE',  ( 5.078902502065831825, -26.44091005802452798, 13.32518128616608877 ) ) ;
#21222=CARTESIAN_POINT ( 'NONE',  ( -17.62780868050729666, -18.45076755199299257, 20.82122704794079837 ) ) ;
#21248=CARTESIAN_POINT ( 'NONE',  ( 22.09885373566428868, -20.02268770624830552, 20.50957957746051719 ) ) ;
#21262=CARTESIAN_POINT ( 'NONE',  ( 17.01882136418227986, 27.23043334310844799, 13.32518128616608877 ) ) ;
#21275=CARTESIAN_POINT ( 'NONE',  ( 29.28423149095877420, -1.632116715646417138, 18.42518152272108622 ) ) ;
#21280=CARTESIAN_POINT ( 'NONE',  ( 38.66460482429456391, -17.32098562631985672, 11.00000000000000178 ) ) ;
#21291=VERTEX_POINT ( 'NONE', #7010 ) ;
#21294=AXIS2_PLACEMENT_3D ( 'NONE', #18892, #3050, #27834 ) ;
#21295=CARTESIAN_POINT ( 'NONE',  ( -20.16616670141840828, 17.52816929147905967, 13.92931973827678682 ) ) ;
#21304=B_SPLINE_CURVE_WITH_KNOTS ( 'NONE', 3,
 ( #3988, #17205, #13734, #952, #16390, #29582, #32231, #10904, #22873, #23291, #28776, #26125, #25723, #1760, #35076, #13534, #25519, #37920 ),
 .UNSPECIFIED., .F., .F.,
 ( 4, 2, 2, 2, 2, 2, 2, 2, 4 ),
 ( 0.000000000000000000, 0.1250000000000000278, 0.2500000000000000555, 0.3750000000000001110, 0.5000000000000000000, 0.6250000000000000000, 0.7500000000000000000, 0.8750000000000001110, 1.000000000000000000 ),
 .UNSPECIFIED. ) ;
#21306=CARTESIAN_POINT ( 'NONE',  ( 32.33143948541787438, 1.358872982501792226, 11.00000000000000000 ) ) ;
#21310=CYLINDRICAL_SURFACE ( 'NONE', #4520, 60.00000000000007816 ) ;
#21317=CARTESIAN_POINT ( 'NONE',  ( 2.590671895605813901, 26.81128010880988199, 23.00000000000000355 ) ) ;
#21322=EDGE_CURVE ( 'NONE', #20949, #17265, #17269, .T. ) ;
#21327=DIRECTION ( 'NONE',  ( -1.000000000000000000, 0.000000000000000000, 0.000000000000000000 ) ) ;
#21338=EDGE_CURVE ( 'NONE', #10384, #3967, #14153, .T. ) ;
#21350=ORIENTED_EDGE ( 'NONE', *, *, #11909, .F. ) ;
#21353=CARTESIAN_POINT ( 'NONE',  ( -10.68781676061691854, 36.56370694841923807, 13.32518128616608699 ) ) ;
#21354=CARTESIAN_POINT ( 'NONE',  ( -11.59681349794144012, -18.61320969085484833, 20.50957957746048521 ) ) ;
#21356=CARTESIAN_POINT ( 'NONE',  ( 5.569982264780531267, 31.74975025675623286, 19.99202127657103745 ) ) ;
#21373=CARTESIAN_POINT ( 'NONE',  ( -29.73172958077499572, -1.192874570366647458, 17.92354375535250810 ) ) ;
#21385=CARTESIAN_POINT ( 'NONE',  ( 39.05366788733209660, -6.582903524762724778, 22.99999999999999289 ) ) ;
#21397=CARTESIAN_POINT ( 'NONE',  ( 29.73172958077661931, -1.192874570368608333, 17.92354375535250810 ) ) ;
#21403=CARTESIAN_POINT ( 'NONE',  ( -17.42101839920251649, -19.25229542401852001, 20.69868183039780618 ) ) ;
#21410=ADVANCED_FACE ( 'NONE', ( #10473 ), #12262, .F. ) ;
#21418=CARTESIAN_POINT ( 'NONE',  ( -26.93475362026834219, -11.92845428170184974, 20.82122704794080192 ) ) ;
#21435=EDGE_CURVE ( 'NONE', #8296, #8510, #11205, .T. ) ;
#21445=CARTESIAN_POINT ( 'NONE',  ( 25.82695510740672162, -7.282951130326176248, 20.82122704794095114 ) ) ;
#21462=CARTESIAN_POINT ( 'NONE',  ( -9.762440214458996124, -29.39637225280792521, 22.99999999999999645 ) ) ;
#21472=CARTESIAN_POINT ( 'NONE',  ( 32.33143948541893309, 1.358872982500733961, 11.55979286843934695 ) ) ;
#21477=CARTESIAN_POINT ( 'NONE',  ( -24.32690616642468839, -27.49953951067762148, 15.13084544680243049 ) ) ;
#21488=CARTESIAN_POINT ( 'NONE',  ( -17.15083734909836011, 27.26712758904658784, 12.73282698324853257 ) ) ;
#21491=CARTESIAN_POINT ( 'NONE',  ( 18.76532695907111403, -16.22790357942847805, 22.99999999999999289 ) ) ;
#21500=FACE_OUTER_BOUND ( 'NONE', #23953, .T. ) ;
#21515=CARTESIAN_POINT ( 'NONE',  ( 1.082972213713614407, 27.41125570341915818, 23.00000000000000000 ) ) ;
#21544=CARTESIAN_POINT ( 'NONE',  ( -15.81288461013852498, 30.89878388227737105, 12.73282698324828743 ) ) ;
#21545=CARTESIAN_POINT ( 'NONE',  ( 6.077490221915134327, -14.56650175400723946, 20.99999999999999645 ) ) ;
#21547=CARTESIAN_POINT ( 'NONE',  ( 7.604809270644918406, 28.95580224300140770, 20.25080042701566541 ) ) ;
#21568=CARTESIAN_POINT ( 'NONE',  ( -32.94198380406523796, -19.01906321691725310, 16.87380292611441845 ) ) ;
#21591=CARTESIAN_POINT ( 'NONE',  ( 30.60828605274730663, -21.42068866017963913, 17.42190598798431012 ) ) ;
#21602=CARTESIAN_POINT ( 'NONE',  ( 22.71454497019403362, 13.11424865306083731, 13.92931973827808889 ) ) ;
#21613=CARTESIAN_POINT ( 'NONE',  ( -17.21213525677265821, -20.06193531423681620, 20.50957957746029692 ) ) ;
#21641=CARTESIAN_POINT ( 'NONE',  ( 25.38348611796611110, -5.460896781497905472, 20.69868183039781329 ) ) ;
#21657=PRESENTATION_STYLE_ASSIGNMENT (( #16166 ) ) ;
#21675=CARTESIAN_POINT ( 'NONE',  ( -36.22115687806137174, -16.54570019420447835, 13.92931973827825409 ) ) ;
#21687=CARTESIAN_POINT ( 'NONE',  ( -31.51573171626090897, 0.5582143012903738599, 15.13084544680213561 ) ) ;
#21696=EDGE_LOOP ( 'NONE', ( #39862, #31122, #36071, #22516 ) ) ;
#21714=CARTESIAN_POINT ( 'NONE',  ( 2.109373541296217347, 27.06550157850341876, 23.00000000000000000 ) ) ;
#21741=CARTESIAN_POINT ( 'NONE',  ( -13.65031603318048070, 34.08687889766149226, 12.73282698324877238 ) ) ;
#21744=CARTESIAN_POINT ( 'NONE',  ( 9.535948996435982039, 27.56441102001909016, 19.99202127657104100 ) ) ;
#21748=CARTESIAN_POINT ( 'NONE',  ( -14.43694901005348719, 26.51279404187317468, 17.42190598798392642 ) ) ;
#21764=CARTESIAN_POINT ( 'NONE',  ( -17.40362039086605250, -25.54020003774204639, 17.92354375535249034 ) ) ;
#21771=CARTESIAN_POINT ( 'NONE',  ( 10.09822582592851425, -27.41751403068707660, 11.00000000000204992 ) ) ;
#21778=CARTESIAN_POINT ( 'NONE',  ( 4.817371740575539185, 23.83900317890011422, 20.99999999999999645 ) ) ;
#21779=CARTESIAN_POINT ( 'NONE',  ( 19.48557158514982746, -11.25000000000009415, 2.999999999999999112 ) ) ;
#21786=CARTESIAN_POINT ( 'NONE',  ( 24.37759566069541961, -10.08322588119077423, 21.00000000000001776 ) ) ;
#21787=CARTESIAN_POINT ( 'NONE',  ( 33.27313359469018650, -17.33775975077022480, 17.42190598798393353 ) ) ;
#21811=CARTESIAN_POINT ( 'NONE',  ( -20.97603028425659843, -19.42790760331400790, 20.69868183039763565 ) ) ;
#21837=CARTESIAN_POINT ( 'NONE',  ( -39.48557158816404211, -12.76940457902596471, 10.99999999999999645 ) ) ;
#21838=CARTESIAN_POINT ( 'NONE',  ( 26.77583779507883222, -12.71777209950087340, 20.82122704794080903 ) ) ;
#21853=B_SPLINE_CURVE_WITH_KNOTS ( 'NONE', 3,
 ( #4672, #22746, #19504, #38800, #29052, #23364 ),
 .UNSPECIFIED., .F., .F.,
 ( 4, 2, 4 ),
 ( 0.000000000000000000, 0.5000000000000000000, 1.000000000000000000 ),
 .UNSPECIFIED. ) ;
#21867=ORIENTED_EDGE ( 'NONE', *, *, #36950, .T. ) ;
#21870=CARTESIAN_POINT ( 'NONE',  ( -16.99774364072496979, -28.32416636927843001, 14.53008259253979517 ) ) ;
#21880=CARTESIAN_POINT ( 'NONE',  ( -22.19651343352304806, 6.568638172588403989, 18.42518152272124965 ) ) ;
#21889=CARTESIAN_POINT ( 'NONE',  ( 16.95459465864674442, -28.62006465032575164, 13.92931973827687919 ) ) ;
#21893=ADVANCED_FACE ( 'NONE', ( #32789, #32994 ), #17351, .F. ) ;
#21908=CARTESIAN_POINT ( 'NONE',  ( 19.26948696230205016, 27.85601271560038228, 11.00000000000000000 ) ) ;
#21936=LINE ( 'NONE', #6098, #6643 ) ;
#21943=CARTESIAN_POINT ( 'NONE',  ( 13.75541765477348655, 34.17602237659296094, 12.14047268033109184 ) ) ;
#21948=CARTESIAN_POINT ( 'NONE',  ( -9.417362331747755277, 30.49429905890304937, 19.27171037444153612 ) ) ;
#21968=CARTESIAN_POINT ( 'NONE',  ( -23.60877407455476984, -25.08990816560874038, 17.92354375535287403 ) ) ;
#21990=CARTESIAN_POINT ( 'NONE',  ( 31.36686156446545581, -22.11446460981255058, 16.30093088680227709 ) ) ;
#22003=CARTESIAN_POINT ( 'NONE',  ( 25.43795106045698518, 8.821996438889113890, 13.32518128616659148 ) ) ;
#22013=CARTESIAN_POINT ( 'NONE',  ( -27.85940672053882849, -14.94704994757599081, 20.50957957746051719 ) ) ;
#22014=CARTESIAN_POINT ( 'NONE',  ( -19.48557158514998022, -11.24999999999982414, 2.999999999999999112 ) ) ;
#22040=CARTESIAN_POINT ( 'NONE',  ( 27.57147631791876918, -9.321847555861369372, 20.69868183039781329 ) ) ;
#22070=CARTESIAN_POINT ( 'NONE',  ( -33.75875814100331951, 2.759858869446532470, 23.00000000000000000 ) ) ;
#22072=CARTESIAN_POINT ( 'NONE',  ( -18.85754271145797034, -29.00601859117224990, 13.32518128616650799 ) ) ;
#22080=CARTESIAN_POINT ( 'NONE',  ( -6.055828121133336239, 35.60995051739008943, 17.92354375535250810 ) ) ;
#22085=CARTESIAN_POINT ( 'NONE',  ( -13.83280510892634929, 26.34487040056601970, 17.92354375535250810 ) ) ;
#22093=CARTESIAN_POINT ( 'NONE',  ( 26.32119069355270113, -27.53777429989680670, 13.32518128616608521 ) ) ;
#22098=CARTESIAN_POINT ( 'NONE',  ( 15.00309677617812554, 1.567672476142359050, 23.00000000000000000 ) ) ;
#22111=CARTESIAN_POINT ( 'NONE',  ( -13.82587226055958851, 37.11292026377127229, 23.00000000000187583 ) ) ;
#22141=CARTESIAN_POINT ( 'NONE',  ( 7.508063977623086416, 38.75471409550124235, 12.73282698324837803 ) ) ;
#22143=CARTESIAN_POINT ( 'NONE',  ( -8.842909878189049167, 12.23753042740625752, 23.00000000000000355 ) ) ;
#22144=CARTESIAN_POINT ( 'NONE',  ( 8.843001881758423721, 30.00677403926963294, 19.66345542862529783 ) ) ;
#22157=CARTESIAN_POINT ( 'NONE',  ( -4.817371740575545402, 23.83900317890010001, 20.99999999999999645 ) ) ;
#22161=CARTESIAN_POINT ( 'NONE',  ( -26.77946264071690052, -24.43926981373589058, 17.42190598798356049 ) ) ;
#22163=EDGE_CURVE ( 'NONE', #3967, #27076, #8295, .T. ) ;
#22171=CARTESIAN_POINT ( 'NONE',  ( 14.98890121934609532, -28.67928442654220333, 11.00000000000000000 ) ) ;
#22184=CARTESIAN_POINT ( 'NONE',  ( 27.27686897040210212, -25.33890797347431700, 16.30093088680153102 ) ) ;
#22189=CARTESIAN_POINT ( 'NONE',  ( -0.5415361484147104276, 27.50000000000004263, 20.99999999999998934 ) ) ;
#22194=CARTESIAN_POINT ( 'NONE',  ( 17.34253826607094240, 27.32041144404343314, 11.55979286843934872 ) ) ;
#22203=CARTESIAN_POINT ( 'NONE',  ( -25.23650320482248333, -19.40090744331417127, 20.25080042701566185 ) ) ;
#22218=ORIENTED_EDGE ( 'NONE', *, *, #5820, .T. ) ;
#22228=CARTESIAN_POINT ( 'NONE',  ( 25.23650320482206055, -19.40090744331450878, 20.25080042701540961 ) ) ;
#22249=ORIENTED_EDGE ( 'NONE', *, *, #15295, .F. ) ;
#22263=CARTESIAN_POINT ( 'NONE',  ( -20.77381726376759019, -29.00435581194061641, 12.73282698324853257 ) ) ;
#22271=CARTESIAN_POINT ( 'NONE',  ( -13.41665185498830937, 27.84207739517983171, 17.92354375535208888 ) ) ;
#22276=CARTESIAN_POINT ( 'NONE',  ( -28.25018339770460685, -2.647087534799629438, 19.27171037444156809 ) ) ;
#22280=CARTESIAN_POINT ( 'NONE',  ( 24.49503443140846315, -11.70166252807803176, 23.00000000000000000 ) ) ;
#22286=CARTESIAN_POINT ( 'NONE',  ( 24.59814121633610640, -28.40949844211205644, 12.73282698324863738 ) ) ;
#22291=CARTESIAN_POINT ( 'NONE',  ( 33.75875814100320582, 2.759858869446452534, 22.99999999999999645 ) ) ;
#22336=CARTESIAN_POINT ( 'NONE',  ( 16.82090372984188065, 29.19711159930560740, 10.99999999999877609 ) ) ;
#22339=CARTESIAN_POINT ( 'NONE',  ( -2.823200210931145815, 35.29864485453418865, 18.87996532025786323 ) ) ;
#22351=CARTESIAN_POINT ( 'NONE',  ( -0.5415361484146622439, 27.50000000000005329, 21.00000000000000355 ) ) ;
#22356=CARTESIAN_POINT ( 'NONE',  ( -34.68832217153530451, -7.625465254389222736, 16.87380292611359778 ) ) ;
#22364=( BOUNDED_CURVE ( )  B_SPLINE_CURVE ( 2, ( #12531, #22070, #15582 ),
 .UNSPECIFIED., .F., .F. ) 
 B_SPLINE_CURVE_WITH_KNOTS ( ( 3, 3 ),
 ( 0.000000000000000000, 1.000000000000000000 ),
 .UNSPECIFIED. ) 
 CURVE ( )  GEOMETRIC_REPRESENTATION_ITEM ( )  RATIONAL_B_SPLINE_CURVE ( ( 1.000000000000000000, 0.7071067811865475727, 1.000000000000000000 ) ) 
 REPRESENTATION_ITEM ( '' )  );
#22377=CARTESIAN_POINT ( 'NONE',  ( 22.38472516250418209, -15.35952186208521120, 20.99999999999999645 ) ) ;
#22378=CARTESIAN_POINT ( 'NONE',  ( 34.83511892542234278, -16.10726664690938392, 16.30093088680188984 ) ) ;
#22380=ORIENTED_EDGE ( 'NONE', *, *, #9518, .F. ) ;
#22381=CARTESIAN_POINT ( 'NONE',  ( -12.63297681466540467, 33.22352044042957431, 15.72805884748945005 ) ) ;
#22384=CARTESIAN_POINT ( 'NONE',  ( -5.400187688428998334E-14, 29.10878045366048639, 20.94377226548378346 ) ) ;
#22400=CARTESIAN_POINT ( 'NONE',  ( -28.38958307348538668, -9.126824876481562043, 20.50957957745985283 ) ) ;
#22427=CARTESIAN_POINT ( 'NONE',  ( 29.32420241873593625, -10.00128497722831611, 20.25080042701565830 ) ) ;
#22440=EDGE_LOOP ( 'NONE', ( #5852, #1965, #29037, #680 ) ) ;
#22442=CARTESIAN_POINT ( 'NONE',  ( 33.75875814100317029, 2.759858869446390361, 23.00000000000000000 ) ) ;
#22454=CARTESIAN_POINT ( 'NONE',  ( 32.84658669524289110, -23.46788009898384075, 10.99999999999997691 ) ) ;
#22466=CARTESIAN_POINT ( 'NONE',  ( -24.55877074691219164, -28.27742302307168742, 13.32518128616625930 ) ) ;
#22473=CARTESIAN_POINT ( 'NONE',  ( -13.80284393768010531, 29.83092525299177566, 16.87380292611440069 ) ) ;
#22476=CARTESIAN_POINT ( 'NONE',  ( -27.25314217027208841, 3.686469637083872541, 16.30093088680831315 ) ) ;
#22482=CARTESIAN_POINT ( 'NONE',  ( 24.65531199400567886, -28.60128534115905552, 11.55979286843931675 ) ) ;
#22502=CARTESIAN_POINT ( 'NONE',  ( 2.166144593658585915, 42.50000000000004974, 22.99999999999999289 ) ) ;
#22516=ORIENTED_EDGE ( 'NONE', *, *, #3158, .T. ) ;
#22533=CARTESIAN_POINT ( 'NONE',  ( -13.80290580123972966, 34.21636679304910444, 11.55979286843966314 ) ) ;
#22536=CARTESIAN_POINT ( 'NONE',  ( 2.498547013092441649, 33.82729453933308150, 19.66345542862528006 ) ) ;
#22559=CARTESIAN_POINT ( 'NONE',  ( -35.63595018118445523, -14.50160624002370469, 15.72805884748939143 ) ) ;
#22579=CARTESIAN_POINT ( 'NONE',  ( -39.31168172498703939, -14.28874104167793035, 11.00000000000000000 ) ) ;
#22585=CARTESIAN_POINT ( 'NONE',  ( 34.55475982899568521, -10.97206003969012755, 17.42190598798391932 ) ) ;
#22588=CARTESIAN_POINT ( 'NONE',  ( -6.751265526281039264, 37.11581529111845867, 16.30093088680186142 ) ) ;
#22590=CARTESIAN_POINT ( 'NONE',  ( 2.442402655125668787, 27.78651631404541789, 21.00000000000000355 ) ) ;
#22596=CARTESIAN_POINT ( 'NONE',  ( 16.78686424248630615, 15.93842542257170258, 18.42518152272128518 ) ) ;
#22606=CARTESIAN_POINT ( 'NONE',  ( -29.47277113412615179, -17.01611234805157480, 19.66345542862529072 ) ) ;
#22631=CARTESIAN_POINT ( 'NONE',  ( 29.36302367423321869, -15.61102309902083185, 19.99202127657103389 ) ) ;
#22665=CARTESIAN_POINT ( 'NONE',  ( -18.86506720475286514, -28.79250143785268534, 13.92931973827851522 ) ) ;
#22672=CARTESIAN_POINT ( 'NONE',  ( -33.75875814100324845, 2.759858869446484064, 3.000000000000000000 ) ) ;
#22675=CARTESIAN_POINT ( 'NONE',  ( 10.35750558343008798, 33.44896173338925394, 17.42190598798391932 ) ) ;
#22678=CARTESIAN_POINT ( 'NONE',  ( -17.92566989744610950, 16.47414500506816992, 17.42190598798358181 ) ) ;
#22680=CARTESIAN_POINT ( 'NONE',  ( 21.91981567634952910, -15.65087685632039793, 20.99999999999999645 ) ) ;
#22683=CARTESIAN_POINT ( 'NONE',  ( 33.53883321253825756, -0.1552552779180596254, 12.73282698324945805 ) ) ;
#22716=DIRECTION ( 'NONE',  ( 1.000000000000000000, 0.000000000000000000, 0.000000000000000000 ) ) ;
#22735=CARTESIAN_POINT ( 'NONE',  ( 9.340438144417221977, 38.00965938232028662, 11.00000000000005151 ) ) ;
#22740=CARTESIAN_POINT ( 'NONE',  ( 6.372562348371962671, 33.08234073371033190, 19.27171037444156809 ) ) ;
#22746=CARTESIAN_POINT ( 'NONE',  ( -28.79337657216479940, 4.963436916928028353, 11.00000000000544276 ) ) ;
#22750=CARTESIAN_POINT ( 'NONE',  ( -18.23649648353780961, -16.09146789626143814, 20.99999999999999645 ) ) ;
#22759=CARTESIAN_POINT ( 'NONE',  ( -32.49165476041793710, -0.9821698610459400625, 15.72805884748929373 ) ) ;
#22763=CARTESIAN_POINT ( 'NONE',  ( 33.75875814100317029, 2.759858869446390361, 11.00000000000000000 ) ) ;
#22777=EDGE_LOOP ( 'NONE', ( #2820, #30750, #39759, #10155 ) ) ;
#22783=CARTESIAN_POINT ( 'NONE',  ( 23.94800771174125842, -26.22823558801567145, 16.87380292611481636 ) ) ;
#22785=CARTESIAN_POINT ( 'NONE',  ( -1.824109939552144288, 39.35700678546971432, 15.13084544680213561 ) ) ;
#22786=B_SPLINE_CURVE_WITH_KNOTS ( 'NONE', 3,
 ( #38360, #26576, #13775, #1796, #20085, #31862, #10531, #26167, #22914, #38966, #35115, #10945, #35315, #35922, #7474, #38763, #28816, #38561 ),
 .UNSPECIFIED., .F., .F.,
 ( 4, 2, 2, 2, 2, 2, 2, 2, 4 ),
 ( 0.000000000000000000, 0.1249999999999998335, 0.2499999999999996669, 0.3749999999999995004, 0.4999999999999993339, 0.6249999999999994449, 0.7499999999999996669, 0.8749999999999997780, 1.000000000000000000 ),
 .UNSPECIFIED. ) ;
#22791=CARTESIAN_POINT ( 'NONE',  ( -4.143025606350054302E-14, 27.50000000000004974, 20.99999999999998934 ) ) ;
#22797=CARTESIAN_POINT ( 'NONE',  ( 15.85745926881093304, 21.40218184472425023, 17.42190598797886025 ) ) ;
#22807=CARTESIAN_POINT ( 'NONE',  ( -30.79094061804842397, -13.52614530981761831, 19.66345542862528006 ) ) ;
#22833=CARTESIAN_POINT ( 'NONE',  ( 19.13253804983751394, -21.21924640916230942, 20.25080042701564764 ) ) ;
#22855=CARTESIAN_POINT ( 'NONE',  ( -24.08646667827941101, -13.28101593840491290, 20.99999999999999645 ) ) ;
#22866=CARTESIAN_POINT ( 'NONE',  ( -37.13148535761799707, -14.80270701502672459, 11.55979286843934872 ) ) ;
#22873=CARTESIAN_POINT ( 'NONE',  ( -2.166144608099595636, 42.50000000000004974, 11.00000000000000000 ) ) ;
#22875=CARTESIAN_POINT ( 'NONE',  ( -8.686999124430418107, 33.93090424204633848, 17.92354375535250810 ) ) ;
#22878=CARTESIAN_POINT ( 'NONE',  ( -14.75813536907479318, 8.520613428071742490, 20.69868183039781329 ) ) ;
#22884=CARTESIAN_POINT ( 'NONE',  ( 35.07402885326985853, -20.24999999999990408, 11.55979286843934872 ) ) ;
#22892=VERTEX_POINT ( 'NONE', #33455 ) ;
#22914=CARTESIAN_POINT ( 'NONE',  ( -24.08861866610206093, -13.27715813466841865, 23.00000000000000355 ) ) ;
#22942=CARTESIAN_POINT ( 'NONE',  ( 13.80292604922460953, 34.21633694312859575, 11.00000000000012257 ) ) ;
#22946=CARTESIAN_POINT ( 'NONE',  ( 12.19685572513878036, 28.97783243917147900, 18.42518152272108622 ) ) ;
#22965=CARTESIAN_POINT ( 'NONE',  ( -27.04902410903751786, -24.92680750149321867, 16.87380292611406318 ) ) ;
#22988=CARTESIAN_POINT ( 'NONE',  ( 35.26975574857903695, -18.21959598282672488, 14.53008259254013979 ) ) ;
#22990=CARTESIAN_POINT ( 'NONE',  ( 5.259215691052598451, 38.11244126491433803, 15.72805884748939853 ) ) ;
#22991=CARTESIAN_POINT ( 'NONE',  ( 4.269522338418829820E-14, -20.30912387778604966, 19.66345542862528717 ) ) ;
#22994=CARTESIAN_POINT ( 'NONE',  ( 4.568463557893653437, 27.32878864566524868, 20.94377226548378346 ) ) ;
#23001=CARTESIAN_POINT ( 'NONE',  ( 31.24272016125543416, 0.2902395683448312225, 15.72805884748939498 ) ) ;
#23006=ORIENTED_EDGE ( 'NONE', *, *, #11114, .T. ) ;
#23011=CARTESIAN_POINT ( 'NONE',  ( -16.80389827882202880, -21.64427909825945662, 19.99202127657103389 ) ) ;
#23037=CARTESIAN_POINT ( 'NONE',  ( 30.23838254412189386, -12.22961151633820442, 19.99202127657102324 ) ) ;
#23062=CARTESIAN_POINT ( 'NONE',  ( -25.30804003627941867, -11.14301119665289264, 21.00000000000009948 ) ) ;
#23074=CARTESIAN_POINT ( 'NONE',  ( -16.88398162953599169, -29.10422986782303667, 12.14047268033038129 ) ) ;
#23088=CARTESIAN_POINT ( 'NONE',  ( -13.32472804387900567, 14.30980730577158155, 20.25080042701567251 ) ) ;
#23090=DIRECTION ( 'NONE',  ( -0.000000000000000000, -0.000000000000000000, -1.000000000000000000 ) ) ;
#23093=CARTESIAN_POINT ( 'NONE',  ( 37.09709568333405372, -7.051483854461498169, 11.55979286843942511 ) ) ;
#23107=CARTESIAN_POINT ( 'NONE',  ( 19.26948696230199687, 27.85601271560034675, 11.00000000000000000 ) ) ;
#23145=CARTESIAN_POINT ( 'NONE',  ( 1.947644445291152104, 40.50000000000006395, 11.55979286843935050 ) ) ;
#23149=CARTESIAN_POINT ( 'NONE',  ( 12.83067079990607340, 27.60880874002252128, 18.42518152272263521 ) ) ;
#23153=DIRECTION ( 'NONE',  ( -0.000000000000000000, -0.000000000000000000, -1.000000000000000000 ) ) ;
#23161=CARTESIAN_POINT ( 'NONE',  ( -4.817371740575545402, 23.83900317890010001, 20.99999999999999645 ) ) ;
#23169=CARTESIAN_POINT ( 'NONE',  ( -27.27686897039919955, -25.33890797347529755, 16.30093088680157010 ) ) ;
#23196=CARTESIAN_POINT ( 'NONE',  ( 32.79363849989022839, -0.7437118703939968878, 15.13084544680386578 ) ) ;
#23198=CARTESIAN_POINT ( 'NONE',  ( -8.305703523986128545, 36.29191545080267645, 16.30093088680110469 ) ) ;
#23200=CARTESIAN_POINT ( 'NONE',  ( -5.409649191045132532, -22.50706359516090060, 18.42518152272108978 ) ) ;
#23202=CARTESIAN_POINT ( 'NONE',  ( 5.000428297552684143, 29.07988060316543155, 20.69868183039781329 ) ) ;
#23211=CARTESIAN_POINT ( 'NONE',  ( 22.19651343351639738, 6.568638172588949331, 18.42518152272089793 ) ) ;
#23223=CARTESIAN_POINT ( 'NONE',  ( -30.78606151650984657, -16.23943018785164938, 19.27171037444191981 ) ) ;
#23239=CARTESIAN_POINT ( 'NONE',  ( 14.48927117870122494, -30.61587158504688588, 22.99999999999999289 ) ) ;
#23248=CARTESIAN_POINT ( 'NONE',  ( 28.25018339770975118, -2.647087534805041553, 19.27171037444157164 ) ) ;
#23271=CARTESIAN_POINT ( 'NONE',  ( -24.81299795227001326, -13.60183200321525732, 21.00000000000004619 ) ) ;
#23282=CARTESIAN_POINT ( 'NONE',  ( -24.63751168576463968, -28.54157386114988881, 12.14047268033103322 ) ) ;
#23291=CARTESIAN_POINT ( 'NONE',  ( 2.166144608099552116, 42.50000000000005684, 11.00000000000000178 ) ) ;
#23297=CARTESIAN_POINT ( 'NONE',  ( -11.93114467671392553, 6.888449590841186243, 20.99999999999999645 ) ) ;
#23299=CARTESIAN_POINT ( 'NONE',  ( 25.20894334605389986, -14.55439022683022543, 20.94377226548378346 ) ) ;
#23303=CARTESIAN_POINT ( 'NONE',  ( 36.68766582957253064, -16.69324967293806239, 12.14047268033083249 ) ) ;
#23306=FACE_OUTER_BOUND ( 'NONE', #12351, .T. ) ;
#23344=CARTESIAN_POINT ( 'NONE',  ( -19.48557158514998022, -11.24999999999982414, 23.00000000000000000 ) ) ;
#23358=CARTESIAN_POINT ( 'NONE',  ( 6.055828121132759811, 35.60995051739030259, 17.92354375535250099 ) ) ;
#23364=CARTESIAN_POINT ( 'NONE',  ( -17.34253826607186966, 27.32041144404028188, 11.00000000000000000 ) ) ;
#23377=CARTESIAN_POINT ( 'NONE',  ( -31.36686156446269536, -22.11446460981446549, 16.30093088680186852 ) ) ;
#23392=CARTESIAN_POINT ( 'NONE',  ( -29.42868960315909632, -26.31588593299390411, 11.00000000000013856 ) ) ;
#23396=VERTEX_POINT ( 'NONE', #18105 ) ;
#23398=CARTESIAN_POINT ( 'NONE',  ( 27.69088631811219159, -26.08775134479562396, 15.13084544680181054 ) ) ;
#23400=CARTESIAN_POINT ( 'NONE',  ( 5.476246462222536415, 38.75671607062970025, 14.53008259254011136 ) ) ;
#23402=CARTESIAN_POINT ( 'NONE',  ( 5.356921161177231383, -23.13411080437162326, 17.92354375535250810 ) ) ;
#23404=CARTESIAN_POINT ( 'NONE',  ( -7.722840163547155967, 25.57530741997960888, 20.69868183039764276 ) ) ;
#23406=ORIENTED_EDGE ( 'NONE', *, *, #25998, .F. ) ;
#23413=CARTESIAN_POINT ( 'NONE',  ( 12.60925743022028378, 20.19802119776807103, 19.66345542862461215 ) ) ;
#23423=CARTESIAN_POINT ( 'NONE',  ( -31.08318648610590884, -11.03630075675877364, 19.66345542862590889 ) ) ;
#23426=ORIENTED_EDGE ( 'NONE', *, *, #27135, .T. ) ;
#23448=CARTESIAN_POINT ( 'NONE',  ( 25.46386631785966159, -22.05997124774561513, 19.27171037444122348 ) ) ;
#23480=CARTESIAN_POINT ( 'NONE',  ( -34.04990527597851013, -21.89993885138022378, 12.14047268033099591 ) ) ;
#23493=CARTESIAN_POINT ( 'NONE',  ( -15.00309677617818771, 1.567672476163658013, 20.99999999999999645 ) ) ;
#23494=CARTESIAN_POINT ( 'NONE',  ( 24.70330546561584129, -7.131334670375485629, 20.94377226548427018 ) ) ;
#23498=CARTESIAN_POINT ( 'NONE',  ( 37.34232268491259532, -8.983628415038339199, 11.00000000000000000 ) ) ;
#23508=CARTESIAN_POINT ( 'NONE',  ( 5.578133564216165574, 24.05045924978295702, 20.99999999999999645 ) ) ;
#23512=CARTESIAN_POINT ( 'NONE',  ( 3.863783140547853712E-14, -86.77689918168233874, 23.00000000000000000 ) ) ;
#23513=CARTESIAN_POINT ( 'NONE',  ( -19.26948696230207858, 27.85601271560029701, 11.00000000000000000 ) ) ;
#23517=EDGE_CURVE ( 'NONE', #10557, #17915, #26478, .T. ) ;
#23540=CARTESIAN_POINT ( 'NONE',  ( 23.05386822411318803, -7.747535282638377652, 20.99999999999999645 ) ) ;
#23557=CARTESIAN_POINT ( 'NONE',  ( -9.490716042090618032, 32.53254263376179267, 18.42518152272187137 ) ) ;
#23564=CARTESIAN_POINT ( 'NONE',  ( 0.5459530983554482519, 27.49993477425252664, 23.00000000000000355 ) ) ;
#23577=CARTESIAN_POINT ( 'NONE',  ( -27.98024382195074367, -26.61114576561620026, 13.92931973827786685 ) ) ;
#23600=CARTESIAN_POINT ( 'NONE',  ( 35.60445263620119505, -7.407141432647699197, 15.72805884748942518 ) ) ;
#23602=CARTESIAN_POINT ( 'NONE',  ( -7.235364705666516905, 38.16413851588594497, 14.53008259254001544 ) ) ;
#23603=CARTESIAN_POINT ( 'NONE',  ( -11.06125417660426535, -21.75993793948570953, 19.27171037444298207 ) ) ;
#23605=CARTESIAN_POINT ( 'NONE',  ( -3.486159013132843043, 30.04627872069379535, 20.69868183039781684 ) ) ;
#23610=CARTESIAN_POINT ( 'NONE',  ( -5.578133564216452456, 24.05045924978193739, 20.99999999999999289 ) ) ;
#23615=CARTESIAN_POINT ( 'NONE',  ( 18.74997338759060383, -3.362744936764435089, 21.00000000000000000 ) ) ;
#23624=CARTESIAN_POINT ( 'NONE',  ( -25.46386631785724219, -22.05997124774662055, 19.27171037444124124 ) ) ;
#23648=CARTESIAN_POINT ( 'NONE',  ( 16.23042486173695309, -23.86708630543283149, 18.87996532025784546 ) ) ;
#23655=CARTESIAN_POINT ( 'NONE',  ( -33.14621996124576953, 0.5287779871183843072, 10.99999999999978506 ) ) ;
#23671=CARTESIAN_POINT ( 'NONE',  ( 16.87498849720590144, -29.16588574430808123, 10.99999999999838174 ) ) ;
#23680=CARTESIAN_POINT ( 'NONE',  ( -26.45121176803932173, -27.84758587393086060, 11.00000000000000000 ) ) ;
#23696=CARTESIAN_POINT ( 'NONE',  ( -11.07177992392671939, 13.25002113301073159, 20.82122704794080903 ) ) ;
#23697=CARTESIAN_POINT ( 'NONE',  ( 18.40750778688494904, -18.65192611823397328, 20.82122704794068113 ) ) ;
#23710=CARTESIAN_POINT ( 'NONE',  ( 17.28285333400959445, 27.30382183500221771, 12.14047268033097282 ) ) ;
#23756=FILL_AREA_STYLE_COLOUR ( '', #35929 ) ;
#23772=CARTESIAN_POINT ( 'NONE',  ( -22.52485696384032110, -27.93079472553808529, 15.13084544680170218 ) ) ;
#23788=CARTESIAN_POINT ( 'NONE',  ( -37.32914646357117050, -13.98551220633469150, 10.99999999999993783 ) ) ;
#23795=CARTESIAN_POINT ( 'NONE',  ( 27.50471383176380868, -25.75100844545640300, 15.72805884748903971 ) ) ;
#23797=CARTESIAN_POINT ( 'NONE',  ( 7.235364705665938700, 38.16413851588617234, 14.53008259254001011 ) ) ;
#23798=CARTESIAN_POINT ( 'NONE',  ( -16.05557028315303469, -24.54483004364683296, 18.42518152272108978 ) ) ;
#23800=CARTESIAN_POINT ( 'NONE',  ( 3.858525888476776800, 28.90799431746422243, 20.82122704794079837 ) ) ;
#23807=ADVANCED_FACE ( 'NONE', ( #5647 ), #32697, .T. ) ;
#23811=CARTESIAN_POINT ( 'NONE',  ( 23.79662817859708568, 0.8209266585812692307, 19.66345542863611939 ) ) ;
#23820=CARTESIAN_POINT ( 'NONE',  ( -32.25947621352474215, -13.82181017473423346, 18.87996532025784191 ) ) ;
#23836=CARTESIAN_POINT ( 'NONE',  ( -14.48927117870122316, -30.61587158504648087, 23.00000000000000000 ) ) ;
#23841=CARTESIAN_POINT ( 'NONE',  ( -39.51968005975108866, -13.07391886567259220, 11.00000000000000000 ) ) ;
#23847=CARTESIAN_POINT ( 'NONE',  ( 31.98112326865622279, -15.20435932463063899, 18.87996532025785967 ) ) ;
#23848=ORIENTED_EDGE ( 'NONE', *, *, #21338, .F. ) ;
#23852=CARTESIAN_POINT ( 'NONE',  ( -15.74227866054087066, -25.75916161678338057, 17.42190598798392998 ) ) ;
#23868=CARTESIAN_POINT ( 'NONE',  ( -14.98890121934409869, -28.67928442654153542, 11.55979286843934872 ) ) ;
#23871=CARTESIAN_POINT ( 'NONE',  ( -22.04303751225598873, -17.34387783897684443, 20.94377226548378346 ) ) ;
#23880=CARTESIAN_POINT ( 'NONE',  ( -27.36225479889090906, 10.16098284204026569, 11.00000000000000178 ) ) ;
#23883=CARTESIAN_POINT ( 'NONE',  ( -23.19735768193462278, -14.64350930037788423, 21.00000000000000355 ) ) ;
#23896=CARTESIAN_POINT ( 'NONE',  ( 25.56674216509423658, -13.93466449336444413, 20.94377226548378346 ) ) ;
#23914=CARTESIAN_POINT ( 'NONE',  ( -18.23649648353769948, -16.09146789626166196, 23.00000000000000000 ) ) ;
#23939=CARTESIAN_POINT ( 'NONE',  ( -25.43795106045734045, 8.821996438890993275, 13.32518128616756314 ) ) ;
#23953=EDGE_LOOP ( 'NONE', ( #32454, #25450, #14048, #14042 ) ) ;
#23995=CARTESIAN_POINT ( 'NONE',  ( 37.24966284334288247, -10.92205745603815714, 13.32518128616603015 ) ) ;
#23997=CARTESIAN_POINT ( 'NONE',  ( -15.50250408130212421, 30.73387816234496484, 13.92931973827792191 ) ) ;
#24000=CARTESIAN_POINT ( 'NONE',  ( 4.288075229727362547, 29.62123851724225077, 20.69868183039781329 ) ) ;
#24004=CARTESIAN_POINT ( 'NONE',  ( -16.81416712651214951, 27.17354907310119572, 13.92931973827808712 ) ) ;
#24011=CARTESIAN_POINT ( 'NONE',  ( 27.71565130972690127, -3.171757977843685961, 19.66345542862528362 ) ) ;
#24022=CARTESIAN_POINT ( 'NONE',  ( -28.56250045050152409, -21.55178514600735440, 18.42518152272108978 ) ) ;
#24049=CARTESIAN_POINT ( 'NONE',  ( 28.17486335742866643, -23.56478353225200095, 17.42190598798355339 ) ) ;
#24069=CARTESIAN_POINT ( 'NONE',  ( -10.09822582592840590, -27.41751403068705528, 11.00000000001392308 ) ) ;
#24072=CARTESIAN_POINT ( 'NONE',  ( -25.95165700074868553, -9.707988825434739510, 20.94377226548358806 ) ) ;
#24097=CARTESIAN_POINT ( 'NONE',  ( 26.10558707266147493, -11.85287147006363462, 20.94377226548379056 ) ) ;
#24100=CARTESIAN_POINT ( 'NONE',  ( 35.07402885326985142, -20.24999999999992184, 11.00000000000000000 ) ) ;
#24126=CARTESIAN_POINT ( 'NONE',  ( 16.58673509445612382, -31.15700704434060242, 11.00000000000000000 ) ) ;
#24135=CARTESIAN_POINT ( 'NONE',  ( -23.01716326618291575, 13.28896540771138213, 12.73282698324853079 ) ) ;
#24176=VERTEX_POINT ( 'NONE', #37732 ) ;
#24192=CARTESIAN_POINT ( 'NONE',  ( 36.42486030274157116, -16.61012894281671137, 13.32518128616598574 ) ) ;
#24194=CARTESIAN_POINT ( 'NONE',  ( 13.15436037709940287, 33.66595454666934728, 14.53008259254018242 ) ) ;
#24195=CARTESIAN_POINT ( 'NONE',  ( -5.799013854623373376, -17.87737810982027398, 20.50957957746029336 ) ) ;
#24197=CARTESIAN_POINT ( 'NONE',  ( -9.555312204553054301, 25.15592819202761632, 20.25080042701566541 ) ) ;
#24205=AXIS2_PLACEMENT_3D ( 'NONE', #34742, #9762, #3460 ) ;
#24207=CARTESIAN_POINT ( 'NONE',  ( 10.32009510687484521, 12.89643020664140316, 20.94377226548379411 ) ) ;
#24219=CARTESIAN_POINT ( 'NONE',  ( -18.99709059511109288, -25.05170461721374053, 18.42518152272145571 ) ) ;
#24238=AXIS2_PLACEMENT_3D ( 'NONE', #4469, #10767, #25593 ) ;
#24239=CARTESIAN_POINT ( 'NONE',  ( -18.77248997590657709, -31.35432035705730414, 11.00000000000000000 ) ) ;
#24246=CARTESIAN_POINT ( 'NONE',  ( 31.37624276535957435, -18.11508220673916014, 18.42518152272108622 ) ) ;
#24253=CARTESIAN_POINT ( 'NONE',  ( -37.48524466415686618, -10.08537157645187499, 11.00000000000012967 ) ) ;
#24263=ADVANCED_FACE ( 'NONE', ( #28581 ), #10500, .F. ) ;
#24267=CARTESIAN_POINT ( 'NONE',  ( 4.250808094710701366E-14, -26.77689918168226058, 11.55979286843934872 ) ) ;
#24271=CARTESIAN_POINT ( 'NONE',  ( -23.10579450714032745, -17.79557859931359332, 20.82122704794065982 ) ) ;
#24298=CARTESIAN_POINT ( 'NONE',  ( 25.98021325959767225, -4.875178728622389102, 20.50957957746029336 ) ) ;
#24302=ADVANCED_FACE ( 'NONE', ( #17008 ), #34664, .F. ) ;
#24338=ORIENTED_EDGE ( 'NONE', *, *, #12294, .T. ) ;
#24340=CARTESIAN_POINT ( 'NONE',  ( -20.35904855840124128, 17.61891361913183474, 13.32518128616461084 ) ) ;
#24360=CARTESIAN_POINT ( 'NONE',  ( 3.831426523743819423, 25.75866349410729939, 22.99999999999999289 ) ) ;
#24376=EDGE_LOOP ( 'NONE', ( #33441, #17466, #10552, #33856 ) ) ;
#24394=ORIENTED_EDGE ( 'NONE', *, *, #13824, .T. ) ;
#24395=CARTESIAN_POINT ( 'NONE',  ( 9.237168799396084040, 37.83823547837376111, 12.73282698324857520 ) ) ;
#24397=CARTESIAN_POINT ( 'NONE',  ( -17.62780868050356986, -18.45076755199228202, 20.82122704794079837 ) ) ;
#24399=CARTESIAN_POINT ( 'NONE',  ( -3.838817179443412275, 30.80979998870936498, 20.50957957746028981 ) ) ;
#24418=CARTESIAN_POINT ( 'NONE',  ( -30.63324413334818885, -19.40199358733788415, 18.42518152272070964 ) ) ;
#24424=ORIENTED_EDGE ( 'NONE', *, *, #31159, .F. ) ;
#24442=CARTESIAN_POINT ( 'NONE',  ( 28.97703757779505551, -22.02226062111144955, 17.92354375535251165 ) ) ;
#24462=CARTESIAN_POINT ( 'NONE',  ( 15.12590024503359842, -28.14827041158748244, 13.92931973827808534 ) ) ;
#24465=CARTESIAN_POINT ( 'NONE',  ( -22.70288158165621084, -17.06695585772259705, 20.94377226548368753 ) ) ;
#24468=EDGE_LOOP ( 'NONE', ( #5847, #37268, #24424, #31924 ) ) ;
#24471=AXIS2_PLACEMENT_3D ( 'NONE', #23344, #18057, #26990 ) ;
#24484=CARTESIAN_POINT ( 'NONE',  ( 18.72723793738837372, -3.339582153676996512, 23.00000000000000000 ) ) ;
#24490=CARTESIAN_POINT ( 'NONE',  ( 25.35679574134477932, -6.615406304682780458, 20.82122704794150181 ) ) ;
#24524=CARTESIAN_POINT ( 'NONE',  ( 14.48927117870123027, -30.61587158504688233, 11.00000000000000000 ) ) ;
#24525=CARTESIAN_POINT ( 'NONE',  ( -26.12394372346507865, -27.06777822797208088, 14.53008259254010959 ) ) ;
#24540=CARTESIAN_POINT ( 'NONE',  ( -28.79337657216479585, 4.963436916928034570, 11.00000000000544276 ) ) ;
#24569=CARTESIAN_POINT ( 'NONE',  ( 4.817371740575539185, 23.83900317890011067, 23.00000000000000000 ) ) ;
#24598=CARTESIAN_POINT ( 'NONE',  ( -7.450289500751556382, 38.62958991718460311, 13.32518128616595376 ) ) ;
#24600=CARTESIAN_POINT ( 'NONE',  ( 4.311100837790133051E-14, -15.38567963534269900, 20.94377226548378701 ) ) ;
#24602=CARTESIAN_POINT ( 'NONE',  ( -3.426866961292544644, 32.67295397237167975, 19.99202127657103034 ) ) ;
#24619=CARTESIAN_POINT ( 'NONE',  ( -30.57450045107738035, -0.3656520783173805578, 16.87380292611442201 ) ) ;
#24630=CARTESIAN_POINT ( 'NONE',  ( 38.42882785865584339, -4.479089857566261657, 11.00000000000000000 ) ) ;
#24641=CARTESIAN_POINT ( 'NONE',  ( 29.39157470508798298, -22.49273609621582182, 17.42190598798393353 ) ) ;
#24653=CARTESIAN_POINT ( 'NONE',  ( 28.53381226737487708, 4.748233269553930214, 13.32518128616595909 ) ) ;
#24663=CARTESIAN_POINT ( 'NONE',  ( -27.76392016787528760, -12.00403709334065461, 20.69868183039782039 ) ) ;
#24690=CARTESIAN_POINT ( 'NONE',  ( 23.50870743262586160, -18.52420134090368720, 20.69868183039761789 ) ) ;
#24699=CARTESIAN_POINT ( 'NONE',  ( -27.36225479881674616, 10.16098284219160597, 22.99999999999999645 ) ) ;
#24707=FILL_AREA_STYLE_COLOUR ( '', #11940 ) ;
#24713=CARTESIAN_POINT ( 'NONE',  ( 4.881458130820872654, -28.77689918168226768, 11.00000000000000178 ) ) ;
#24717=CARTESIAN_POINT ( 'NONE',  ( 30.17922767059877032, -0.7536324250949817394, 17.42190598798393353 ) ) ;
#24722=CARTESIAN_POINT ( 'NONE',  ( -15.20016916874712365, -27.86040092368495280, 14.53008259254011136 ) ) ;
#24732=CARTESIAN_POINT ( 'NONE',  ( -25.55085611915244570, 8.900480655597387880, 12.73282698325014550 ) ) ;
#24782=DIRECTION ( 'NONE',  ( -0.000000000000000000, -0.000000000000000000, -1.000000000000000000 ) ) ;
#24793=CARTESIAN_POINT ( 'NONE',  ( -1.926143243141299921, 40.30103163374180752, 12.73282698324853079 ) ) ;
#24794=CARTESIAN_POINT ( 'NONE',  ( 4.290760370981760375E-14, -17.87737810982027398, 20.50957957746029336 ) ) ;
#24796=CARTESIAN_POINT ( 'NONE',  ( 1.073573824165682256, 32.41755745572909575, 20.25080042701565830 ) ) ;
#24813=VERTEX_POINT ( 'NONE', #25291 ) ;
#24816=CARTESIAN_POINT ( 'NONE',  ( -28.17486335743007686, -23.56478353225083922, 17.42190598798394774 ) ) ;
#24840=CARTESIAN_POINT ( 'NONE',  ( 20.56996978659388731, -26.19496882840791940, 17.42190598798392642 ) ) ;
#24852=CARTESIAN_POINT ( 'NONE',  ( 17.15083734909311630, 27.26712758906529643, 12.73282698324853257 ) ) ;
#24862=CARTESIAN_POINT ( 'NONE',  ( -26.56332897235036228, -4.302820985780034135, 20.25080042701566541 ) ) ;
#24865=FACE_OUTER_BOUND ( 'NONE', #24376, .T. ) ;
#24869=VERTEX_POINT ( 'NONE', #3951 ) ;
#24890=CARTESIAN_POINT ( 'NONE',  ( 27.68412949013584168, -10.20944236609925859, 20.69868183039781329 ) ) ;
#24900=CARTESIAN_POINT ( 'NONE',  ( -4.817371740575532080, 23.83900317890012843, 23.00000000000000000 ) ) ;
#24926=CARTESIAN_POINT ( 'NONE',  ( -27.83556507003000391, -26.34944855520640061, 14.53008259253985379 ) ) ;
#24936=CARTESIAN_POINT ( 'NONE',  ( -11.11100267139899778, 25.58833710556205077, 19.66345542862528717 ) ) ;
#24942=CARTESIAN_POINT ( 'NONE',  ( 28.15028875895061944, -26.91874057850925439, 12.73282698324841888 ) ) ;
#24963=CARTESIAN_POINT ( 'NONE',  ( 15.33540832684242616, 35.51988609203954894, 23.00000000000000711 ) ) ;
#24995=CARTESIAN_POINT ( 'NONE',  ( -7.508063977623400831, 38.75471409550113577, 12.73282698324837980 ) ) ;
#24999=CARTESIAN_POINT ( 'NONE',  ( -8.768078002823385120, 24.93711404285670596, 20.50957957746029692 ) ) ;
#25015=CARTESIAN_POINT ( 'NONE',  ( -31.14237565978616118, -19.77424633423363787, 17.92354375535212796 ) ) ;
#25032=DIRECTION ( 'NONE',  ( 1.000000000000000000, 0.000000000000000000, 0.000000000000000000 ) ) ;
#25038=CARTESIAN_POINT ( 'NONE',  ( 34.68832217153572373, -7.625465254387286507, 16.87380292611443267 ) ) ;
#25043=LINE ( 'NONE', #16300, #31214 ) ;
#25045=CARTESIAN_POINT ( 'NONE',  ( 3.833852081710590110, 25.75497152300995296, 21.00000000000000355 ) ) ;
#25062=CARTESIAN_POINT ( 'NONE',  ( -26.64268929643286299, -15.38216383723055714, 20.69868183039780973 ) ) ;
#25088=CARTESIAN_POINT ( 'NONE',  ( 27.09004689510926056, -14.60731774717147680, 20.69868183039781329 ) ) ;
#25113=CARTESIAN_POINT ( 'NONE',  ( -75.15099915297791711, 43.38844959084113384, 3.000000000000000000 ) ) ;
#25121=CARTESIAN_POINT ( 'NONE',  ( -37.24966284334341537, -10.92205745603902045, 13.32518128616676911 ) ) ;
#25132=CARTESIAN_POINT ( 'NONE',  ( -21.05742987670793909, 12.15751280775709020, 16.87380292611441490 ) ) ;
#25135=CARTESIAN_POINT ( 'NONE',  ( 23.43672666297240426, -8.137589884419345054, 23.00000000000000355 ) ) ;
#25139=CARTESIAN_POINT ( 'NONE',  ( 36.21549415350893497, -5.268335738863441975, 13.32518128616590225 ) ) ;
#25162=CARTESIAN_POINT ( 'NONE',  ( -2.166144593658632544, 42.50000000000004974, 11.00000000000000000 ) ) ;
#25190=VERTEX_POINT ( 'NONE', #40081 ) ;
#25194=CARTESIAN_POINT ( 'NONE',  ( -15.69117760686815721, 30.83412033666087737, 13.32518128616588093 ) ) ;
#25199=CARTESIAN_POINT ( 'NONE',  ( 4.159699369156109938, 34.84843100105947400, 18.87996532025784902 ) ) ;
#25210=CARTESIAN_POINT ( 'NONE',  ( 0.5415361484146482551, 27.50000000000004974, 20.99999999999999289 ) ) ;
#25216=CARTESIAN_POINT ( 'NONE',  ( -33.56035593554165075, -14.08372035823108526, 17.92354375535250810 ) ) ;
#25219=ADVANCED_FACE ( 'NONE', ( #12256 ), #27302, .T. ) ;
#25238=CARTESIAN_POINT ( 'NONE',  ( 30.17922767059609512, -0.7536324250923613910, 17.42190598798392998 ) ) ;
#25242=CARTESIAN_POINT ( 'NONE',  ( 1.848241319495468993, 27.98666583367186078, 21.00000000000000355 ) ) ;
#25250=ADVANCED_FACE ( 'NONE', ( #12453 ), #31416, .F. ) ;
#25259=CARTESIAN_POINT ( 'NONE',  ( -19.19127776371468030, -19.55740820284875880, 20.69868183039799092 ) ) ;
#25287=CARTESIAN_POINT ( 'NONE',  ( 21.42135062927563993, -21.87239811599182460, 19.99202127657103745 ) ) ;
#25291=CARTESIAN_POINT ( 'NONE',  ( 14.98890121934609532, -28.67928442654220333, 2.999999999999999112 ) ) ;
#25295=B_SPLINE_CURVE_WITH_KNOTS ( 'NONE', 3,
 ( #14783, #36321, #24713, #18232, #33873, #12129 ),
 .UNSPECIFIED., .F., .F.,
 ( 4, 2, 4 ),
 ( 0.000000000000000000, 0.5000000000000000000, 1.000000000000000000 ),
 .UNSPECIFIED. ) ;
#25318=CARTESIAN_POINT ( 'NONE',  ( -36.55626306615705090, -16.65168930787910284, 12.73282698324876350 ) ) ;
#25326=CARTESIAN_POINT ( 'NONE',  ( 4.960307196185259393, 37.22510528292774268, 16.87380292611441845 ) ) ;
#25329=CARTESIAN_POINT ( 'NONE',  ( -21.86831431663999936, 12.62567715743360530, 15.72805884748939498 ) ) ;
#25331=CARTESIAN_POINT ( 'NONE',  ( 24.51396478725026640, -11.15767879383070138, 20.99999999999999645 ) ) ;
#25336=CARTESIAN_POINT ( 'NONE',  ( 18.85757713438717786, -29.00601609346521670, 13.32518128616639785 ) ) ;
#25385=CARTESIAN_POINT ( 'NONE',  ( -15.93459161340889096, 30.96344742789386828, 12.14047268033069393 ) ) ;
#25388=CARTESIAN_POINT ( 'NONE',  ( -1.072992850107295468E-13, 35.53022820328502718, 18.87996532025784546 ) ) ;
#25401=AXIS2_PLACEMENT_3D ( 'NONE', #15608, #19052, #28391 ) ;
#25403=CARTESIAN_POINT ( 'NONE',  ( 4.817371740575539185, 23.83900317890011422, 20.99999999999999645 ) ) ;
#25407=CARTESIAN_POINT ( 'NONE',  ( -18.95257105546425791, -26.31232633481670646, 17.42190598798432077 ) ) ;
#25429=CARTESIAN_POINT ( 'NONE',  ( 32.48135758214254309, -20.75321993593874126, 16.30093088680188984 ) ) ;
#25432=CARTESIAN_POINT ( 'NONE',  ( -4.002244506128481483, 26.73020382270282269, 21.00000000000009237 ) ) ;
#25439=CARTESIAN_POINT ( 'NONE',  ( 17.28285333400761914, 27.30382183500914550, 12.14047268033097460 ) ) ;
#25447=CARTESIAN_POINT ( 'NONE',  ( -18.04765032505036970, -21.12132759291239381, 20.25080042701569027 ) ) ;
#25450=ORIENTED_EDGE ( 'NONE', *, *, #12294, .F. ) ;
#25475=CARTESIAN_POINT ( 'NONE',  ( 26.84751477640508810, -17.98144108585584178, 20.25080042701592120 ) ) ;
#25494=( LENGTH_UNIT ( ) NAMED_UNIT ( * ) SI_UNIT ( .MILLI., .METRE. ) );
#25512=CARTESIAN_POINT ( 'NONE',  ( -24.59814121633841566, -28.40949844211078812, 12.73282698324864626 ) ) ;
#25519=CARTESIAN_POINT ( 'NONE',  ( 18.68939205906152523, 29.94303747981216901, 11.00000000000000000 ) ) ;
#25520=CARTESIAN_POINT ( 'NONE',  ( -4.960307196185540057, 37.22510528292767873, 16.87380292611441845 ) ) ;
#25525=CARTESIAN_POINT ( 'NONE',  ( -17.58821720676843370, 10.15456193889213665, 19.66345542862528362 ) ) ;
#25531=CARTESIAN_POINT ( 'NONE',  ( 34.04990527597812644, -21.89993885138089524, 12.14047268033092308 ) ) ;
#25545=CARTESIAN_POINT ( 'NONE',  ( 22.48079666807004529, 18.61591633964211212, 11.00000000000000178 ) ) ;
#25586=CARTESIAN_POINT ( 'NONE',  ( -7.591957726968742826, 38.93640765974102180, 11.55979286843917464 ) ) ;
#25589=CARTESIAN_POINT ( 'NONE',  ( 7.884092257452433472, 32.87438847863636937, 18.87996532025784902 ) ) ;
#25593=DIRECTION ( 'NONE',  ( 1.000000000000000000, 0.000000000000000000, 0.000000000000000000 ) ) ;
#25607=CARTESIAN_POINT ( 'NONE',  ( -35.45119270310583914, -5.541672998605994493, 15.13084544680260457 ) ) ;
#25630=CARTESIAN_POINT ( 'NONE',  ( 30.90861030616521177, -0.03770625498525858460, 16.30093088680191116 ) ) ;
#25632=CARTESIAN_POINT ( 'NONE',  ( 3.652674690108948852, 39.05729514278202430, 15.13084544680221732 ) ) ;
#25635=CARTESIAN_POINT ( 'NONE',  ( -5.067517038533118523, 26.80213145839204358, 20.94377226548377990 ) ) ;
#25644=CARTESIAN_POINT ( 'NONE',  ( 15.47112132963536446, 15.31948306976098628, 19.27171037444173507 ) ) ;
#25653=CARTESIAN_POINT ( 'NONE',  ( -17.42101839920251649, -19.25229542401853067, 20.69868183039781329 ) ) ;
#25681=CARTESIAN_POINT ( 'NONE',  ( 26.17288861939790579, -20.72787579792467838, 19.66345542862498519 ) ) ;
#25688=B_SPLINE_CURVE_WITH_KNOTS ( 'NONE', 3,
 ( #9947, #16444, #10550, #19284, #32080, #13182, #31679, #29236, #1007, #16652, #4452, #28631, #29034, #26183, #1210, #1408, #19483, #3847 ),
 .UNSPECIFIED., .F., .F.,
 ( 4, 2, 2, 2, 2, 2, 2, 2, 4 ),
 ( 0.000000000000000000, 0.1250000000000000555, 0.2500000000000001110, 0.3750000000000001665, 0.5000000000000002220, 0.6250000000000002220, 0.7500000000000003331, 0.8750000000000001110, 1.000000000000000000 ),
 .UNSPECIFIED. ) ;
#25717=CARTESIAN_POINT ( 'NONE',  ( -24.49773858737561838, -28.07267629079790439, 13.92931973827830383 ) ) ;
#25723=CARTESIAN_POINT ( 'NONE',  ( 10.37659643210531257, 39.73422260934388106, 11.00000000000000000 ) ) ;
#25725=CARTESIAN_POINT ( 'NONE',  ( 6.320269494896071372, 36.18253918181417816, 17.42190598798391221 ) ) ;
#25726=ORIENTED_EDGE ( 'NONE', *, *, #30406, .T. ) ;
#25729=CARTESIAN_POINT ( 'NONE',  ( -22.71318823113784546, 6.927825590549916868, 17.92354375535276390 ) ) ;
#25731=CARTESIAN_POINT ( 'NONE',  ( 22.79104142221947171, -15.00151558123164008, 20.99999999999999645 ) ) ;
#25734=CARTESIAN_POINT ( 'NONE',  ( 37.28086807198950225, -8.991428209509072289, 12.14047268033097815 ) ) ;
#25747=CARTESIAN_POINT ( 'NONE',  ( 20.57674455326933582, 23.15285302515658472, 10.99999999999999822 ) ) ;
#25756=CARTESIAN_POINT ( 'NONE',  ( 4.331888854854896387, 42.14502281367649772, 22.99999999999999645 ) ) ;
#25762=CIRCLE ( 'NONE', #8258, 18.00000000000002487 ) ;
#25768=CARTESIAN_POINT ( 'NONE',  ( -38.48801548572855324, -4.879739702264117795, 10.99999999999999822 ) ) ;
#25788=SHAPE_DEFINITION_REPRESENTATION ( #1274, #12760 ) ;
#25789=CARTESIAN_POINT ( 'NONE',  ( 15.98959510862154509, 30.99271259066425088, 11.55979286843923148 ) ) ;
#25793=CARTESIAN_POINT ( 'NONE',  ( -2.498547013092590863, 33.82729453933302466, 19.66345542862529427 ) ) ;
#25796=DIRECTION ( 'NONE',  ( -0.000000000000000000, -0.000000000000000000, -1.000000000000000000 ) ) ;
#25810=CARTESIAN_POINT ( 'NONE',  ( 15.07283634909883752, -28.35394831540530447, 13.32518128616608699 ) ) ;
#25814=CARTESIAN_POINT ( 'NONE',  ( -34.64549836162045438, -5.829828142712631056, 16.30093088680235880 ) ) ;
#25836=CARTESIAN_POINT ( 'NONE',  ( 25.67968615518546827, -26.00921032235772046, 16.30093088680190760 ) ) ;
#25838=CARTESIAN_POINT ( 'NONE',  ( 7.110004120643233172, 37.89265721834169653, 15.13084544680205390 ) ) ;
#25840=CARTESIAN_POINT ( 'NONE',  ( 5.578133564216165574, 24.05045924978294991, 20.99999999999999645 ) ) ;
#25846=CARTESIAN_POINT ( 'NONE',  ( 15.42165057837873654, 26.78649484832369154, 16.30093088680190760 ) ) ;
#25854=CARTESIAN_POINT ( 'NONE',  ( -21.42136340053371057, -21.87239718931726173, 19.99202127657076034 ) ) ;
#25881=CARTESIAN_POINT ( 'NONE',  ( 30.09689698601827246, -15.93509466225769344, 19.66345542862528362 ) ) ;
#25904=CARTESIAN_POINT ( 'NONE',  ( -23.43324262027536875, -8.134040356058614307, 20.99999999999999645 ) ) ;
#25910=AXIS2_PLACEMENT_3D ( 'NONE', #32097, #25796, #38193 ) ;
#25916=CARTESIAN_POINT ( 'NONE',  ( -29.80853493429716750, -25.87953118560963617, 12.73282698324867468 ) ) ;
#25922=LINE ( 'NONE', #1351, #27082 ) ;
#25924=CARTESIAN_POINT ( 'NONE',  ( -13.31085751088330760, 29.56957116847145173, 17.42190598798392998 ) ) ;
#25933=CARTESIAN_POINT ( 'NONE',  ( 37.31659891191883105, -12.87518290988953495, 12.73282698324865514 ) ) ;
#25936=ORIENTED_EDGE ( 'NONE', *, *, #9033, .F. ) ;
#25945=EDGE_CURVE ( 'NONE', #17014, #27076, #12753, .T. ) ;
#25987=CARTESIAN_POINT ( 'NONE',  ( 12.44178368932906409, 35.65276919561902957, 11.55979286843929543 ) ) ;
#25990=CARTESIAN_POINT ( 'NONE',  ( 13.83280510892147674, 26.34487040058358076, 17.92354375535250810 ) ) ;
#25998=EDGE_CURVE ( 'NONE', #6337, #22892, #15211, .T. ) ;
#26005=CARTESIAN_POINT ( 'NONE',  ( 3.456468065140018808, 26.15323006594238464, 20.99999999999998934 ) ) ;
#26010=CARTESIAN_POINT ( 'NONE',  ( -35.14638740386807569, -7.516303343519180835, 16.30093088680109048 ) ) ;
#26027=AXIS2_PLACEMENT_3D ( 'NONE', #35099, #38750, #4011 ) ;
#26035=CARTESIAN_POINT ( 'NONE',  ( 36.43809855126006880, -10.93713533239221825, 15.13084544680210364 ) ) ;
#26037=CARTESIAN_POINT ( 'NONE',  ( -1.474891194420403403E-13, 38.97445513318768207, 15.72805884748939498 ) ) ;
#26038=CARTESIAN_POINT ( 'NONE',  ( 4.276346332578968397E-14, -21.80712738496724157, 18.87996532025784902 ) ) ;
#26040=CARTESIAN_POINT ( 'NONE',  ( -1.082972213713723431, 27.41125570341915463, 20.99999999999999645 ) ) ;
#26047=CARTESIAN_POINT ( 'NONE',  ( 31.51573171626900205, 0.5582143012820769412, 15.13084544680213739 ) ) ;
#26056=CARTESIAN_POINT ( 'NONE',  ( -16.60464863832889648, -22.41657912773201744, 19.66345542862528362 ) ) ;
#26076=CARTESIAN_POINT ( 'NONE',  ( -35.27625572565145973, 1.213838575764629946, 23.00000000000000000 ) ) ;
#26080=CARTESIAN_POINT ( 'NONE',  ( 28.20105441993420925, -17.62361288429907447, 19.99202127657103389 ) ) ;
#26105=CARTESIAN_POINT ( 'NONE',  ( -19.30730118283918628, -16.27608008926400274, 20.99999999999999645 ) ) ;
#26118=CARTESIAN_POINT ( 'NONE',  ( -20.78821643698927701, -29.20280246618805720, 11.00000000000000000 ) ) ;
#26125=CARTESIAN_POINT ( 'NONE',  ( 8.437494178870114325, 40.76200630940460456, 11.00000000000000178 ) ) ;
#26127=CARTESIAN_POINT ( 'NONE',  ( 12.85888779259182968, 31.22252129899190720, 16.87380292611442201 ) ) ;
#26130=CARTESIAN_POINT ( 'NONE',  ( -10.32009510687426435, 12.89643020662261108, 20.94377226548379056 ) ) ;
#26138=CARTESIAN_POINT ( 'NONE',  ( 37.34232268491259532, -8.983628415038312554, 11.55979286843934872 ) ) ;
#26159=CLOSED_SHELL ( 'NONE', ( #35204, #35647, #1730, #6258, #12387, #7373, #28137, #23807, #4885, #21893, #20744, #27980, #4681, #11590, #37536, #8741, #27444, #24263, #25219, #14998, #11270, #4797, #31707, #25250, #38691, #33970, #21410, #24302, #34954 ) ) ;
#26167=CARTESIAN_POINT ( 'NONE',  ( -24.27952205336340441, -12.77208933892361209, 23.00000000000000711 ) ) ;
#26174=CARTESIAN_POINT ( 'NONE',  ( -24.08646667827941457, -13.28101593840491468, 21.00000000000000000 ) ) ;
#26183=CARTESIAN_POINT ( 'NONE',  ( -31.94006737154284892, 0.9747213384881107112, 13.92931973827808534 ) ) ;
#26192=CARTESIAN_POINT ( 'NONE',  ( 17.34253826607184834, 27.32041144404034938, 11.00000000000000178 ) ) ;
#26195=CARTESIAN_POINT ( 'NONE',  ( 2.974899668820615073, 35.98612526451933746, 18.42518152272109333 ) ) ;
#26198=ORIENTED_EDGE ( 'NONE', *, *, #17114, .F. ) ;
#26216=CARTESIAN_POINT ( 'NONE',  ( -33.89025995733841512, -4.271010277521935627, 16.30093088680190405 ) ) ;
#26240=CARTESIAN_POINT ( 'NONE',  ( 33.86049899301212207, -2.258468967557679452, 15.13084544680245536 ) ) ;
#26242=CARTESIAN_POINT ( 'NONE',  ( -6.948689594653023605, 37.54332414141784113, 15.72805884748933813 ) ) ;
#26243=CARTESIAN_POINT ( 'NONE',  ( 10.93513760492762366, -22.50092802241915635, 18.87996532025630003 ) ) ;
#26245=CARTESIAN_POINT ( 'NONE',  ( -6.839309919355111234, 27.13928353713039954, 20.69868183039781329 ) ) ;
#26254=CARTESIAN_POINT ( 'NONE',  ( 13.83280510891587767, 26.34487040060352925, 17.92354375535250810 ) ) ;
#26266=CARTESIAN_POINT ( 'NONE',  ( -17.00801676779734350, -20.85310720624813641, 20.25080042701566541 ) ) ;
#26275=CARTESIAN_POINT ( 'NONE',  ( -9.742785792574970571, -49.01344959084108410, 3.000000000000000000 ) ) ;
#26291=CARTESIAN_POINT ( 'NONE',  ( 16.41753675003191759, -23.14183271658236762, 19.27171037444156454 ) ) ;
#26294=AXIS2_PLACEMENT_3D ( 'NONE', #1335, #935, #13518 ) ;
#26311=CARTESIAN_POINT ( 'NONE',  ( 14.48927117870123027, -30.61587158504688233, 11.00000000000000000 ) ) ;
#26316=CARTESIAN_POINT ( 'NONE',  ( -25.28503033819723456, -11.77807541141262782, 20.99999999999999645 ) ) ;
#26326=CARTESIAN_POINT ( 'NONE',  ( -37.58754968649146377, -10.91577297561622117, 11.55979286843978215 ) ) ;
#26339=CARTESIAN_POINT ( 'NONE',  ( -12.61496056324094539, 7.283250877003592194, 20.99999999999999645 ) ) ;
#26341=CARTESIAN_POINT ( 'NONE',  ( 25.28503033819712087, -11.77807541141322822, 20.99999999999999645 ) ) ;
#26346=CARTESIAN_POINT ( 'NONE',  ( 36.47502800187007210, -5.175502249961421164, 12.14047268033090887 ) ) ;
#26396=CARTESIAN_POINT ( 'NONE',  ( -1.189115275033253716E-13, 36.23016441347868977, 18.42518152272108622 ) ) ;
#26418=CARTESIAN_POINT ( 'NONE',  ( -29.03912765165685528, -24.78940378269006573, 15.72805884748945715 ) ) ;
#26439=CARTESIAN_POINT ( 'NONE',  ( 36.73707435953490119, -10.93158220173851802, 14.53008259254007051 ) ) ;
#26441=CARTESIAN_POINT ( 'NONE',  ( 13.24632657851087991, 31.48533120267433461, 16.30093088680191116 ) ) ;
#26443=CARTESIAN_POINT ( 'NONE',  ( 11.18737074831306266, -21.01894785638886987, 19.66345542862420714 ) ) ;
#26446=CARTESIAN_POINT ( 'NONE',  ( -4.499574175057204251, 28.42082499241989169, 20.82122704794079837 ) ) ;
#26453=CARTESIAN_POINT ( 'NONE',  ( 18.85374159600720745, 16.91074157332428385, 16.30093088680196445 ) ) ;
#26456=CARTESIAN_POINT ( 'NONE',  ( -13.80290580123967992, 34.21636679304901918, 11.00000000000033218 ) ) ;
#26466=CARTESIAN_POINT ( 'NONE',  ( -30.40812954450618832, -7.345122744317324148, 19.66345542862560691 ) ) ;
#26478=CIRCLE ( 'NONE', #21294, 58.00000000000006395 ) ;
#26488=CARTESIAN_POINT ( 'NONE',  ( -24.51396478725048667, -11.15767879383074757, 23.00000000000000000 ) ) ;
#26494=CARTESIAN_POINT ( 'NONE',  ( 30.54456991890647899, -14.74984208377836481, 19.66345542862529072 ) ) ;
#26505=CARTESIAN_POINT ( 'NONE',  ( -23.05386822411323422, -7.747535282638357224, 23.00000000000000000 ) ) ;
#26522=CARTESIAN_POINT ( 'NONE',  ( -21.14791330573199346, -16.83114732581389461, 21.00000000000004619 ) ) ;
#26532=CARTESIAN_POINT ( 'NONE',  ( -34.83527399001570046, -1.648960735038180525, 11.55979286843900411 ) ) ;
#26545=( BOUNDED_CURVE ( )  B_SPLINE_CURVE ( 2, ( #35309, #2000, #29614 ),
 .UNSPECIFIED., .F., .F. ) 
 B_SPLINE_CURVE_WITH_KNOTS ( ( 3, 3 ),
 ( 0.000000000000000000, 1.000000000000000000 ),
 .UNSPECIFIED. ) 
 CURVE ( )  GEOMETRIC_REPRESENTATION_ITEM ( )  RATIONAL_B_SPLINE_CURVE ( ( 1.000000000000000000, 0.7071067811865474617, 1.000000000000000000 ) ) 
 REPRESENTATION_ITEM ( '' )  );
#26547=CARTESIAN_POINT ( 'NONE',  ( -14.04126239388531161, 8.106726622871482490, 20.82122704794079837 ) ) ;
#26548=EDGE_CURVE ( 'NONE', #10384, #21291, #39834, .T. ) ;
#26549=CARTESIAN_POINT ( 'NONE',  ( 23.61737546510263996, -7.194424252577891643, 20.99999999999999645 ) ) ;
#26550=CARTESIAN_POINT ( 'NONE',  ( 18.23649648353767461, -16.09146789626181118, 20.99999999999999645 ) ) ;
#26576=CARTESIAN_POINT ( 'NONE',  ( -23.43644022947910344, -8.137298067154993930, 22.99999999999999289 ) ) ;
#26598=CARTESIAN_POINT ( 'NONE',  ( 17.34253826607184479, 27.32041144404033162, 2.999999999999999112 ) ) ;
#26600=CARTESIAN_POINT ( 'NONE',  ( -5.496198527381525700, 34.39821714758459592, 18.87996532025786323 ) ) ;
#26617=CARTESIAN_POINT ( 'NONE',  ( -36.01097648505578519, -14.57711145883881620, 15.13084544680213384 ) ) ;
#26642=CARTESIAN_POINT ( 'NONE',  ( 35.28408311606053616, -16.24929212131948475, 15.72805884748936656 ) ) ;
#26644=CARTESIAN_POINT ( 'NONE',  ( 15.69115823232677620, 30.83414889893647626, 13.32518128616601061 ) ) ;
#26646=CARTESIAN_POINT ( 'NONE',  ( -15.48695972776671326, -26.74878859331622039, 16.30093088680190405 ) ) ;
#26648=CARTESIAN_POINT ( 'NONE',  ( -5.140622461635718565, 27.93365566737808692, 20.82122704794108259 ) ) ;
#26651=CARTESIAN_POINT ( 'NONE',  ( -4.817371740575545402, 23.83900317890010001, 20.99999999999999645 ) ) ;
#26656=CARTESIAN_POINT ( 'NONE',  ( 25.98021325959672723, -4.875178728621328617, 20.50957957746029336 ) ) ;
#26667=CARTESIAN_POINT ( 'NONE',  ( -28.63945468191068500, -5.523831429905184720, 19.99202127657074612 ) ) ;
#26687=CARTESIAN_POINT ( 'NONE',  ( -14.48927117870124270, -30.61587158504648087, 11.00000000000000000 ) ) ;
#26692=CARTESIAN_POINT ( 'NONE',  ( 29.18141975161354651, -3.595827299475466532, 19.27171037444328405 ) ) ;
#26715=CARTESIAN_POINT ( 'NONE',  ( 5.050662510305750530, -26.77689918168226058, 11.00000000000000000 ) ) ;
#26719=CARTESIAN_POINT ( 'NONE',  ( -20.92112759555556067, -16.07000418475133330, 20.99999999999999645 ) ) ;
#26729=CARTESIAN_POINT ( 'NONE',  ( -37.51589702892751887, -12.89337557385609401, 10.99999999999969269 ) ) ;
#26737=CARTESIAN_POINT ( 'NONE',  ( 23.05386822411318803, -7.747535282638377652, 23.00000000000000000 ) ) ;
#26743=CARTESIAN_POINT ( 'NONE',  ( 24.39151161285758107, -15.73551128733868865, 20.94377226548388293 ) ) ;
#26746=CARTESIAN_POINT ( 'NONE',  ( 36.53369576860743706, -5.154516326609254406, 11.00000000000007994 ) ) ;
#26790=B_SPLINE_CURVE_WITH_KNOTS ( 'NONE', 3,
 ( #30630, #21472, #30433, #36723, #8887, #9087, #18236, #39561, #24717, #21275, #27965, #6231, #2991, #14982, #20886, #33877, #33288, #27369 ),
 .UNSPECIFIED., .F., .F.,
 ( 4, 2, 2, 2, 2, 2, 2, 2, 4 ),
 ( 0.000000000000000000, 0.1249999999999998335, 0.2499999999999996669, 0.3749999999999995004, 0.4999999999999993339, 0.6249999999999994449, 0.7499999999999996669, 0.8749999999999997780, 1.000000000000000000 ),
 .UNSPECIFIED. ) ;
#26821=CARTESIAN_POINT ( 'NONE',  ( -27.69088631810926415, -26.08775134479659741, 15.13084544680184074 ) ) ;
#26824=ORIENTED_EDGE ( 'NONE', *, *, #3158, .F. ) ;
#26835=CARTESIAN_POINT ( 'NONE',  ( -34.30322546405390227, -21.55963432478805331, 11.00000000000007105 ) ) ;
#26842=CARTESIAN_POINT ( 'NONE',  ( 27.83556507003290648, -26.34944855520544493, 14.53008259253983070 ) ) ;
#26845=CARTESIAN_POINT ( 'NONE',  ( -13.15434222961970612, 33.66598129999007227, 14.53008259254024281 ) ) ;
#26847=CARTESIAN_POINT ( 'NONE',  ( 4.269643690484067594E-14, -24.31502561551697283, 16.87380292611441845 ) ) ;
#26849=CARTESIAN_POINT ( 'NONE',  ( 4.721973484737132409, 30.34170004520692032, 20.50957957746029692 ) ) ;
#26853=CARTESIAN_POINT ( 'NONE',  ( -8.768078002823386896, 24.93711404285670952, 20.50957957746029692 ) ) ;
#26858=CARTESIAN_POINT ( 'NONE',  ( 27.14644468510626041, -3.730463242941437496, 19.99202127657103389 ) ) ;
#26868=CARTESIAN_POINT ( 'NONE',  ( -31.98112326865703992, -15.20435932463186113, 18.87996532025782415 ) ) ;
#26892=CARTESIAN_POINT ( 'NONE',  ( 20.37435360786973959, -23.49902402743850871, 19.27171037444156099 ) ) ;
#26899=CARTESIAN_POINT ( 'NONE',  ( -15.37000524125038048, -27.20210912714572160, 15.72805884748939853 ) ) ;
#26915=CARTESIAN_POINT ( 'NONE',  ( -5.146739273647190416, -25.63390596715193936, 15.13084544680213739 ) ) ;
#26919=CARTESIAN_POINT ( 'NONE',  ( -20.02374874442591590, -18.66705478562314013, 20.82122704794079837 ) ) ;
#26930=CARTESIAN_POINT ( 'NONE',  ( -36.53368004180963169, -5.154483866377390200, 11.55979286843969511 ) ) ;
#26947=CARTESIAN_POINT ( 'NONE',  ( 19.96384346486630434, -17.84145166816523798, 20.94377226548378701 ) ) ;
#26951=CARTESIAN_POINT ( 'NONE',  ( 24.65531199400567175, -28.60128534115908749, 10.99999999999988987 ) ) ;
#26959=CARTESIAN_POINT ( 'NONE',  ( 4.817371740575539185, 23.83900317890011422, 20.99999999999999645 ) ) ;
#26988=CARTESIAN_POINT ( 'NONE',  ( -22.19961376577589718, 12.81695298357469426, 15.13084544680213561 ) ) ;
#26990=DIRECTION ( 'NONE',  ( -1.000000000000000000, 0.000000000000000000, 0.000000000000000000 ) ) ;
#27039=CARTESIAN_POINT ( 'NONE',  ( -37.48481798130409004, -12.61800288157225580, 10.99999999999995381 ) ) ;
#27046=CARTESIAN_POINT ( 'NONE',  ( 29.60586052328657303, -25.59238499873126216, 13.92931973827783843 ) ) ;
#27049=CARTESIAN_POINT ( 'NONE',  ( -13.38233516095408149, 33.85946688991404585, 13.92931973827825587 ) ) ;
#27050=CARTESIAN_POINT ( 'NONE',  ( 12.15426487969635261, -15.33773963132624552, 20.99999999999999645 ) ) ;
#27053=CARTESIAN_POINT ( 'NONE',  ( 7.962467718761615743, 24.71319220551615459, 20.69868183039781329 ) ) ;
#27062=CARTESIAN_POINT ( 'NONE',  ( 11.85876577156197165, 19.91979463203424672, 19.99202127657068218 ) ) ;
#27064=CARTESIAN_POINT ( 'NONE',  ( 12.44178368932927015, 35.65276919561884483, 10.99999999999994493 ) ) ;
#27071=CARTESIAN_POINT ( 'NONE',  ( -31.37624276535950330, -18.11508220673910685, 18.42518152272108622 ) ) ;
#27076=VERTEX_POINT ( 'NONE', #10972 ) ;
#27082=VECTOR ( 'NONE', #34877, 1000.000000000000000 ) ;
#27086=CARTESIAN_POINT ( 'NONE',  ( 23.05386822411317027, -7.747535282638454035, 23.00000000000000000 ) ) ;
#27096=CARTESIAN_POINT ( 'NONE',  ( 31.11751882148445603, -7.091474513517732170, 19.27171037444123414 ) ) ;
#27117=CARTESIAN_POINT ( 'NONE',  ( 4.238566308745586637E-14, -25.93120163663720845, 14.53008259254011136 ) ) ;
#27120=CARTESIAN_POINT ( 'NONE',  ( -26.13185812888372794, -11.12779425996339988, 20.94377226548397886 ) ) ;
#27130=CARTESIAN_POINT ( 'NONE',  ( -16.87498849720607552, -29.16588574430774017, 10.99999999999931433 ) ) ;
#27133=CARTESIAN_POINT ( 'NONE',  ( -24.22138565352712902, -9.557272464391486366, 20.99999999999999289 ) ) ;
#27135=EDGE_CURVE ( 'NONE', #12781, #10973, #3216, .T. ) ;
#27148=CARTESIAN_POINT ( 'NONE',  ( 21.14791330573125805, -16.83114732581536899, 21.00000000000004619 ) ) ;
#27160=CARTESIAN_POINT ( 'NONE',  ( 13.22866120778972387, 26.17694675929307735, 18.42518152272108978 ) ) ;
#27163=DIRECTION ( 'NONE',  ( -0.000000000000000000, -0.000000000000000000, -1.000000000000000000 ) ) ;
#27164=CARTESIAN_POINT ( 'NONE',  ( -4.881458130668121953, -28.77689918168226413, 22.99999999999999645 ) ) ;
#27188=CARTESIAN_POINT ( 'NONE',  ( -28.53381226739762511, 4.748233269558084224, 13.32518128617320130 ) ) ;
#27242=CARTESIAN_POINT ( 'NONE',  ( 37.03605016780974069, -10.92602907108481958, 13.92931973827803738 ) ) ;
#27244=CARTESIAN_POINT ( 'NONE',  ( -11.65184672540978639, 34.81748849094240228, 15.13084544680287813 ) ) ;
#27245=CARTESIAN_POINT ( 'NONE',  ( 5.799013854623458641, -17.87737810982027398, 20.50957957746029336 ) ) ;
#27249=CARTESIAN_POINT ( 'NONE',  ( 6.855490822441819176, 29.74656830693212939, 20.25080042701566896 ) ) ;
#27251=DIRECTION ( 'NONE',  ( -0.000000000000000000, -0.000000000000000000, -1.000000000000000000 ) ) ;
#27253=CARTESIAN_POINT ( 'NONE',  ( -17.28285333400955182, 27.30382183500235627, 12.14047268033097815 ) ) ;
#27258=CARTESIAN_POINT ( 'NONE',  ( 25.38348611796501686, -5.460896781496693997, 20.69868183039781329 ) ) ;
#27260=CARTESIAN_POINT ( 'NONE',  ( -7.591957726968679765, 38.93640765974109996, 10.99999999999981348 ) ) ;
#27270=CARTESIAN_POINT ( 'NONE',  ( -21.96133346275663456, -24.83662088761592202, 18.42518152272072740 ) ) ;
#27296=CARTESIAN_POINT ( 'NONE',  ( 33.92416433109537621, -10.98373637526195168, 17.92354375535250455 ) ) ;
#27302=CYLINDRICAL_SURFACE ( 'NONE', #36232, 60.00000000000007105 ) ;
#27314=CARTESIAN_POINT ( 'NONE',  ( 5.146739273647275681, -25.63390596715193936, 15.13084544680213739 ) ) ;
#27317=CARTESIAN_POINT ( 'NONE',  ( -25.43307211745671736, -8.368469763667990335, 20.94377226548378346 ) ) ;
#27343=CARTESIAN_POINT ( 'NONE',  ( 26.67038870798830885, -5.578326634889591240, 20.50957957746141958 ) ) ;
#27355=CARTESIAN_POINT ( 'NONE',  ( 15.87271491999988804, 26.91186955879557985, 15.72805884748939143 ) ) ;
#27369=CARTESIAN_POINT ( 'NONE',  ( 23.05386822411318803, -7.747535282638377652, 20.99999999999999645 ) ) ;
#27381=ORIENTED_EDGE ( 'NONE', *, *, #36702, .F. ) ;
#27396=CARTESIAN_POINT ( 'NONE',  ( 20.66414367075948277, 17.76245163070630184, 10.99999999999898037 ) ) ;
#27422=CARTESIAN_POINT ( 'NONE',  ( -39.48531003256149319, -11.24999992065011156, 11.00000000000000000 ) ) ;
#27441=CARTESIAN_POINT ( 'NONE',  ( 13.65033576027476414, 34.08684981564654493, 12.73282698324863738 ) ) ;
#27442=CARTESIAN_POINT ( 'NONE',  ( 11.73759695151994009, -17.78600041297262635, 20.69868183039754328 ) ) ;
#27444=ADVANCED_FACE ( 'NONE', ( #15609 ), #21310, .T. ) ;
#27445=CARTESIAN_POINT ( 'NONE',  ( -4.528037020496219256, 32.30201321073018050, 19.99202127657103389 ) ) ;
#27455=CARTESIAN_POINT ( 'NONE',  ( 16.89748511972537770, 9.755767582501292168, 19.99202127657103389 ) ) ;
#27465=CARTESIAN_POINT ( 'NONE',  ( -32.91936639158274858, -8.047070124328334018, 18.42518152272033660 ) ) ;
#27479=CARTESIAN_POINT ( 'NONE',  ( 38.66460482714475688, -17.32098561216329458, 11.00000000000000000 ) ) ;
#27490=CARTESIAN_POINT ( 'NONE',  ( 32.65234849725225530, -15.41672394535051893, 18.42518152272110044 ) ) ;
#27497=CARTESIAN_POINT ( 'NONE',  ( -16.60464863832890003, -22.41657912773202099, 19.66345542862528717 ) ) ;
#27511=CARTESIAN_POINT ( 'NONE',  ( 15.03860650580597991, -28.48662463501975139, 12.73282698324853257 ) ) ;
#27515=CARTESIAN_POINT ( 'NONE',  ( -21.62094419769859144, -18.41873747672905282, 20.82122704794093693 ) ) ;
#27543=CARTESIAN_POINT ( 'NONE',  ( 26.17801803039862918, -8.007547698857949925, 20.82122704794080903 ) ) ;
#27575=CARTESIAN_POINT ( 'NONE',  ( -20.72701401736282989, -28.35932241216953287, 14.53008259254010959 ) ) ;
#27586=CARTESIAN_POINT ( 'NONE',  ( -32.18944385490033255, 1.219497045965482140, 12.73282698324853079 ) ) ;
#27638=CARTESIAN_POINT ( 'NONE',  ( 23.05386822411318803, -7.747535282638377652, 23.00000000000000000 ) ) ;
#27642=CARTESIAN_POINT ( 'NONE',  ( 3.827636526755794577, 39.84991882288247211, 13.32518128616622555 ) ) ;
#27643=CARTESIAN_POINT ( 'NONE',  ( -5.869341256201681567, -17.04122685614420263, 20.69868183039781684 ) ) ;
#27645=CARTESIAN_POINT ( 'NONE',  ( 8.810137414575107684, 27.17888719461359415, 20.25080042701567251 ) ) ;
#27647=EDGE_LOOP ( 'NONE', ( #14211, #21350, #28806, #23848 ) ) ;
#27649=CARTESIAN_POINT ( 'NONE',  ( -17.01882136418225500, 27.23043334310857588, 13.32518128616609054 ) ) ;
#27664=CARTESIAN_POINT ( 'NONE',  ( -33.25367603495013213, -15.60696645162129315, 17.92354375535250810 ) ) ;
#27676=CARTESIAN_POINT ( 'NONE',  ( 31.08218589456554071, -27.68808744834075597, 11.00000000000000000 ) ) ;
#27686=CARTESIAN_POINT ( 'NONE',  ( 24.51396478725026640, -11.15767879383071026, 21.00000000000001066 ) ) ;
#27687=CARTESIAN_POINT ( 'NONE',  ( 33.86703583613424939, -12.56047426484072993, 17.92354375535250455 ) ) ;
#27691=DIRECTION ( 'NONE',  ( -0.000000000000000000, -0.000000000000000000, -1.000000000000000000 ) ) ;
#27692=CARTESIAN_POINT ( 'NONE',  ( -33.88090307477148855, -0.3823557797707961003, 10.99999999999973355 ) ) ;
#27696=CARTESIAN_POINT ( 'NONE',  ( 32.18944385490472371, 1.219497045960946657, 12.73282698324853257 ) ) ;
#27708=CARTESIAN_POINT ( 'NONE',  ( -21.38319344285576662, -17.62079982023109181, 20.94377226548387938 ) ) ;
#27738=CARTESIAN_POINT ( 'NONE',  ( 21.12676075887526750, -20.25532016563445481, 20.50957957746029692 ) ) ;
#27750=CARTESIAN_POINT ( 'NONE',  ( -6.462764152204137247, 17.91932574235844555, 23.00000000000000000 ) ) ;
#27773=CARTESIAN_POINT ( 'NONE',  ( -36.59387134601861646, -14.69446750445176342, 13.92931973827808712 ) ) ;
#27788=CARTESIAN_POINT ( 'NONE',  ( -17.89938016360686390, 22.15910768086194693, 14.53008259255394208 ) ) ;
#27798=CARTESIAN_POINT ( 'NONE',  ( 30.33922525720639030, 6.243664897696307392, 11.00000000000000000 ) ) ;
#27815=CARTESIAN_POINT ( 'NONE',  ( -3.456468065140151591, 26.15323006594331545, 23.00000000000000000 ) ) ;
#27834=DIRECTION ( 'NONE',  ( 1.000000000000000000, 0.000000000000000000, 0.000000000000000000 ) ) ;
#27844=CARTESIAN_POINT ( 'NONE',  ( -13.54523449123470691, 33.99770581697566740, 13.32518128616629483 ) ) ;
#27845=CARTESIAN_POINT ( 'NONE',  ( -17.00801676778996097, -20.85310720624647374, 20.25080042701566541 ) ) ;
#27847=CARTESIAN_POINT ( 'NONE',  ( -5.145977874761546111, 31.04572515097865804, 20.25080042701513960 ) ) ;
#27866=CARTESIAN_POINT ( 'NONE',  ( -26.47427689499508574, -23.88731992525624293, 17.92354375535214572 ) ) ;
#27889=CARTESIAN_POINT ( 'NONE',  ( 26.16909114927596747, -23.33537003677559696, 18.42518152272070253 ) ) ;
#27899=CARTESIAN_POINT ( 'NONE',  ( 28.74551992320437321, 4.923758765711149010, 12.14047268032575211 ) ) ;
#27910=CARTESIAN_POINT ( 'NONE',  ( -26.24102572421938362, -17.42682220599465737, 20.50957957746029692 ) ) ;
#27938=CARTESIAN_POINT ( 'NONE',  ( 25.62037635619481790, -16.85925998830611761, 20.69868183039799803 ) ) ;
#27946=CARTESIAN_POINT ( 'NONE',  ( -22.48079666814428634, 18.61591633949074520, 22.99999999999999645 ) ) ;
#27965=CARTESIAN_POINT ( 'NONE',  ( 28.78471548569376282, -2.122417091767359931, 18.87996532025784546 ) ) ;
#27970=CARTESIAN_POINT ( 'NONE',  ( -22.57842393431380756, -28.22498519091902125, 14.53008259253967971 ) ) ;
#27980=ADVANCED_FACE ( 'NONE', ( #1778 ), #15616, .T. ) ;
#27981=CARTESIAN_POINT ( 'NONE',  ( -14.97058623677449773, 26.66112013779128986, 16.87380292611441490 ) ) ;
#27987=CARTESIAN_POINT ( 'NONE',  ( 32.43957513061237563, -23.09559191376027343, 13.92931973827834113 ) ) ;
#28040=CARTESIAN_POINT ( 'NONE',  ( 7.565838454495062315, 38.87983827381772528, 12.14047268033080407 ) ) ;
#28044=CARTESIAN_POINT ( 'NONE',  ( -2.905187527479620613, 31.12430299512148935, 20.50957957746028626 ) ) ;
#28061=CARTESIAN_POINT ( 'NONE',  ( -15.89892447185300917, -25.15199583021655272, 17.92354375535250810 ) ) ;
#28065=ORIENTED_EDGE ( 'NONE', *, *, #31991, .T. ) ;
#28073=CARTESIAN_POINT ( 'NONE',  ( 23.09341953181412421, -31.04079623447207581, 11.00000000000000000 ) ) ;
#28084=CARTESIAN_POINT ( 'NONE',  ( 31.14237565978548616, -19.77424633423373024, 17.92354375535250455 ) ) ;
#28096=CARTESIAN_POINT ( 'NONE',  ( 16.52773037515250465, 27.09393310381576114, 14.53008259254011136 ) ) ;
#28107=CARTESIAN_POINT ( 'NONE',  ( -24.27776115474302543, -18.04224162735225079, 20.69868183039780973 ) ) ;
#28109=DIRECTION ( 'NONE',  ( -1.000000000000000000, 0.000000000000000000, 0.000000000000000000 ) ) ;
#28135=CARTESIAN_POINT ( 'NONE',  ( 26.32839453010175035, -14.27099112026796135, 20.82122704794079837 ) ) ;
#28137=ADVANCED_FACE ( 'NONE', ( #918 ), #7402, .F. ) ;
#28143=PLANE ( 'NONE',  #13237 ) ;
#28144=CARTESIAN_POINT ( 'NONE',  ( -22.48079666815685940, 18.61591633949185010, 11.00000000000000000 ) ) ;
#28170=CARTESIAN_POINT ( 'NONE',  ( -37.03648387062790448, -7.065924075330933363, 12.14047268033043991 ) ) ;
#28181=CARTESIAN_POINT ( 'NONE',  ( -20.03472765055071036, 11.56705540218451311, 17.92354375535250810 ) ) ;
#28187=CARTESIAN_POINT ( 'NONE',  ( 20.74852905477029452, -28.65583854707664457, 13.92931973827808356 ) ) ;
#28188=VERTEX_POINT ( 'NONE', #10458 ) ;
#28192=FACE_OUTER_BOUND ( 'NONE', #20897, .T. ) ;
#28195=ORIENTED_EDGE ( 'NONE', *, *, #28784, .F. ) ;
#28208=CARTESIAN_POINT ( 'NONE',  ( 13.82587226056084262, 37.11292026376988673, 11.00000000000000000 ) ) ;
#28232=CARTESIAN_POINT ( 'NONE',  ( -37.48531001978128074, -11.24999991186452775, 11.00000000000002309 ) ) ;
#28243=CARTESIAN_POINT ( 'NONE',  ( 17.15083734909593360, 27.26712758905532752, 12.73282698324853257 ) ) ;
#28246=CARTESIAN_POINT ( 'NONE',  ( -7.971538940947521468, 30.92644086613018928, 19.66345542862593376 ) ) ;
#28264=CARTESIAN_POINT ( 'NONE',  ( -31.01938180031993753, -21.79666295253727171, 16.87380292611439359 ) ) ;
#28286=CARTESIAN_POINT ( 'NONE',  ( 24.49409870379991716, -11.70597971641862856, 21.00000000000001776 ) ) ;
#28287=CARTESIAN_POINT ( 'NONE',  ( 32.10122455788091145, -20.47530094824173474, 16.87380292611440424 ) ) ;
#28291=CARTESIAN_POINT ( 'NONE',  ( 3.428976547226190608, 28.19475011768619055, 20.94377226548378346 ) ) ;
#28305=CARTESIAN_POINT ( 'NONE',  ( -27.53764137322051297, -17.13852093243013996, 20.25080042701539540 ) ) ;
#28327=VERTEX_POINT ( 'NONE', #26505 ) ;
#28330=CARTESIAN_POINT ( 'NONE',  ( 29.45937559703822473, -11.06631500863537454, 20.25080042701566185 ) ) ;
#28364=CARTESIAN_POINT ( 'NONE',  ( -35.50541758542772186, -3.488475578028477742, 12.73282698324853257 ) ) ;
#28371=CARTESIAN_POINT ( 'NONE',  ( -11.91493164750346700, 32.61411734499214532, 16.87380292611442201 ) ) ;
#28376=CARTESIAN_POINT ( 'NONE',  ( -18.42861860568109833, 16.71074749267419435, 16.87380292611394239 ) ) ;
#28386=CARTESIAN_POINT ( 'NONE',  ( 37.00900745416906545, -9.025932648522378088, 13.32518128616608877 ) ) ;
#28391=DIRECTION ( 'NONE',  ( 1.000000000000000000, 0.000000000000000000, 0.000000000000000000 ) ) ;
#28438=CARTESIAN_POINT ( 'NONE',  ( -16.82090372984253435, 29.19711159930247746, 11.55979286843847653 ) ) ;
#28442=CARTESIAN_POINT ( 'NONE',  ( 10.24444524355854291, 27.94074263397462232, 19.66345542862530493 ) ) ;
#28455=CARTESIAN_POINT ( 'NONE',  ( 4.441848239913459118, 24.85865334748800137, 21.00000000000001066 ) ) ;
#28461=CARTESIAN_POINT ( 'NONE',  ( -31.91928157790810516, -18.42860581134450726, 17.92354375535250810 ) ) ;
#28483=CARTESIAN_POINT ( 'NONE',  ( 23.19735768193467962, -14.64350930037813647, 20.99999999999999289 ) ) ;
#28484=CARTESIAN_POINT ( 'NONE',  ( 27.04902410904039556, -24.92680750149222746, 16.87380292611402055 ) ) ;
#28487=CARTESIAN_POINT ( 'NONE',  ( 3.003889247183332056, 27.48891118973832448, 20.99999999999999645 ) ) ;
#28497=CARTESIAN_POINT ( 'NONE',  ( 32.33143948541787438, 1.358872982501808435, 11.00000000000000000 ) ) ;
#28505=CARTESIAN_POINT ( 'NONE',  ( -20.20329687195632218, -21.14155277498739594, 20.25080042701566541 ) ) ;
#28533=CARTESIAN_POINT ( 'NONE',  ( 25.71034552362537084, -20.07240169439175403, 19.99202127657074257 ) ) ;
#28559=CARTESIAN_POINT ( 'NONE',  ( 28.24711154207322750, -27.09388640670316661, 11.00000000000010303 ) ) ;
#28568=CARTESIAN_POINT ( 'NONE',  ( -34.78244346405214316, -1.681994768166323428, 12.14047268033058558 ) ) ;
#28576=CARTESIAN_POINT ( 'NONE',  ( 14.52022913576961116, 28.28138333486318601, 16.87380292611584665 ) ) ;
#28579=CARTESIAN_POINT ( 'NONE',  ( -27.71565130972192392, -3.171757977838549625, 19.66345542862528717 ) ) ;
#28581=FACE_OUTER_BOUND ( 'NONE', #27647, .T. ) ;
#28582=CARTESIAN_POINT ( 'NONE',  ( 24.51445621669102692, -11.16206880503134080, 23.00000000000000355 ) ) ;
#28587=CARTESIAN_POINT ( 'NONE',  ( 32.18944385490208759, 1.219497045963512827, 12.73282698324853257 ) ) ;
#28619=CARTESIAN_POINT ( 'NONE',  ( -75.15099915297791711, 43.38844959084113384, 2.999999999999999112 ) ) ;
#28631=CARTESIAN_POINT ( 'NONE',  ( -31.24272016124700713, 0.2902395683534712556, 15.72805884748939143 ) ) ;
#28640=CARTESIAN_POINT ( 'NONE',  ( -1.473879933410623262E-13, 40.50000000000004974, 11.55979286843934872 ) ) ;
#28644=CARTESIAN_POINT ( 'NONE',  ( -2.660873612011868339, 34.56296969693360666, 19.27171037444157875 ) ) ;
#28661=CARTESIAN_POINT ( 'NONE',  ( -24.21699896819899678, -27.13078975446515528, 15.72805884748972360 ) ) ;
#28684=CARTESIAN_POINT ( 'NONE',  ( 20.64393337882627577, -27.21432092515273382, 16.30093088680190760 ) ) ;
#28686=CARTESIAN_POINT ( 'NONE',  ( 3.569741787452879400, 38.68155838841062888, 15.72805884748945360 ) ) ;
#28689=CARTESIAN_POINT ( 'NONE',  ( 3.503066876655847040, 27.10955750621999982, 20.99999999999999645 ) ) ;
#28694=CARTESIAN_POINT ( 'NONE',  ( 17.35626706996901092, 16.20628521381938469, 17.92354375535268929 ) ) ;
#28704=CARTESIAN_POINT ( 'NONE',  ( -29.45937559703918751, -11.06631500863563922, 20.25080042701617344 ) ) ;
#28730=CARTESIAN_POINT ( 'NONE',  ( 24.71109915377187605, -20.69862126830684801, 19.99202127657072481 ) ) ;
#28760=CYLINDRICAL_SURFACE ( 'NONE', #26294, 17.99999999999992895 ) ;
#28769=CARTESIAN_POINT ( 'NONE',  ( -32.09165771328245853, 1.123514972296517422, 13.32518128616608699 ) ) ;
#28776=CARTESIAN_POINT ( 'NONE',  ( 4.331888841169166504, 42.14502281828541896, 11.00000000000000000 ) ) ;
#28777=CARTESIAN_POINT ( 'NONE',  ( -3.110808594360106927, 36.60201144129489137, 17.92354375535252586 ) ) ;
#28782=CARTESIAN_POINT ( 'NONE',  ( -15.42165057838969666, 26.78649484828442695, 16.30093088680190405 ) ) ;
#28784=EDGE_CURVE ( 'NONE', #22892, #1139, #21853, .T. ) ;
#28785=CARTESIAN_POINT ( 'NONE',  ( 18.76090689389213395, -16.22676322417229500, 20.99999999999999645 ) ) ;
#28786=PRODUCT_DEFINITION_FORMATION_WITH_SPECIFIED_SOURCE ( 'ANY', '', #37908, .NOT_KNOWN. ) ;
#28789=CARTESIAN_POINT ( 'NONE',  ( 33.64699323788449448, -0.06984207429561786751, 12.14047268033164073 ) ) ;
#28793=DIRECTION ( 'NONE',  ( 0.000000000000000000, 0.000000000000000000, 1.000000000000000000 ) ) ;
#28806=ORIENTED_EDGE ( 'NONE', *, *, #39443, .F. ) ;
#28810=CARTESIAN_POINT ( 'NONE',  ( 4.331888854854090809, 42.14502281367550296, 11.00000000000000000 ) ) ;
#28816=CARTESIAN_POINT ( 'NONE',  ( -18.76572289696387941, -16.22800572947405584, 23.00000000000000355 ) ) ;
#28828=ORIENTED_EDGE ( 'NONE', *, *, #13359, .F. ) ;
#28843=CARTESIAN_POINT ( 'NONE',  ( -9.574495036671709640E-14, 34.03222469610383882, 19.66345542862528362 ) ) ;
#28863=CARTESIAN_POINT ( 'NONE',  ( -30.06723386280177124, -23.25956985441318636, 16.30093088680191116 ) ) ;
#28882=CARTESIAN_POINT ( 'NONE',  ( -39.48531003256149319, -11.24999992065011156, 11.00000000000000000 ) ) ;
#28886=CARTESIAN_POINT ( 'NONE',  ( 15.48695972777691310, -26.74878859331900927, 16.30093088680190405 ) ) ;
#28889=CARTESIAN_POINT ( 'NONE',  ( -1.412590157703688977E-13, 38.50629078351121137, 16.30093088680190405 ) ) ;
#28893=CARTESIAN_POINT ( 'NONE',  ( 4.002244506128361579, 26.73020382270167516, 20.99999999999999645 ) ) ;
#28900=CARTESIAN_POINT ( 'NONE',  ( 15.26743640727520557, 21.18345451738099428, 17.92354375534863209 ) ) ;
#28908=CARTESIAN_POINT ( 'NONE',  ( -30.12142568021468136, -17.39061322484690919, 19.27171037444157164 ) ) ;
#28933=CARTESIAN_POINT ( 'NONE',  ( 29.41993030479209281, -12.15499915640502948, 20.25080042701565475 ) ) ;
#28956=CARTESIAN_POINT ( 'NONE',  ( -23.31304291943800067, -15.59395685184293967, 21.00000000000000000 ) ) ;
#28969=CARTESIAN_POINT ( 'NONE',  ( -31.25372621196067513, -24.60616950719562723, 12.73282698324853079 ) ) ;
#28978=CARTESIAN_POINT ( 'NONE',  ( -13.83280510892178938, 26.34487040058245455, 17.92354375535250810 ) ) ;
#28989=CARTESIAN_POINT ( 'NONE',  ( 32.84658669524299768, -23.46788009898371996, 11.55979286843938958 ) ) ;
#29025=CARTESIAN_POINT ( 'NONE',  ( -24.28032989564857047, -12.76774640304084585, 21.00000000000000000 ) ) ;
#29034=CARTESIAN_POINT ( 'NONE',  ( -31.51573171626090186, 0.5582143012903737489, 15.13084544680213739 ) ) ;
#29037=ORIENTED_EDGE ( 'NONE', *, *, #12511, .T. ) ;
#29041=CARTESIAN_POINT ( 'NONE',  ( 12.44178368932912093, 35.65276919561900826, 10.99999999999994316 ) ) ;
#29044=CARTESIAN_POINT ( 'NONE',  ( 1.329271672591037179, 34.78122644969443655, 19.27171037444156454 ) ) ;
#29052=CARTESIAN_POINT ( 'NONE',  ( -18.69515074622357176, 22.45407711376243753, 11.00000000002426148 ) ) ;
#29057=CARTESIAN_POINT ( 'NONE',  ( 6.143904198944456496, -13.77689918168226058, 20.99999999999998934 ) ) ;
#29059=EDGE_CURVE ( 'NONE', #25190, #14259, #16546, .T. ) ;
#29065=CARTESIAN_POINT ( 'NONE',  ( -22.45592429723070893, -27.55223906713353088, 15.72805884748896688 ) ) ;
#29089=CARTESIAN_POINT ( 'NONE',  ( 34.90004137879596868, -9.293601764822927436, 16.87380292611441845 ) ) ;
#29092=CARTESIAN_POINT ( 'NONE',  ( 8.548670570950529068, 36.69528512485702976, 15.72805884748941807 ) ) ;
#29094=CARTESIAN_POINT ( 'NONE',  ( -5.178899460637612862, -25.25135431486990711, 15.72805884748939853 ) ) ;
#29096=CARTESIAN_POINT ( 'NONE',  ( -4.817371740575544514, 23.83900317890010001, 20.99999999999999645 ) ) ;
#29103=CARTESIAN_POINT ( 'NONE',  ( 13.22866120778439125, 26.17694675931205595, 18.42518152272108978 ) ) ;
#29112=CARTESIAN_POINT ( 'NONE',  ( -27.96047413129358006, -4.559793092419412552, 19.99202127657104455 ) ) ;
#29132=CARTESIAN_POINT ( 'NONE',  ( -18.23649648353780961, -16.09146789626144169, 23.00000000000000000 ) ) ;
#29138=CARTESIAN_POINT ( 'NONE',  ( 22.33353841799053541, -20.81031336111236740, 20.25080042701592475 ) ) ;
#29142=( BOUNDED_SURFACE ( )  B_SPLINE_SURFACE ( 2, 3, ( 
 ( #9114, #18856, #37143, #373, #27798, #30854 ),
 ( #31445, #9317, #12752, #18661, #31053, #22291 ),
 ( #6059, #9718, #3218, #22098, #6844, #6646 ) ),
 .UNSPECIFIED., .F., .F., .F. ) 
 B_SPLINE_SURFACE_WITH_KNOTS ( ( 3, 3 ),
 ( 4, 2, 4 ),
 ( 0.000000000000000000, 1.000000000000000000 ),
 ( 3.412702215524944904, 3.665191429188091377, 3.917680642851237405 ),
 .UNSPECIFIED. ) 
 GEOMETRIC_REPRESENTATION_ITEM ( )  RATIONAL_B_SPLINE_SURFACE ( (
 ( 1.000000000000000000, 1.000000000000000000, 1.000000000000000000, 1.000000000000000000, 1.000000000000000000, 1.000000000000000000),
 ( 0.7071067811865474617, 0.7071067811865474617, 0.7071067811865474617, 0.7071067811865474617, 0.7071067811865474617, 0.7071067811865474617),
 ( 1.000000000000000000, 1.000000000000000000, 1.000000000000000000, 1.000000000000000000, 1.000000000000000000, 1.000000000000000000) ) ) 
 REPRESENTATION_ITEM ( '' )  SURFACE ( )  );
#29164=CARTESIAN_POINT ( 'NONE',  ( -23.98526753813956347, -9.069922861307588846, 20.99999999999999645 ) ) ;
#29178=CARTESIAN_POINT ( 'NONE',  ( -37.45384686740443669, -12.88771083438535214, 12.14047268033070992 ) ) ;
#29186=CARTESIAN_POINT ( 'NONE',  ( 11.91494638969559361, 32.61409561180352057, 16.87380292611443977 ) ) ;
#29189=CARTESIAN_POINT ( 'NONE',  ( -22.54917513128955164, -0.2132175735129904770, 20.25080042701864969 ) ) ;
#29195=CARTESIAN_POINT ( 'NONE',  ( 34.90171719354076885, -20.15051581687074034, 12.73282698324853257 ) ) ;
#29227=CARTESIAN_POINT ( 'NONE',  ( -24.37759566069507855, -10.08322588119030172, 20.99999999999999645 ) ) ;
#29236=CARTESIAN_POINT ( 'NONE',  ( -28.78471548568729688, -2.122417091760708807, 18.87996532025785257 ) ) ;
#29246=CARTESIAN_POINT ( 'NONE',  ( -1.947644445291446980, 40.50000000000003553, 11.55979286843934695 ) ) ;
#29249=CARTESIAN_POINT ( 'NONE',  ( -11.57512167954172355, 28.64755075779800464, 18.87996532025787388 ) ) ;
#29270=CARTESIAN_POINT ( 'NONE',  ( -35.98781724630784140, -12.75392035872630991, 15.72805884748931859 ) ) ;
#29293=CARTESIAN_POINT ( 'NONE',  ( 30.62963707967951166, -23.89786472172307086, 15.13084544680214094 ) ) ;
#29296=CARTESIAN_POINT ( 'NONE',  ( 1.732136883776949521, 38.50629078351121137, 16.30093088680190760 ) ) ;
#29297=CARTESIAN_POINT ( 'NONE',  ( 15.89892447185634339, -25.15199583021764695, 17.92354375535250810 ) ) ;
#29299=CARTESIAN_POINT ( 'NONE',  ( 6.290729337820269329, 29.14951258272645163, 20.50957957746029692 ) ) ;
#29306=CARTESIAN_POINT ( 'NONE',  ( 18.88552629894499546, 10.90356369248356572, 18.87996532025784902 ) ) ;
#29316=CARTESIAN_POINT ( 'NONE',  ( -26.58217467610690932, -19.30423083005489104, 19.99202127657103389 ) ) ;
#29330=CARTESIAN_POINT ( 'NONE',  ( 24.28032989564874811, -12.76774640304083874, 23.00000000000000000 ) ) ;
#29339=CARTESIAN_POINT ( 'NONE',  ( 30.06493440560372221, -18.98646248983848395, 18.87996532025784546 ) ) ;
#29359=CARTESIAN_POINT ( 'NONE',  ( -23.54493052986481771, -14.21898406159468742, 20.99999999999999645 ) ) ;
#29371=CARTESIAN_POINT ( 'NONE',  ( -34.10020663062403656, -21.93670956716201914, 11.55979286843944820 ) ) ;
#29385=CARTESIAN_POINT ( 'NONE',  ( -11.85876577173794466, 19.91979463210470769, 19.99202127657087402 ) ) ;
#29387=CARTESIAN_POINT ( 'NONE',  ( 24.81299795227012339, -13.60183200321584707, 20.99999999999999645 ) ) ;
#29392=CARTESIAN_POINT ( 'NONE',  ( 32.69891748962707112, -23.33280782877936943, 12.73282698324868356 ) ) ;
#29410=EDGE_LOOP ( 'NONE', ( #14780, #37860, #38866, #2683, #5059, #3499, #26824 ) ) ;
#29419=EDGE_CURVE ( 'NONE', #4088, #24813, #35112, .T. ) ;
#29446=CARTESIAN_POINT ( 'NONE',  ( 11.00934640754938165, 31.84548813490947694, 17.92354375535252231 ) ) ;
#29456=CARTESIAN_POINT ( 'NONE',  ( 18.23649648353767461, -16.09146789626181118, 20.99999999999999645 ) ) ;
#29461=EDGE_CURVE ( 'NONE', #24176, #36229, #4877, .T. ) ;
#29465=CARTESIAN_POINT ( 'NONE',  ( -23.94800771174391585, -26.22823558801417221, 16.87380292611477728 ) ) ;
#29491=CARTESIAN_POINT ( 'NONE',  ( 34.34163329534274567, -19.82715122747730163, 14.53008259254011136 ) ) ;
#29493=CARTESIAN_POINT ( 'NONE',  ( -15.39524332971155474, 28.62968336403564962, 15.72805884748878746 ) ) ;
#29495=CARTESIAN_POINT ( 'NONE',  ( -15.74227866052810221, -25.75916161678033234, 17.42190598798392998 ) ) ;
#29499=CARTESIAN_POINT ( 'NONE',  ( 1.790359260782300899, 30.61752677313665671, 20.69868183039780973 ) ) ;
#29506=CARTESIAN_POINT ( 'NONE',  ( 21.61978140912328072, 6.167694920802003544, 18.87996532025766783 ) ) ;
#29517=CARTESIAN_POINT ( 'NONE',  ( -29.65272772477494101, -7.615234770328493497, 19.99202127657132522 ) ) ;
#29536=CARTESIAN_POINT ( 'NONE',  ( -24.22138565352702955, -9.557272464391553868, 23.00000000000000000 ) ) ;
#29541=CARTESIAN_POINT ( 'NONE',  ( 26.60725962520467647, -21.34341596033631561, 19.27171037444124480 ) ) ;
#29564=CARTESIAN_POINT ( 'NONE',  ( -23.78345815580402345, -15.17947280105380514, 21.00000000000000000 ) ) ;
#29574=CARTESIAN_POINT ( 'NONE',  ( -36.68766582957241695, -16.69324967293977124, 12.14047268033123750 ) ) ;
#29576=AXIS2_PLACEMENT_3D ( 'NONE', #39208, #32928, #21327 ) ;
#29582=CARTESIAN_POINT ( 'NONE',  ( -10.37659643210535698, 39.73422260934387396, 11.00000000000000355 ) ) ;
#29587=CARTESIAN_POINT ( 'NONE',  ( -21.91791918718876175, -0.7365302467875901593, 20.50957957746284066 ) ) ;
#29588=CARTESIAN_POINT ( 'NONE',  ( 23.74914942275264096, -8.582573258223899160, 20.99999999999999645 ) ) ;
#29614=CARTESIAN_POINT ( 'NONE',  ( -14.48927117870122316, -30.61587158504648087, 11.00000000000000000 ) ) ;
#29619=( BOUNDED_SURFACE ( )  B_SPLINE_SURFACE ( 2, 3, ( 
 ( #24569, #36964, #18675, #9128, #3030, #6073, #21714, #21515, #9332, #18478, #20923, #182, #15422, #27815, #32058, #3231, #12372, #37158 ),
 ( #34116, #15622, #12571, #24963, #5475, #37357, #3425, #25756, #22502, #15821, #6860, #16225, #37955, #22111, #10127, #38152, #35108, #4228 ),
 ( #21908, #9927, #34511, #37559, #28208, #9730, #6660, #28810, #16630, #25162, #31857, #387, #12964, #6466, #13567, #3625, #31660, #31459 ) ),
 .UNSPECIFIED., .F., .F., .F. ) 
 B_SPLINE_SURFACE_WITH_KNOTS ( ( 3, 3 ),
 ( 4, 2, 2, 2, 2, 2, 2, 2, 4 ),
 ( 0.000000000000000000, 1.000000000000000000 ),
 ( 0.2711095619351563957, 0.5960312531500917554, 0.9209529443650270597, 1.245874635579962364, 1.570796326794897668, 1.895718018009833195, 2.220639709224768499, 2.545561400439703803, 2.870483091654639107 ),
 .UNSPECIFIED. ) 
 GEOMETRIC_REPRESENTATION_ITEM ( )  RATIONAL_B_SPLINE_SURFACE ( (
 ( 1.000000000000000000, 1.000000000000000000, 1.000000000000000000, 1.000000000000000000, 1.000000000000000000, 1.000000000000000000, 1.000000000000000000, 1.000000000000000000, 1.000000000000000000, 1.000000000000000000, 1.000000000000000000, 1.000000000000000000, 1.000000000000000000, 1.000000000000000000, 1.000000000000000000, 1.000000000000000000, 1.000000000000000000, 1.000000000000000000),
 ( 0.7071067811865474617, 0.7071067811865474617, 0.7071067811865474617, 0.7071067811865474617, 0.7071067811865473507, 0.7071067811865473507, 0.7071067811865474617, 0.7071067811865474617, 0.7071067811865474617, 0.7071067811865474617, 0.7071067811865475727, 0.7071067811865475727, 0.7071067811865474617, 0.7071067811865474617, 0.7071067811865474617, 0.7071067811865474617, 0.7071067811865474617, 0.7071067811865474617),
 ( 1.000000000000000000, 1.000000000000000000, 1.000000000000000000, 1.000000000000000000, 1.000000000000000000, 1.000000000000000000, 1.000000000000000000, 1.000000000000000000, 1.000000000000000000, 1.000000000000000000, 1.000000000000000000, 1.000000000000000000, 1.000000000000000000, 1.000000000000000000, 1.000000000000000000, 1.000000000000000000, 1.000000000000000000, 1.000000000000000000) ) ) 
 REPRESENTATION_ITEM ( '' )  SURFACE ( )  );
#29647=CARTESIAN_POINT ( 'NONE',  ( 1.485997264023448450, 36.23016441347868977, 18.42518152272108622 ) ) ;
#29660=CARTESIAN_POINT ( 'NONE',  ( -12.28720923544494070, -14.55658080566520418, 20.99999999999999289 ) ) ;
#29668=CARTESIAN_POINT ( 'NONE',  ( -32.43957513060942688, -23.09559191376246901, 13.92931973827798231 ) ) ;
#29684=CARTESIAN_POINT ( 'NONE',  ( -17.67639428338700114, -29.21024101586626998, 10.99999999999985434 ) ) ;
#29691=CARTESIAN_POINT ( 'NONE',  ( 36.01097648505593440, -14.57711145883802395, 15.13084544680213384 ) ) ;
#29693=CARTESIAN_POINT ( 'NONE',  ( -10.55929393611012124, 36.39458846701819539, 13.92931973827808712 ) ) ;
#29695=CARTESIAN_POINT ( 'NONE',  ( -10.81727955708315925, -23.19337658762207965, 18.42518152272366549 ) ) ;
#29698=CARTESIAN_POINT ( 'NONE',  ( -0.8051564177164421965, 29.93655406406123376, 20.82122704794079837 ) ) ;
#29706=CARTESIAN_POINT ( 'NONE',  ( 5.578133564215900009, 24.05045924978373861, 20.99999999999999645 ) ) ;
#29708=CARTESIAN_POINT ( 'NONE',  ( -9.340438144419710653, 38.00965938231844632, 10.99999999999994138 ) ) ;
#29718=CARTESIAN_POINT ( 'NONE',  ( -28.25018339770791087, -2.647087534802860187, 19.27171037444157164 ) ) ;
#29733=LINE ( 'NONE', #23836, #7960 ) ;
#29738=CARTESIAN_POINT ( 'NONE',  ( -35.72300736400992349, -23.12593624637962719, 22.99999999999905498 ) ) ;
#29742=CARTESIAN_POINT ( 'NONE',  ( 21.70013981686734894, -23.40282575515950825, 19.27171037444156809 ) ) ;
#29743=EDGE_LOOP ( 'NONE', ( #8757, #929, #22249, #11897 ) ) ;
#29768=CARTESIAN_POINT ( 'NONE',  ( -23.05386822411328041, -7.747535282638268406, 20.99999999999999645 ) ) ;
#29779=CARTESIAN_POINT ( 'NONE',  ( -22.73078996736959922, -29.06185046644121428, 10.99999999999970868 ) ) ;
#29790=VECTOR ( 'NONE', #27251, 1000.000000000000000 ) ;
#29793=CARTESIAN_POINT ( 'NONE',  ( -10.32110568927837413, 19.34973993761487066, 20.50957957746001981 ) ) ;
#29794=CARTESIAN_POINT ( 'NONE',  ( 24.85114452701355958, -15.17411596029600851, 20.94377226548378346 ) ) ;
#29809=FACE_OUTER_BOUND ( 'NONE', #39873, .T. ) ;
#29847=B_SPLINE_CURVE_WITH_KNOTS ( 'NONE', 3,
 ( #6202, #4504, #854, #10601, #34240, #6930, #37085, #34043, #1260, #3895, #37283, #4299, #13234, #32137, #9255, #22579, #21837, #28882 ),
 .UNSPECIFIED., .F., .F.,
 ( 4, 2, 2, 2, 2, 2, 2, 2, 4 ),
 ( 0.000000000000000000, 0.08767908505624519289, 0.1753581701124903858, 0.2630372551687354954, 0.3507163402249806605, 0.4383954252812256591, 0.5260745103374705467, 0.6137535953937155453, 0.7014326804499604329 ),
 .UNSPECIFIED. ) ;
#29853=CARTESIAN_POINT ( 'NONE',  ( -4.817371740575545402, 23.83900317890010001, 23.00000000000000000 ) ) ;
#29860=CARTESIAN_POINT ( 'NONE',  ( 17.21213525677114120, -20.06193531423683041, 20.50957957746029336 ) ) ;
#29864=CARTESIAN_POINT ( 'NONE',  ( -36.30242391553720438, -14.63578948164528981, 14.53008259254010959 ) ) ;
#29882=CARTESIAN_POINT ( 'NONE',  ( -25.76746751309237737, -28.17378816281799558, 10.99999999999996625 ) ) ;
#29889=CARTESIAN_POINT ( 'NONE',  ( 35.82891851945763761, -9.175709056023070076, 15.72805884748939853 ) ) ;
#29890=VERTEX_POINT ( 'NONE', #40142 ) ;
#29891=CARTESIAN_POINT ( 'NONE',  ( -16.24129362380272212, 27.01431713449522221, 15.13084544680213561 ) ) ;
#29893=CARTESIAN_POINT ( 'NONE',  ( 16.23042486174298560, -23.86708630543422416, 18.87996532025784546 ) ) ;
#29895=CARTESIAN_POINT ( 'NONE',  ( 8.504221777570171170, 25.88639746736838987, 20.50957957746123128 ) ) ;
#29899=CARTESIAN_POINT ( 'NONE',  ( -39.48557158514991272, -11.24999999999982414, 23.00000000000000000 ) ) ;
#29906=CARTESIAN_POINT ( 'NONE',  ( 19.05502067200783500, 4.384649331628448721, 20.25080042701557304 ) ) ;
#29916=CARTESIAN_POINT ( 'NONE',  ( -24.52800942765094305, -23.26501842005211884, 18.87996532025785257 ) ) ;
#29930=CARTESIAN_POINT ( 'NONE',  ( 22.38472516250426381, -15.35952186208530357, 23.00000000000000000 ) ) ;
#29939=CARTESIAN_POINT ( 'NONE',  ( 30.92601969764218950, -9.797982979853070873, 19.66345542862528006 ) ) ;
#29955=CARTESIAN_POINT ( 'NONE',  ( 14.48927117870123027, -30.61587158504688233, 23.00000000000000000 ) ) ;
#29960=CARTESIAN_POINT ( 'NONE',  ( -10.24066009500599250, -26.58087177409006330, 14.53008259255018153 ) ) ;
#29964=CARTESIAN_POINT ( 'NONE',  ( -25.52323811238533224, -15.66556294379314451, 20.82122704794065271 ) ) ;
#29974=CARTESIAN_POINT ( 'NONE',  ( -31.38526299860026825, -24.75545609243354406, 11.55979286843934872 ) ) ;
#29985=CARTESIAN_POINT ( 'NONE',  ( 8.842822184360947801, 12.23747979796203289, 22.99999999999999289 ) ) ;
#29993=CARTESIAN_POINT ( 'NONE',  ( 20.02374874442605091, -18.66705478562347764, 20.82122704794080192 ) ) ;
#30012=CARTESIAN_POINT ( 'NONE',  ( 9.762440214476880485, -29.39637225273894572, 22.99999999999999645 ) ) ;
#30025=CARTESIAN_POINT ( 'NONE',  ( 39.51968006260096189, -13.07391885151743338, 11.00000000000000000 ) ) ;
#30038=CARTESIAN_POINT ( 'NONE',  ( -27.91036560783436471, 4.231346453976238209, 15.13084544680909005 ) ) ;
#30056=( NAMED_UNIT ( * ) SI_UNIT ( $, .STERADIAN. ) SOLID_ANGLE_UNIT ( ) );
#30068=B_SPLINE_CURVE_WITH_KNOTS ( 'NONE', 3,
 ( #14588, #2600, #12136, #39761, #15183, #5442, #30025, #21280, #8891, #17653, #33691, #8693, #14986, #8287, #5241, #2201, #24126, #24524 ),
 .UNSPECIFIED., .F., .F.,
 ( 4, 2, 2, 2, 2, 2, 2, 2, 4 ),
 ( 0.000000000000000000, 0.1250000000000000000, 0.2500000000000000000, 0.3750000000000000000, 0.5000000000000000000, 0.6250000000000000000, 0.7500000000000000000, 0.8750000000000000000, 1.000000000000000000 ),
 .UNSPECIFIED. ) ;
#30094=CARTESIAN_POINT ( 'NONE',  ( 16.92376161250197697, -28.83147800495239466, 13.32518128616474939 ) ) ;
#30096=CARTESIAN_POINT ( 'NONE',  ( -12.06278152636159007, 35.25200209733603174, 13.92931973827870706 ) ) ;
#30097=CARTESIAN_POINT ( 'NONE',  ( 12.01634099004108513, -16.14815750340189027, 20.94377226548372661 ) ) ;
#30098=CARTESIAN_POINT ( 'NONE',  ( 14.98890121934609532, -28.67928442654220333, 11.00000000000000000 ) ) ;
#30100=CARTESIAN_POINT ( 'NONE',  ( 6.949287954459814287, 25.26733242291902926, 20.82122704794137746 ) ) ;
#30111=CARTESIAN_POINT ( 'NONE',  ( 19.99288511728601136, -2.332377806213334015, 20.94377226548710524 ) ) ;
#30114=CARTESIAN_POINT ( 'NONE',  ( -1.947644445291298432, 40.50000000000004974, 11.00000000000000000 ) ) ;
#30122=CARTESIAN_POINT ( 'NONE',  ( -32.11924139737082129, -16.82817082614032955, 18.42518152272146637 ) ) ;
#30129=CARTESIAN_POINT ( 'NONE',  ( -19.26948696230206082, 27.85601271560033965, 23.00000000000000355 ) ) ;
#30136=CARTESIAN_POINT ( 'NONE',  ( 24.22138565352641493, -9.557272464391596500, 23.00000000000000000 ) ) ;
#30141=CARTESIAN_POINT ( 'NONE',  ( -38.66460482714639824, -17.32098561216439947, 22.99999999999999289 ) ) ;
#30143=ORIENTED_EDGE ( 'NONE', *, *, #36804, .F. ) ;
#30147=CARTESIAN_POINT ( 'NONE',  ( 31.26284659378134734, -14.97710070420450279, 19.27171037444157520 ) ) ;
#30168=CARTESIAN_POINT ( 'NONE',  ( -15.27443809245026785, -27.57253143578022048, 15.13084544680213561 ) ) ;
#30171=CARTESIAN_POINT ( 'NONE',  ( -26.96432039561874205, -11.11241571815037865, 20.82122704794107548 ) ) ;
#30199=CARTESIAN_POINT ( 'NONE',  ( 23.31304291943814277, -15.59395685184307290, 20.99999999999999645 ) ) ;
#30201=CARTESIAN_POINT ( 'NONE',  ( 14.98890121934608288, -28.67928442654220333, 11.00000000000000000 ) ) ;
#30210=CARTESIAN_POINT ( 'NONE',  ( 6.367390439426123372, 24.26983560722166544, 20.94377226548378701 ) ) ;
#30241=CARTESIAN_POINT ( 'NONE',  ( -17.01882136418544889, 27.23043334309702956, 13.32518128616608877 ) ) ;
#30260=( NAMED_UNIT ( * ) PLANE_ANGLE_UNIT ( ) SI_UNIT ( $, .RADIAN. ) );
#30298=CARTESIAN_POINT ( 'NONE',  ( 35.19094867589885212, -3.640833979052563674, 13.92931973827808534 ) ) ;
#30300=CARTESIAN_POINT ( 'NONE',  ( 16.03057579644872988, 28.88256098452291454, 14.53008259254079881 ) ) ;
#30301=CARTESIAN_POINT ( 'NONE',  ( -11.45923940081499559, -19.42154971137169639, 20.25080042701605976 ) ) ;
#30303=CARTESIAN_POINT ( 'NONE',  ( -8.504221777570748486, 25.88639746736783565, 20.50957957746009797 ) ) ;
#30314=CARTESIAN_POINT ( 'NONE',  ( 4.817371740575477013, 23.83900317890016751, 20.99999999999999645 ) ) ;
#30323=CARTESIAN_POINT ( 'NONE',  ( -24.79887074938341840, -23.91042127310561938, 18.42518152272108978 ) ) ;
#30338=CARTESIAN_POINT ( 'NONE',  ( 29.22254794994939786, -28.85350742528249413, 11.00000000000000000 ) ) ;
#30343=CARTESIAN_POINT ( 'NONE',  ( -35.72300736400902110, -23.12593624637910850, 11.00000000000000000 ) ) ;
#30351=CARTESIAN_POINT ( 'NONE',  ( 26.77946264071975691, -24.43926981373490648, 17.42190598798353207 ) ) ;
#30357=CARTESIAN_POINT ( 'NONE',  ( -15.07283634910000814, -28.35394831540519789, 13.32518128616608699 ) ) ;
#30368=CARTESIAN_POINT ( 'NONE',  ( -8.859192577249677569, 12.20922670551869516, 20.99999999999999645 ) ) ;
#30373=CARTESIAN_POINT ( 'NONE',  ( 10.13173764377233077, -27.22067640325132487, 12.73282698324872442 ) ) ;
#30377=CARTESIAN_POINT ( 'NONE',  ( -26.77583779507883932, -12.71777209950081655, 20.82122704794079837 ) ) ;
#30395=CARTESIAN_POINT ( 'NONE',  ( -75.15099915297791711, 43.38844959084113384, 23.00000000000000000 ) ) ;
#30405=CARTESIAN_POINT ( 'NONE',  ( 28.38958307348582366, -9.126824876479627591, 20.50957957746028626 ) ) ;
#30406=EDGE_CURVE ( 'NONE', #30744, #29890, #17770, .T. ) ;
#30409=CARTESIAN_POINT ( 'NONE',  ( 37.13148535761800417, -14.80270701502663044, 11.00000000000000000 ) ) ;
#30433=CARTESIAN_POINT ( 'NONE',  ( 32.28722999652337933, 1.315479119629256788, 12.14047268033097460 ) ) ;
#30447=CARTESIAN_POINT ( 'NONE',  ( -23.13582672293654596, 13.35747578641134048, 12.14047268033097282 ) ) ;
#30502=CARTESIAN_POINT ( 'NONE',  ( 22.69490999519655006, -28.86496244640809650, 12.73282698324817552 ) ) ;
#30504=CARTESIAN_POINT ( 'NONE',  ( -15.75274587708708474, 28.77197995862396240, 15.13084544680146770 ) ) ;
#30505=CARTESIAN_POINT ( 'NONE',  ( 4.283810552457587037E-14, -19.51153516500234630, 19.99202127657103389 ) ) ;
#30507=CARTESIAN_POINT ( 'NONE',  ( -1.161969254298623522, 33.23463598332011770, 19.99202127657103034 ) ) ;
#30518=CARTESIAN_POINT ( 'NONE',  ( 26.56332897235149559, -4.302820985781383278, 20.25080042701566541 ) ) ;
#30528=CARTESIAN_POINT ( 'NONE',  ( -29.15792305772344761, -20.09428552990363670, 18.87996532025785257 ) ) ;
#30539=ORIENTED_EDGE ( 'NONE', *, *, #11114, .F. ) ;
#30542=CARTESIAN_POINT ( 'NONE',  ( 38.42882785865609918, -4.479089857565665689, 22.99999999999905853 ) ) ;
#30553=CARTESIAN_POINT ( 'NONE',  ( 32.94564365859739752, -13.95995841273500915, 18.42518152272108978 ) ) ;
#30573=CARTESIAN_POINT ( 'NONE',  ( 10.24066009500897856, -26.58087177406422796, 14.53008259253875067 ) ) ;
#30576=CARTESIAN_POINT ( 'NONE',  ( -25.38348611796456922, -5.460896781496030528, 20.69868183039781684 ) ) ;
#30602=CARTESIAN_POINT ( 'NONE',  ( 17.21213525677114120, -20.06193531423682685, 20.50957957746029692 ) ) ;
#30630=CARTESIAN_POINT ( 'NONE',  ( 32.33143948541787438, 1.358872982501792226, 11.00000000000000000 ) ) ;
#30635=CARTESIAN_POINT ( 'NONE',  ( -33.02831943717539787, -0.5583946152437758714, 14.53008259253993728 ) ) ;
#30642=ORIENTED_EDGE ( 'NONE', *, *, #29059, .F. ) ;
#30644=CARTESIAN_POINT ( 'NONE',  ( -17.34253826607185545, 27.32041144404030675, 11.00000000000000000 ) ) ;
#30696=ORIENTED_EDGE ( 'NONE', *, *, #20027, .F. ) ;
#30699=CARTESIAN_POINT ( 'NONE',  ( 10.77072277543604351, 36.67279993932673676, 12.73282698324853435 ) ) ;
#30700=CARTESIAN_POINT ( 'NONE',  ( 4.287285461719674021E-14, -18.69445663741131014, 20.25080042701566541 ) ) ;
#30702=CARTESIAN_POINT ( 'NONE',  ( -7.420252307062940034, 30.34362403113889073, 19.99202127657163075 ) ) ;
#30724=CARTESIAN_POINT ( 'NONE',  ( -30.82027224585467096, -2.301877357439013227, 17.92354375535249389 ) ) ;
#30744=VERTEX_POINT ( 'NONE', #26598 ) ;
#30745=EDGE_CURVE ( 'NONE', #38528, #18297, #9710, .T. ) ;
#30749=CARTESIAN_POINT ( 'NONE',  ( 32.91936639158326017, -8.047070124325959029, 18.42518152272108622 ) ) ;
#30750=ORIENTED_EDGE ( 'NONE', *, *, #4509, .T. ) ;
#30756=CARTESIAN_POINT ( 'NONE',  ( -39.48557158514991272, -11.24999999999982414, 3.000000000000000000 ) ) ;
#30761=CARTESIAN_POINT ( 'NONE',  ( 23.01716326618264574, 13.28896540771174628, 12.73282698324853257 ) ) ;
#30772=CARTESIAN_POINT ( 'NONE',  ( -25.82695741053184335, -7.282955883995192892, 20.82122704794065982 ) ) ;
#30792=ORIENTED_EDGE ( 'NONE', *, *, #2330, .T. ) ;
#30798=CARTESIAN_POINT ( 'NONE',  ( 26.93475362026859088, -11.92845428170237909, 20.82122704794080548 ) ) ;
#30829=CARTESIAN_POINT ( 'NONE',  ( -37.03605016781039438, -10.92602907108566868, 13.92931973827882253 ) ) ;
#30839=CARTESIAN_POINT ( 'NONE',  ( -22.45707936798516968, 12.96560081831745670, 14.53008259254011136 ) ) ;
#30843=CARTESIAN_POINT ( 'NONE',  ( 21.92391373441417102, -15.64922772886939661, 23.00000000000000711 ) ) ;
#30854=CARTESIAN_POINT ( 'NONE',  ( 33.75875814100320582, 2.759858869446452978, 11.00000000000000000 ) ) ;
#30896=CARTESIAN_POINT ( 'NONE',  ( -9.166052203149666511, 37.72018303275904572, 13.32518128616555586 ) ) ;
#30898=CARTESIAN_POINT ( 'NONE',  ( 5.938964939929074482, -16.21345324574345170, 20.82122704794080192 ) ) ;
#30900=CARTESIAN_POINT ( 'NONE',  ( 8.207473342610013489, 28.06734471880750093, 20.25080042701566896 ) ) ;
#30920=CARTESIAN_POINT ( 'NONE',  ( -29.39157470508739323, -22.49273609621608827, 17.42190598798392998 ) ) ;
#30924=ORIENTED_EDGE ( 'NONE', *, *, #15295, .T. ) ;
#30927=( BOUNDED_CURVE ( )  B_SPLINE_CURVE ( 2, ( #26311, #36062, #8627 ),
 .UNSPECIFIED., .F., .F. ) 
 B_SPLINE_CURVE_WITH_KNOTS ( ( 3, 3 ),
 ( 0.000000000000000000, 1.000000000000000000 ),
 .UNSPECIFIED. ) 
 CURVE ( )  GEOMETRIC_REPRESENTATION_ITEM ( )  RATIONAL_B_SPLINE_CURVE ( ( 1.000000000000000000, 0.7071067811865474617, 1.000000000000000000 ) ) 
 REPRESENTATION_ITEM ( '' )  );
#30944=CARTESIAN_POINT ( 'NONE',  ( 30.14286744058976453, -20.99504498967356270, 17.92354375535288824 ) ) ;
#30952=CARTESIAN_POINT ( 'NONE',  ( 19.89620541518914010, 17.40116461633694911, 14.53008259253988044 ) ) ;
#30963=CARTESIAN_POINT ( 'NONE',  ( -28.07442828530314216, -16.20877872786413576, 20.25080042701565830 ) ) ;
#30991=CARTESIAN_POINT ( 'NONE',  ( 24.79273775960278314, -6.040746354376016924, 20.82122704794079837 ) ) ;
#31000=FACE_OUTER_BOUND ( 'NONE', #20293, .T. ) ;
#31027=CARTESIAN_POINT ( 'NONE',  ( -33.17211272335762118, -21.25822893968250327, 15.13084544680185850 ) ) ;
#31038=B_SPLINE_CURVE_WITH_KNOTS ( 'NONE', 3,
 ( #1660, #11007, #29684, #36187, #32945, #5103, #29882, #14440, #23392, #35787, #7941, #26835, #8354, #39226, #11405, #23788, #27039, #28232 ),
 .UNSPECIFIED., .F., .F.,
 ( 4, 2, 2, 2, 2, 2, 2, 2, 4 ),
 ( 0.000000000000000000, 0.08767823854539483208, 0.1753564770907896642, 0.2630347156361845240, 0.3507129541815793283, 0.4383911927269741327, 0.5260694312723690480, 0.6137476698177638523, 0.7014259083631586567 ),
 .UNSPECIFIED. ) ;
#31042=CARTESIAN_POINT ( 'NONE',  ( -18.85374159600211641, 16.91074157332653982, 16.30093088680128233 ) ) ;
#31053=CARTESIAN_POINT ( 'NONE',  ( 30.33922525716342733, 6.243664897651060919, 23.00000000003197798 ) ) ;
#31097=CARTESIAN_POINT ( 'NONE',  ( 12.20958131808574798, 35.40723086407815856, 13.32518128616605324 ) ) ;
#31101=CARTESIAN_POINT ( 'NONE',  ( -6.000734348601507229, 30.39614672895594438, 20.25080042701566541 ) ) ;
#31117=CARTESIAN_POINT ( 'NONE',  ( -15.74227866054087066, -25.75916161678338412, 17.42190598798392642 ) ) ;
#31122=ORIENTED_EDGE ( 'NONE', *, *, #13984, .T. ) ;
#31130=CARTESIAN_POINT ( 'NONE',  ( 35.27625572565171552, 1.213838575767202776, 11.00000000000000000 ) ) ;
#31141=CARTESIAN_POINT ( 'NONE',  ( 21.91981567634946870, -15.65087685632042103, 20.99999999999999289 ) ) ;
#31142=CARTESIAN_POINT ( 'NONE',  ( 23.60877407455211596, -25.08990816561031778, 17.92354375535291666 ) ) ;
#31153=CARTESIAN_POINT ( 'NONE',  ( 16.81416712650777256, 27.17354907311674950, 13.92931973827808712 ) ) ;
#31159=EDGE_CURVE ( 'NONE', #27076, #4088, #6259, .T. ) ;
#31163=CARTESIAN_POINT ( 'NONE',  ( -22.09885373566634925, -20.02268770624659311, 20.50957957746052074 ) ) ;
#31187=CARTESIAN_POINT ( 'NONE',  ( 26.87422832650572602, -16.65342898056121257, 20.50957957746029336 ) ) ;
#31195=DIRECTION ( 'NONE',  ( 0.000000000000000000, 0.000000000000000000, 1.000000000000000000 ) ) ;
#31214=VECTOR ( 'NONE', #9612, 1000.000000000000000 ) ;
#31222=CARTESIAN_POINT ( 'NONE',  ( -35.62872793493689727, -3.428732413881794727, 12.14047268033097460 ) ) ;
#31232=CARTESIAN_POINT ( 'NONE',  ( -17.25967040862722612, 21.92197836111047593, 15.72805884749868532 ) ) ;
#31241=CARTESIAN_POINT ( 'NONE',  ( 20.76390118686654418, -28.86769433464313650, 13.32518128616608344 ) ) ;
#31294=CARTESIAN_POINT ( 'NONE',  ( -3.857345576530716968, 39.98449713665793581, 12.73282698324867823 ) ) ;
#31297=CARTESIAN_POINT ( 'NONE',  ( -3.920592112299368104, 34.13862021880815689, 19.27171037444158230 ) ) ;
#31312=CARTESIAN_POINT ( 'NONE',  ( -35.11176058605715156, -10.96173827525908706, 16.87380292611522847 ) ) ;
#31334=CARTESIAN_POINT ( 'NONE',  ( 35.51887168742078416, -12.71114019210517121, 16.30093088680192537 ) ) ;
#31340=CARTESIAN_POINT ( 'NONE',  ( -2.109751222703438955, 28.76298082888541785, 20.94377226548378346 ) ) ;
#31356=CARTESIAN_POINT ( 'NONE',  ( -29.41993030479137516, -12.15499915640478257, 20.25080042701567962 ) ) ;
#31384=CARTESIAN_POINT ( 'NONE',  ( 28.84864528223400271, -18.09713003384586827, 19.66345542862528362 ) ) ;
#31399=DIRECTION ( 'NONE',  ( -0.000000000000000000, -0.000000000000000000, -1.000000000000000000 ) ) ;
#31402=( NAMED_UNIT ( * ) SI_UNIT ( $, .STERADIAN. ) SOLID_ANGLE_UNIT ( ) );
#31416=B_SPLINE_SURFACE_WITH_KNOTS ( 'NONE', 3, 3, ( 
 ( #37242, #9414, #268, #12655, #25045, #37439, #21204, #33610, #6547, #5761, #32147, #15906, #22791, #22189, #26040, #1067, #3509, #7347, #12851, #864, #3705, #19545, #6741, #469, #29096 ),
 ( #25840, #4310, #38442, #16105, #16712, #28893, #28689, #28487, #22590, #25242, #34589, #663, #10612, #37642, #31742, #7149, #13043, #19148, #3905, #25432, #13245, #31541, #13448, #38034, #37832 ),
 ( #31936, #10004, #4104, #19752, #1269, #22994, #7555, #28291, #9809, #10410, #13653, #35189, #22384, #34790, #35397, #31340, #6942, #38240, #19347, #16302, #25635, #10206, #34997, #16508, #1672 ),
 ( #20768, #30100, #36003, #35601, #13857, #2274, #14256, #23800, #32759, #4515, #8159, #7756, #33163, #29698, #36205, #17322, #20161, #32354, #26446, #26648, #11020, #39437, #4717, #5117, #19959 ),
 ( #27053, #38641, #39036, #11215, #10815, #17121, #23202, #24000, #1880, #32558, #29499, #14053, #20566, #32961, #17523, #2077, #23605, #5313, #16917, #38843, #11418, #26245, #36399, #23404, #35799 ),
 ( #1469, #29895, #7954, #14452, #20367, #29299, #17724, #26849, #39238, #8367, #14661, #4917, #11619, #12009, #8561, #28044, #24399, #5506, #15257, #18710, #11812, #36791, #33763, #30303, #24999 ),
 ( #14862, #18511, #27645, #30900, #21547, #27249, #5909, #40027, #36995, #21153, #9164, #24796, #34151, #3264, #20956, #33364, #17920, #27847, #31101, #20, #8765, #36594, #12405, #15658, #24197 ),
 ( #221, #12607, #21744, #5710, #8968, #2476, #39636, #21356, #18312, #6301, #15055, #18120, #33561, #30507, #37193, #24602, #27445, #2670, #39832, #30702, #2868, #12208, #33948, #9367, #6105 ),
 ( #3062, #15456, #28442, #16662, #22144, #814, #10361, #13602, #619, #16458, #22536, #7297, #28843, #19703, #25793, #19497, #34947, #3861, #1021, #28246, #32095, #7101, #9566, #13401, #18904 ),
 ( #423, #34544, #31892, #19103, #38190, #16053, #4055, #22740, #4261, #9764, #35144, #29044, #34745, #6695, #28644, #31297, #12802, #31496, #1224, #6499, #21948, #6895, #37391, #34350, #37787 ),
 ( #16259, #3463, #10163, #15858, #19295, #13195, #25589, #3660, #37990, #25199, #37598, #13000, #25388, #9959, #22339, #31694, #26600, #32710, #16869, #4466, #4862, #38992, #29249, #7908, #7504 ),
 ( #1420, #23149, #22946, #35952, #7711, #35547, #1829, #38590, #13803, #11166, #26195, #29647, #26396, #10764, #19907, #8107, #20113, #32301, #10563, #23557, #17276, #32512, #35348, #14209, #4666 ),
 ( #25990, #17068, #38792, #38389, #29446, #1625, #14007, #10971, #23358, #35753, #20313, #10494, #4193, #7232, #28777, #19632, #22080, #953, #22875, #19431, #7031, #12935, #37725, #22271, #28978 ),
 ( #3990, #34676, #9892, #19230, #38118, #22675, #35078, #16597, #25725, #35279, #6628, #6829, #13536, #1353, #31623, #10291, #7435, #38523, #13128, #1154, #32028, #32233, #25924, #4395, #19844 ),
 ( #16801, #28576, #38324, #26127, #29186, #13738, #551, #13332, #34481, #25326, #3790, #16192, #19036, #16391, #750, #25520, #37921, #31428, #3595, #15992, #28371, #10093, #22473, #34878, #31824 ),
 ( #35187, #34787, #32143, #26441, #19955, #19543, #19750, #13242, #34994, #32351, #31933, #29296, #28889, #4511, #10812, #17118, #22588, #23198, #7552, #7344, #7143, #1266, #31737, #862, #4102 ),
 ( #4306, #32555, #13650, #16506, #20156, #16299, #16913, #29092, #1466, #22990, #28686, #16708, #26037, #38436, #1064, #10609, #26242, #35597, #4714, #10002, #22381, #6939, #13851, #29493, #38637 ),
 ( #3902, #7753, #10204, #13445, #35394, #1669, #14049, #19345, #25838, #38238, #25632, #38031, #10408, #22785, #11808, #5113, #36000, #5706, #8156, #27244, #14658, #17520, #17319, #30504, #29891 ),
 ( #33557, #30300, #20560, #7951, #24194, #14449, #2472, #39033, #23797, #23400, #20764, #15051, #8558, #32957, #8364, #1877, #23602, #20953, #2073, #17916, #26845, #33360, #39632, #18117, #11211 ),
 ( #38840, #2664, #39235, #35795, #5310, #8761, #14253, #11415, #36198, #21150, #2270, #33158, #11016, #4911, #5503, #17720, #14859, #11614, #29693, #30096, #27049, #39433, #23997, #36394, #36591 ),
 ( #20363, #32756, #26644, #419, #33944, #31097, #6102, #15855, #8962, #3459, #27642, #18507, #3261, #19099, #31493, #12799, #24598, #30896, #21353, #3657, #27844, #3059, #25194, #15451, #36991 ),
 ( #28243, #15653, #17, #5905, #27441, #12400, #30699, #24395, #22141, #18900, #9160, #36788, #37594, #24793, #31294, #37190, #24995, #9363, #33760, #15253, #21741, #9761, #21544, #37388, #34147 ),
 ( #34541, #9562, #12604, #6297, #21943, #39829, #18706, #6692, #28040, #217, #18308, #2864, #40023, #34347, #6495, #12006, #12204, #4051, #10159, #16455, #811, #10358, #25385, #16049, #10760 ),
 ( #31689, #7501, #25789, #19292, #13192, #25987, #37987, #35343, #34943, #10559, #16865, #23145, #28640, #29246, #13599, #13398, #25586, #7293, #37784, #6892, #22533, #35543, #9956, #28438, #38186 ),
 ( #26192, #22336, #38385, #35141, #22942, #29041, #34741, #22735, #19698, #4258, #7095, #16659, #32298, #1417, #7707, #32507, #615, #12996, #19904, #38585, #4462, #16255, #3858, #13799, #20109 ) ),
 .UNSPECIFIED., .F., .F., .F.,
 ( 4, 3, 3, 3, 3, 3, 3, 3, 4 ),
 ( 4, 3, 3, 3, 3, 3, 3, 3, 4 ),
 ( 0.000000000000000000, 0.1250000000000000000, 0.2500000000000000000, 0.3750000000000000000, 0.5000000000000000000, 0.6250000000000000000, 0.7500000000000000000, 0.8750000000000000000, 1.000000000000000000 ),
 ( 0.2711095619351722164, 0.5960312531501053002, 0.9209529443650383840, 1.245874635579971468, 1.570796326794904552, 1.895718018009837635, 2.220639709224770719, 2.545561400439703803, 2.870483091654636887 ),
 .UNSPECIFIED. ) ;
#31420=CARTESIAN_POINT ( 'NONE',  ( -37.17935095643291987, -12.86265498539201957, 13.32518128616588626 ) ) ;
#31427=CARTESIAN_POINT ( 'NONE',  ( 12.25538945203533459, -14.54837145661906384, 23.00000000000000355 ) ) ;
#31428=CARTESIAN_POINT ( 'NONE',  ( -8.062736477019040393, 35.88854577675052582, 16.87380292611359422 ) ) ;
#31432=CARTESIAN_POINT ( 'NONE',  ( -14.43694901005832243, 26.51279404185573796, 17.42190598798392998 ) ) ;
#31439=CARTESIAN_POINT ( 'NONE',  ( 31.02271782694946722, -24.34398845624577135, 13.92931973827809067 ) ) ;
#31440=ORIENTED_EDGE ( 'NONE', *, *, #16309, .F. ) ;
#31445=CARTESIAN_POINT ( 'NONE',  ( 19.26948696230200397, 27.85601271560037162, 22.99999999999999645 ) ) ;
#31459=CARTESIAN_POINT ( 'NONE',  ( -19.26948696230206437, 27.85601271560034320, 11.00000000000000000 ) ) ;
#31493=CARTESIAN_POINT ( 'NONE',  ( -3.827636526755954449, 39.84991882288245080, 13.32518128616621844 ) ) ;
#31495=CARTESIAN_POINT ( 'NONE',  ( -6.471455985784314358, 17.88805487301255681, 23.00000000000000000 ) ) ;
#31496=CARTESIAN_POINT ( 'NONE',  ( -6.372562348374944285, 33.08234073370745421, 19.27171037444085755 ) ) ;
#31508=CARTESIAN_POINT ( 'NONE',  ( 15.00437666251104396, -28.61930095463400292, 12.14047268033097637 ) ) ;
#31516=CARTESIAN_POINT ( 'NONE',  ( -30.17922767059458167, -0.7536324250905129807, 17.42190598798392998 ) ) ;
#31535=CARTESIAN_POINT ( 'NONE',  ( 24.22138565352629058, -9.557272464391640909, 21.00000000000001066 ) ) ;
#31536=CARTESIAN_POINT ( 'NONE',  ( 33.67755813373108964, -6.176019118478268233, 17.42190598798353562 ) ) ;
#31540=CARTESIAN_POINT ( 'NONE',  ( -17.34253826607186966, 27.32041144404028188, 23.00000000000000000 ) ) ;
#31541=CARTESIAN_POINT ( 'NONE',  ( -4.791301586986582706, 25.75006569903015574, 20.99999999999999645 ) ) ;
#31546=CARTESIAN_POINT ( 'NONE',  ( 18.63686013480785775, 22.43247111562878615, 12.14047268031015214 ) ) ;
#31549=LINE ( 'NONE', #18964, #154 ) ;
#31553=CARTESIAN_POINT ( 'NONE',  ( -21.27406655599722995, -21.06385835267891693, 20.25080042701542382 ) ) ;
#31578=CARTESIAN_POINT ( 'NONE',  ( 27.96047413129323189, -4.559793092418160221, 19.99202127657250116 ) ) ;
#31602=CARTESIAN_POINT ( 'NONE',  ( 36.04785107591597892, -18.56329043283713887, 11.00000000000005684 ) ) ;
#31613=CARTESIAN_POINT ( 'NONE',  ( -28.15028875894780924, -26.91874057851014612, 12.73282698324841711 ) ) ;
#31623=CARTESIAN_POINT ( 'NONE',  ( -3.246717519899657400, 37.21789761807042396, 17.42190598798395484 ) ) ;
#31628=CARTESIAN_POINT ( 'NONE',  ( -15.47112132963103726, 15.31948306975548491, 19.27171037444150770 ) ) ;
#31635=CARTESIAN_POINT ( 'NONE',  ( 15.00437666251104218, -28.61930095463399581, 12.14047268033097460 ) ) ;
#31660=CARTESIAN_POINT ( 'NONE',  ( -18.68934290553424304, 29.94321432092579727, 11.00000000000000000 ) ) ;
#31679=CARTESIAN_POINT ( 'NONE',  ( -27.71565130972192392, -3.171757977838550513, 19.66345542862528717 ) ) ;
#31689=CARTESIAN_POINT ( 'NONE',  ( 17.34253826607195847, 27.32041144403996213, 11.55979286843935050 ) ) ;
#31694=CARTESIAN_POINT ( 'NONE',  ( -4.159699369156335536, 34.84843100105939584, 18.87996532025786323 ) ) ;
#31697=VERTEX_POINT ( 'NONE', #12308 ) ;
#31705=CARTESIAN_POINT ( 'NONE',  ( 4.672335726383267662, 24.36080358023194137, 21.00000000000000000 ) ) ;
#31707=ADVANCED_FACE ( 'NONE', ( #31000 ), #28143, .F. ) ;
#31712=CARTESIAN_POINT ( 'NONE',  ( -34.38615473478483153, -15.96524117250080010, 16.87380292611443622 ) ) ;
#31735=CARTESIAN_POINT ( 'NONE',  ( 29.75773323547294424, -22.90830468393526687, 16.87380292611442556 ) ) ;
#31737=CARTESIAN_POINT ( 'NONE',  ( -14.21869892593723428, 30.05184351263790532, 16.30093088680186497 ) ) ;
#31742=CARTESIAN_POINT ( 'NONE',  ( -1.254079983865611370, 28.18681535329822196, 20.99999999999999645 ) ) ;
#31750=CARTESIAN_POINT ( 'NONE',  ( 16.24129362379723673, 27.01431713451477279, 15.13084544680213739 ) ) ;
#31758=CARTESIAN_POINT ( 'NONE',  ( -25.62037635619380893, -16.85925998830651906, 20.69868183039781684 ) ) ;
#31784=CARTESIAN_POINT ( 'NONE',  ( 20.32014898129569147, -22.75198622026958617, 19.66345542862527651 ) ) ;
#31790=LINE ( 'NONE', #29899, #21057 ) ;
#31816=CARTESIAN_POINT ( 'NONE',  ( -29.72906145568333258, -25.76693493179011085, 13.32518128616621667 ) ) ;
#31824=CARTESIAN_POINT ( 'NONE',  ( -14.97058623676950262, 26.66112013780927015, 16.87380292611441490 ) ) ;
#31827=CARTESIAN_POINT ( 'NONE',  ( -24.37528612864471711, 1.300641855047817153, 19.27171037444580648 ) ) ;
#31830=CARTESIAN_POINT ( 'NONE',  ( 20.38753357181594694, -16.19769905861743098, 20.99999999999999645 ) ) ;
#31834=CARTESIAN_POINT ( 'NONE',  ( 26.42723928173402470, -27.79046472072450413, 12.14047268033097104 ) ) ;
#31857=CARTESIAN_POINT ( 'NONE',  ( -4.331888854854360815, 42.14502281367542480, 11.00000000000000000 ) ) ;
#31862=CARTESIAN_POINT ( 'NONE',  ( -24.51458563001630964, -11.16205237993636956, 23.00000000000000711 ) ) ;
#31892=CARTESIAN_POINT ( 'NONE',  ( 10.90977822005762832, 28.29415442298315142, 19.27171037444158586 ) ) ;
#31908=CARTESIAN_POINT ( 'NONE',  ( -25.49851591039071863, -25.57752154475369366, 16.87380292611442201 ) ) ;
#31924=ORIENTED_EDGE ( 'NONE', *, *, #22163, .F. ) ;
#31931=CARTESIAN_POINT ( 'NONE',  ( 34.14640338304414513, -7.754617911606312752, 17.42190598798393353 ) ) ;
#31933=CARTESIAN_POINT ( 'NONE',  ( 3.468257360957521573, 38.22173125672342309, 16.30093088680195024 ) ) ;
#31936=CARTESIAN_POINT ( 'NONE',  ( 6.367390439426121596, 24.26983560722165834, 20.94377226548378346 ) ) ;
#31944=CARTESIAN_POINT ( 'NONE',  ( 24.77298340259215692, 8.359746025956967586, 15.13084544680224575 ) ) ;
#31952=CARTESIAN_POINT ( 'NONE',  ( -31.83642866623216605, -11.02236948596316424, 19.27171037444223956 ) ) ;
#31953=DIRECTION ( 'NONE',  ( 0.000000000000000000, 0.000000000000000000, 1.000000000000000000 ) ) ;
#31958=EDGE_CURVE ( 'NONE', #34372, #4972, #31790, .T. ) ;
#31980=CARTESIAN_POINT ( 'NONE',  ( 28.04602290581444635, -19.07745245555366864, 19.66345542862561047 ) ) ;
#31991=EDGE_CURVE ( 'NONE', #7799, #1139, #15956, .T. ) ;
#31997=( GEOMETRIC_REPRESENTATION_CONTEXT ( 3 ) GLOBAL_UNCERTAINTY_ASSIGNED_CONTEXT ( ( #32340 ) ) GLOBAL_UNIT_ASSIGNED_CONTEXT ( ( #8111, #30260, #8720 ) ) REPRESENTATION_CONTEXT ( 'NONE', 'WORKASPACE' ) );
#32007=CARTESIAN_POINT ( 'NONE',  ( 36.74707368630883053, -16.71203845619566053, 10.99999999999983125 ) ) ;
#32018=CARTESIAN_POINT ( 'NONE',  ( -35.86478881511108341, -18.48242683698273225, 12.73282698324857698 ) ) ;
#32028=CARTESIAN_POINT ( 'NONE',  ( -11.49018961600678779, 32.25363044047580985, 17.42190598798392287 ) ) ;
#32031=CARTESIAN_POINT ( 'NONE',  ( -8.755436920523948174, 18.76929632780095858, 20.82122704794065982 ) ) ;
#32033=CARTESIAN_POINT ( 'NONE',  ( 19.48557158514982746, -11.25000000000009415, 23.00000000000000000 ) ) ;
#32036=CARTESIAN_POINT ( 'NONE',  ( 29.92393930195800067, -26.04303208588349250, 11.55979286843930964 ) ) ;
#32039=ORIENTED_EDGE ( 'NONE', *, *, #16721, .T. ) ;
#32058=CARTESIAN_POINT ( 'NONE',  ( -3.833852081710640292, 25.75497152300896175, 23.00000000000000000 ) ) ;
#32080=CARTESIAN_POINT ( 'NONE',  ( -25.98021325959403427, -4.875178728618521973, 20.50957957746029692 ) ) ;
#32092=CARTESIAN_POINT ( 'NONE',  ( 4.817371740575539185, 23.83900317890011422, 20.99999999999999645 ) ) ;
#32095=CARTESIAN_POINT ( 'NONE',  ( -8.842993596485667851, 30.00678625355870111, 19.66345542862525519 ) ) ;
#32097=CARTESIAN_POINT ( 'NONE',  ( 3.863783140547853712E-14, -86.77689918168233874, 3.000000000000000000 ) ) ;
#32109=CARTESIAN_POINT ( 'NONE',  ( 15.27443809245942141, -27.57253143578274290, 15.13084544680213561 ) ) ;
#32115=CARTESIAN_POINT ( 'NONE',  ( -33.53427059938940857, -2.462512058961074946, 15.72805884748892957 ) ) ;
#32137=CARTESIAN_POINT ( 'NONE',  ( -38.11240863262091949, -18.68972660803411046, 11.00000000000000355 ) ) ;
#32141=CARTESIAN_POINT ( 'NONE',  ( 17.23228185427324277, -26.71557896777858332, 16.87380292611382515 ) ) ;
#32143=CARTESIAN_POINT ( 'NONE',  ( 14.21868324749889645, 30.05186662605645864, 16.30093088680188274 ) ) ;
#32144=CARTESIAN_POINT ( 'NONE',  ( -5.468510220371378239, -21.80712738496724157, 18.87996532025784902 ) ) ;
#32147=CARTESIAN_POINT ( 'NONE',  ( 1.082972213713589094, 27.41125570341916173, 21.00000000000000355 ) ) ;
#32156=CARTESIAN_POINT ( 'NONE',  ( 19.62624412895855741, 17.27415994119410669, 15.13084544680202548 ) ) ;
#32164=CARTESIAN_POINT ( 'NONE',  ( -30.76885290917900662, -8.559665202950077045, 19.66345542862464768 ) ) ;
#32175=DIRECTION ( 'NONE',  ( 1.000000000000000000, 0.000000000000000000, -0.000000000000000000 ) ) ;
#32184=CARTESIAN_POINT ( 'NONE',  ( -20.92112759555551094, -16.07000418475121961, 23.00000000000000000 ) ) ;
#32191=CARTESIAN_POINT ( 'NONE',  ( 26.04200899061357077, -18.69117426458517528, 20.25080042701566541 ) ) ;
#32224=CARTESIAN_POINT ( 'NONE',  ( -22.73078996736922264, -29.06185046644117165, 11.55979286843901122 ) ) ;
#32231=CARTESIAN_POINT ( 'NONE',  ( -8.437494178870162287, 40.76200630940459746, 11.00000000000000178 ) ) ;
#32233=CARTESIAN_POINT ( 'NONE',  ( -12.40052356344504680, 30.91160080447363256, 17.42190598798392642 ) ) ;
#32236=( BOUNDED_SURFACE ( )  B_SPLINE_SURFACE ( 2, 3, ( 
 ( #2387, #36509, #33278, #39944, #6018, #5827 ),
 ( #14777, #30012, #17837, #27164, #21462, #8877 ),
 ( #2188, #36713, #2979, #11529, #18423, #23914 ) ),
 .UNSPECIFIED., .F., .F., .T. ) 
 B_SPLINE_SURFACE_WITH_KNOTS ( ( 3, 3 ),
 ( 4, 2, 4 ),
 ( 0.000000000000000000, 1.000000000000000000 ),
 ( 1.318307113131750086, 1.570796326794896336, 1.823285540458042586 ),
 .UNSPECIFIED. ) 
 GEOMETRIC_REPRESENTATION_ITEM ( )  RATIONAL_B_SPLINE_SURFACE ( (
 ( 1.000000000000000000, 1.000000000000000000, 1.000000000000000000, 1.000000000000000000, 1.000000000000000000, 1.000000000000000000),
 ( 0.7071067811865474617, 0.7071067811865474617, 0.7071067811865474617, 0.7071067811865474617, 0.7071067811865474617, 0.7071067811865474617),
 ( 1.000000000000000000, 1.000000000000000000, 1.000000000000000000, 1.000000000000000000, 1.000000000000000000, 1.000000000000000000) ) ) 
 REPRESENTATION_ITEM ( '' )  SURFACE ( )  );
#32244=CARTESIAN_POINT ( 'NONE',  ( 37.13148535761801838, -14.80270701502657538, 11.55979286843934872 ) ) ;
#32298=CARTESIAN_POINT ( 'NONE',  ( -1.477035006930975258E-13, 40.50000000000004974, 11.00000000000000000 ) ) ;
#32301=CARTESIAN_POINT ( 'NONE',  ( -7.124477683922587623, 34.33078274760865867, 18.42518152272030463 ) ) ;
#32321=VERTEX_POINT ( 'NONE', #11375 ) ;
#32323=CARTESIAN_POINT ( 'NONE',  ( -34.64424588158978935, -17.94331620955210127, 15.72805884748971650 ) ) ;
#32340=UNCERTAINTY_MEASURE_WITH_UNIT (LENGTH_MEASURE( 1.000000000000000082E-05 ), #8111, 'distance_accuracy_value', 'NONE');
#32349=CARTESIAN_POINT ( 'NONE',  ( 20.70549897995575961, -28.06280627726307486, 15.13084544680213384 ) ) ;
#32351=CARTESIAN_POINT ( 'NONE',  ( 5.109761443618928922, 37.66877327392104036, 16.30093088680190760 ) ) ;
#32352=CARTESIAN_POINT ( 'NONE',  ( 10.71169154830999659, -23.81371503812557222, 17.92354375535058253 ) ) ;
#32354=CARTESIAN_POINT ( 'NONE',  ( -3.858525888478689936, 28.90799431746169290, 20.82122704794051415 ) ) ;
#32364=CARTESIAN_POINT ( 'NONE',  ( 16.15127118876671020, 15.63943246416513588, 18.87996532025803376 ) ) ;
#32374=CARTESIAN_POINT ( 'NONE',  ( -31.66906069137318624, -9.703676519219762042, 19.27171037444156099 ) ) ;
#32394=CARTESIAN_POINT ( 'NONE',  ( -38.42882785865835160, -4.479089857567120525, 23.00000000000094147 ) ) ;
#32401=CARTESIAN_POINT ( 'NONE',  ( 24.52800942765090753, -23.26501842005243148, 18.87996532025785967 ) ) ;
#32434=CARTESIAN_POINT ( 'NONE',  ( -32.33143948541789570, 1.358872982501977633, 11.55979286843934872 ) ) ;
#32446=CARTESIAN_POINT ( 'NONE',  ( -5.578133564216631868, 24.05045924978127303, 20.99999999999999645 ) ) ;
#32448=CARTESIAN_POINT ( 'NONE',  ( 24.37759566069541250, -10.08322588119073693, 20.99999999999999645 ) ) ;
#32452=CARTESIAN_POINT ( 'NONE',  ( 31.25372621196095935, -24.60616950719559526, 12.73282698324852724 ) ) ;
#32454=ORIENTED_EDGE ( 'NONE', *, *, #17127, .F. ) ;
#32507=CARTESIAN_POINT ( 'NONE',  ( -5.746222359017808756, 39.55816310746045872, 11.00000000000000355 ) ) ;
#32512=CARTESIAN_POINT ( 'NONE',  ( -11.36267260525735168, 30.20759924275325758, 18.42518152272108622 ) ) ;
#32532=CARTESIAN_POINT ( 'NONE',  ( -36.05338440271489731, -10.94427667939905824, 15.72805884749021033 ) ) ;
#32534=VECTOR ( 'NONE', #15857, 1000.000000000000000 ) ;
#32553=CARTESIAN_POINT ( 'NONE',  ( 25.86085639998011132, -26.44089909996149501, 15.72805884748939853 ) ) ;
#32555=CARTESIAN_POINT ( 'NONE',  ( 15.39524332970993470, 28.62968336403817204, 15.72805884749054250 ) ) ;
#32556=CARTESIAN_POINT ( 'NONE',  ( -15.37000524123853218, -27.20210912714291496, 15.72805884748939498 ) ) ;
#32558=CARTESIAN_POINT ( 'NONE',  ( 2.638259136957625817, 30.33190274691521182, 20.69868183039781329 ) ) ;
#32565=CARTESIAN_POINT ( 'NONE',  ( 24.07200259733946979, 7.872448391868417161, 16.30093088680184366 ) ) ;
#32575=CARTESIAN_POINT ( 'NONE',  ( -29.77970073067859147, -14.50783476829564300, 19.99202127657101613 ) ) ;
#32589=CARTESIAN_POINT ( 'NONE',  ( 37.88915195766877275, -19.37406375362064992, 22.99999999999999289 ) ) ;
#32600=CARTESIAN_POINT ( 'NONE',  ( 30.79094061804850568, -13.52614530981714225, 19.66345542862527651 ) ) ;
#32627=CARTESIAN_POINT ( 'NONE',  ( -19.84741737732755951, -16.23688957394095311, 20.99999999999999645 ) ) ;
#32638=CARTESIAN_POINT ( 'NONE',  ( -35.68447701591262700, -3.401722300707700430, 11.00000000000000000 ) ) ;
#32646=CARTESIAN_POINT ( 'NONE',  ( 14.48927117870123027, -30.61587158504688233, 3.000000000000000000 ) ) ;
#32651=CARTESIAN_POINT ( 'NONE',  ( -21.27192666516830499, -1.272056932884052971, 20.69868183039990228 ) ) ;
#32652=CARTESIAN_POINT ( 'NONE',  ( 25.15015781186010457, -9.899056496887492784, 20.99999999999999645 ) ) ;
#32657=CARTESIAN_POINT ( 'NONE',  ( 31.38526299860050628, -24.75545609243360090, 11.00000000000000000 ) ) ;
#32697=CYLINDRICAL_SURFACE ( 'NONE', #24471, 19.99999999999993250 ) ;
#32710=CARTESIAN_POINT ( 'NONE',  ( -6.761248272854020414, 33.72770196150105448, 18.87996532025709229 ) ) ;
#32729=CARTESIAN_POINT ( 'NONE',  ( -33.13502155305637586, -2.712192412331239755, 16.30093088680144930 ) ) ;
#32754=CARTESIAN_POINT ( 'NONE',  ( 17.04089262280485073, -28.02826808822959137, 15.13084544680119059 ) ) ;
#32756=CARTESIAN_POINT ( 'NONE',  ( 16.50691157469017867, 29.07214648649524591, 13.32518128616620778 ) ) ;
#32757=CARTESIAN_POINT ( 'NONE',  ( -15.89892447184056756, -25.15199583021358265, 17.92354375535250810 ) ) ;
#32759=CARTESIAN_POINT ( 'NONE',  ( 3.137032374298201365, 29.29040802067843074, 20.82122704794080192 ) ) ;
#32768=CARTESIAN_POINT ( 'NONE',  ( 14.75813536907442192, 8.520613428072293161, 20.69868183039781329 ) ) ;
#32773=CARTESIAN_POINT ( 'NONE',  ( -4.817371740575545402, 23.83900317890010001, 23.00000000000000000 ) ) ;
#32779=CARTESIAN_POINT ( 'NONE',  ( -30.23838254412105186, -12.22961151633805166, 19.99202127657104811 ) ) ;
#32789=FACE_BOUND ( 'NONE', #34187, .T. ) ;
#32799=CARTESIAN_POINT ( 'NONE',  ( -25.22779562677311560, -30.53001673900746837, 23.00000000000093792 ) ) ;
#32804=CARTESIAN_POINT ( 'NONE',  ( 32.53782915839349954, -12.43926102483652940, 18.87996532025783125 ) ) ;
#32818=FACE_OUTER_BOUND ( 'NONE', #20115, .T. ) ;
#32828=CARTESIAN_POINT ( 'NONE',  ( 24.65531199400543372, -28.60128534115915500, 10.99999999999989697 ) ) ;
#32839=CARTESIAN_POINT ( 'NONE',  ( -29.92393930196035257, -26.04303208588109086, 11.00000000000017941 ) ) ;
#32854=CARTESIAN_POINT ( 'NONE',  ( 24.49951449059906139, -14.14480128616252053, 20.99999999999999645 ) ) ;
#32858=CARTESIAN_POINT ( 'NONE',  ( 29.92393930195800422, -26.04303208588348184, 11.00000000000002487 ) ) ;
#32894=B_SPLINE_CURVE_WITH_KNOTS ( 'NONE', 3,
 ( #14744, #2157, #13782, #27133, #29227, #10539, #5396, #29025, #26174, #33247, #23883, #36479, #18002, #4443, #16845, #21040, #8647, #33449 ),
 .UNSPECIFIED., .F., .F.,
 ( 4, 2, 2, 2, 2, 2, 2, 2, 4 ),
 ( 0.000000000000000000, 0.1249999999999999167, 0.2499999999999998335, 0.3749999999999997780, 0.4999999999999996669, 0.6249999999999995559, 0.7499999999999995559, 0.8749999999999997780, 1.000000000000000000 ),
 .UNSPECIFIED. ) ;
#32910=CARTESIAN_POINT ( 'NONE',  ( 15.00309677617812376, 1.567672476142360383, 21.00000000000000000 ) ) ;
#32916=CARTESIAN_POINT ( 'NONE',  ( -2.590592964390336927, 26.81117624614021011, 23.00000000000000000 ) ) ;
#32926=CARTESIAN_POINT ( 'NONE',  ( 16.60464863832688565, -22.41657912773190375, 19.66345542862528362 ) ) ;
#32928=DIRECTION ( 'NONE',  ( -0.000000000000000000, -0.000000000000000000, -1.000000000000000000 ) ) ;
#32931=CARTESIAN_POINT ( 'NONE',  ( -35.93605200993580695, -16.45551934610077538, 14.53008259254024459 ) ) ;
#32945=CARTESIAN_POINT ( 'NONE',  ( -21.78011286655814871, -29.15515566786809032, 10.99999999999984546 ) ) ;
#32955=CARTESIAN_POINT ( 'NONE',  ( 30.37673449013164984, -23.61083502489066177, 15.72805884748940386 ) ) ;
#32957=CARTESIAN_POINT ( 'NONE',  ( -1.856244906471939737, 39.65430245495498696, 14.53008259254010959 ) ) ;
#32959=CARTESIAN_POINT ( 'NONE',  ( -10.60610353951573259, -24.43405348875333871, 17.42190598798822521 ) ) ;
#32961=CARTESIAN_POINT ( 'NONE',  ( -0.8947151973526094038, 30.76432767446198824, 20.69868183039781329 ) ) ;
#32971=CARTESIAN_POINT ( 'NONE',  ( 22.54917513123528394, -0.2132175735513469617, 20.25080042702448679 ) ) ;
#32984=CARTESIAN_POINT ( 'NONE',  ( -23.01245512501514057, -23.08877437847487002, 19.27171037444190205 ) ) ;
#32994=FACE_OUTER_BOUND ( 'NONE', #29410, .T. ) ;
#32999=CARTESIAN_POINT ( 'NONE',  ( 21.91981567634952199, -15.65087685632054004, 23.00000000000000000 ) ) ;
#33010=CARTESIAN_POINT ( 'NONE',  ( 29.95833833019052150, -4.698917079249050666, 19.27171037444192692 ) ) ;
#33016=CARTESIAN_POINT ( 'NONE',  ( -16.23042486173916288, -23.86708630543299847, 18.87996532025784191 ) ) ;
#33027=CARTESIAN_POINT ( 'NONE',  ( -33.75875814100324845, 2.759858869446484064, 23.00000000000000000 ) ) ;
#33032=CARTESIAN_POINT ( 'NONE',  ( 5.055868909836068070, -26.71495157282352650, 12.14047268033097460 ) ) ;
#33035=CARTESIAN_POINT ( 'NONE',  ( -26.61692196988933645, -13.50708991729978514, 20.82122704794079482 ) ) ;
#33044=CARTESIAN_POINT ( 'NONE',  ( -18.84564290660914310, -29.34375446593495695, 11.55979286843968801 ) ) ;
#33061=CARTESIAN_POINT ( 'NONE',  ( 18.52756972024298676, -17.82802275548051796, 20.94377226548369819 ) ) ;
#33119=CARTESIAN_POINT ( 'NONE',  ( 4.671113270415285790, 24.36520164658795551, 23.00000000000000000 ) ) ;
#33133=CARTESIAN_POINT ( 'NONE',  ( -35.73275206861759301, -5.440967016230455755, 14.53008259254057499 ) ) ;
#33156=CARTESIAN_POINT ( 'NONE',  ( 33.41351084210645439, -21.43470647212788194, 14.53008259254008472 ) ) ;
#33158=CARTESIAN_POINT ( 'NONE',  ( 1.888379873391452080, 39.95159812444028091, 13.92931973827809067 ) ) ;
#33161=CARTESIAN_POINT ( 'NONE',  ( -5.938964939928987441, -16.21345324574345170, 20.82122704794080192 ) ) ;
#33163=CARTESIAN_POINT ( 'NONE',  ( -6.050433455602103287E-14, 29.93655406406124087, 20.82122704794079837 ) ) ;
#33171=CARTESIAN_POINT ( 'NONE',  ( 21.91791918713443721, -0.7365302468260908064, 20.50957957746798854 ) ) ;
#33182=CARTESIAN_POINT ( 'NONE',  ( -19.02194587268434844, -24.34812480527924450, 18.87996532025819363 ) ) ;
#33208=CARTESIAN_POINT ( 'NONE',  ( 18.99711117635948554, -25.05170312385142495, 18.42518152272109333 ) ) ;
#33231=CARTESIAN_POINT ( 'NONE',  ( -5.078902502065747449, -26.44091005802452798, 13.32518128616608877 ) ) ;
#33235=CARTESIAN_POINT ( 'NONE',  ( -24.70330546561586615, -7.131334670376221041, 20.94377226548378701 ) ) ;
#33247=CARTESIAN_POINT ( 'NONE',  ( -23.54493052986482837, -14.21898406159469275, 21.00000000000000355 ) ) ;
#33253=CARTESIAN_POINT ( 'NONE',  ( 4.817371740575539185, 23.83900317890011422, 23.00000000000000000 ) ) ;
#33262=CARTESIAN_POINT ( 'NONE',  ( 25.00594398452619771, -16.29738563782240490, 20.82122704794094048 ) ) ;
#33264=CARTESIAN_POINT ( 'NONE',  ( 16.87498849720599736, -29.16588574430810255, 10.99999999999838352 ) ) ;
#33278=CARTESIAN_POINT ( 'NONE',  ( 4.881458130668207218, -28.77689918168226058, 11.00000000000000000 ) ) ;
#33288=CARTESIAN_POINT ( 'NONE',  ( 23.61737546510196850, -7.194424252577107382, 21.00000000000000355 ) ) ;
#33300=CARTESIAN_POINT ( 'NONE',  ( -32.33143948541735568, 1.358872982502395521, 11.55979286843934872 ) ) ;
#33330=MECHANICAL_DESIGN_GEOMETRIC_PRESENTATION_REPRESENTATION('',(#17117),#38494);
#33344=CARTESIAN_POINT ( 'NONE',  ( 33.75875814100317029, 2.759858869446390361, 3.000000000000000000 ) ) ;
#33352=ORIENTED_EDGE ( 'NONE', *, *, #9033, .T. ) ;
#33358=CARTESIAN_POINT ( 'NONE',  ( 31.72789954390550093, 0.7664678198853781543, 14.53008259254011492 ) ) ;
#33360=CARTESIAN_POINT ( 'NONE',  ( -14.19638663437040904, 32.12978188971815996, 14.53008259254011136 ) ) ;
#33362=CARTESIAN_POINT ( 'NONE',  ( 6.143904198944455608, -13.77689918168226235, 20.99999999999999645 ) ) ;
#33364=CARTESIAN_POINT ( 'NONE',  ( -3.166027244386082629, 31.89862848374658455, 20.25080042701565830 ) ) ;
#33368=CARTESIAN_POINT ( 'NONE',  ( -13.22866120779009336, 26.17694675929173798, 18.42518152272108267 ) ) ;
#33373=CARTESIAN_POINT ( 'NONE',  ( 14.79097147050401873, 14.99953367535683668, 19.66345542862543638 ) ) ;
#33376=CARTESIAN_POINT ( 'NONE',  ( -15.98961535660691347, 30.99268274074325902, 10.99999999999966604 ) ) ;
#33385=CARTESIAN_POINT ( 'NONE',  ( -27.44755207257315988, -22.53416897284578368, 18.42518152272109333 ) ) ;
#33401=CARTESIAN_POINT ( 'NONE',  ( 29.22254794995044946, -28.85350742528273926, 22.99999999999905853 ) ) ;
#33402=ORIENTED_EDGE ( 'NONE', *, *, #3444, .T. ) ;
#33410=CARTESIAN_POINT ( 'NONE',  ( 34.17506821248620952, -14.20748230372561238, 17.42190598798392998 ) ) ;
#33433=CARTESIAN_POINT ( 'NONE',  ( 10.19059090746689833, -26.87498467585813344, 13.92931973827711900 ) ) ;
#33436=CARTESIAN_POINT ( 'NONE',  ( -26.10558707266139677, -11.85287147006304309, 20.94377226548378346 ) ) ;
#33441=ORIENTED_EDGE ( 'NONE', *, *, #38997, .T. ) ;
#33449=CARTESIAN_POINT ( 'NONE',  ( -18.23649648353780961, -16.09146789626143814, 20.99999999999999645 ) ) ;
#33454=FACE_OUTER_BOUND ( 'NONE', #1204, .T. ) ;
#33455=CARTESIAN_POINT ( 'NONE',  ( -32.33143948541797386, 1.358872982501903248, 11.00000000000000000 ) ) ;
#33463=CARTESIAN_POINT ( 'NONE',  ( 19.22070351544489597, -18.72532327798363383, 20.82122704794079482 ) ) ;
#33466=CARTESIAN_POINT ( 'NONE',  ( 37.09709568333403240, -7.051483854461488399, 11.00000000000007994 ) ) ;
#33473=CARTESIAN_POINT ( 'NONE',  ( 10.34254640628217992, 25.37474234120048067, 19.99202127657104100 ) ) ;
#33503=CARTESIAN_POINT ( 'NONE',  ( -18.69515074622356821, 22.45407711376244109, 11.00000000002425971 ) ) ;
#33553=ORIENTED_EDGE ( 'NONE', *, *, #29419, .T. ) ;
#33555=CARTESIAN_POINT ( 'NONE',  ( 35.73276616393376770, -5.440996109072101738, 14.53008259253983248 ) ) ;
#33557=CARTESIAN_POINT ( 'NONE',  ( 16.52773037515741805, 27.09393310379826758, 14.53008259254011136 ) ) ;
#33559=CARTESIAN_POINT ( 'NONE',  ( 4.307564594982224211E-14, -17.04122685614420263, 20.69868183039781684 ) ) ;
#33561=CARTESIAN_POINT ( 'NONE',  ( -8.773674293808889584E-14, 33.23463598332012481, 19.99202127657103034 ) ) ;
#33562=CIRCLE ( 'NONE', #8229, 59.99999999999995026 ) ;
#33569=CARTESIAN_POINT ( 'NONE',  ( 11.07177992392776567, 13.25002113302786988, 20.82122704794082679 ) ) ;
#33578=CARTESIAN_POINT ( 'NONE',  ( -25.82842257350429804, -22.71926374633573786, 18.87996532025750440 ) ) ;
#33594=CARTESIAN_POINT ( 'NONE',  ( 36.53988293556081857, -0.5802930328954534200, 11.00000000000000000 ) ) ;
#33605=CARTESIAN_POINT ( 'NONE',  ( 32.11924139737163841, -16.82817082614038995, 18.42518152272108622 ) ) ;
#33610=CARTESIAN_POINT ( 'NONE',  ( 2.594149110900703992, 26.80855565015188446, 20.99999999999999645 ) ) ;
#33611=CARTESIAN_POINT ( 'NONE',  ( -15.00437666251167101, -28.61930095463374357, 12.14047268033097637 ) ) ;
#33629=CARTESIAN_POINT ( 'NONE',  ( -10.19059090746470098, -26.87498467587872142, 13.92931973828929770 ) ) ;
#33632=CARTESIAN_POINT ( 'NONE',  ( -26.01028601707387011, -6.099477938991039849, 20.69868183039782394 ) ) ;
#33651=DIRECTION ( 'NONE',  ( -1.000000000000000000, 0.000000000000000000, 0.000000000000000000 ) ) ;
#33658=CARTESIAN_POINT ( 'NONE',  ( 25.52323811238489881, -15.66556294379320136, 20.82122704794079837 ) ) ;
#33670=CARTESIAN_POINT ( 'NONE',  ( 8.768078002822829120, 24.93711404285870969, 20.50957957746028981 ) ) ;
#33691=CARTESIAN_POINT ( 'NONE',  ( 34.33271598312541784, -24.82403719196558001, 11.00000000000000000 ) ) ;
#33700=CARTESIAN_POINT ( 'NONE',  ( -31.72789954390187006, 0.7664678198892422856, 14.53008259254010959 ) ) ;
#33723=CARTESIAN_POINT ( 'NONE',  ( 2.113538555224950155, 27.06402972250564432, 23.00000000000000355 ) ) ;
#33760=CARTESIAN_POINT ( 'NONE',  ( -10.77072277543642187, 36.67279993932645255, 12.73282698324853079 ) ) ;
#33761=CARTESIAN_POINT ( 'NONE',  ( -12.15426487966493596, -15.33773963145039332, 20.99999999999999645 ) ) ;
#33763=CARTESIAN_POINT ( 'NONE',  ( -8.084330871572442234, 26.79335594083840633, 20.50957957746031113 ) ) ;
#33767=CARTESIAN_POINT ( 'NONE',  ( -14.97058623676949729, 26.66112013780927015, 16.87380292611441845 ) ) ;
#33779=CARTESIAN_POINT ( 'NONE',  ( -32.23453252384940271, -8.210301902002639096, 18.87996532025712071 ) ) ;
#33792=CARTESIAN_POINT ( 'NONE',  ( 33.75875814100313477, 2.759858869446413010, 23.00000000000000000 ) ) ;
#33803=CARTESIAN_POINT ( 'NONE',  ( 23.78889779961332707, -25.69434382178437914, 17.42190598798433854 ) ) ;
#33809=CARTESIAN_POINT ( 'NONE',  ( -36.58707756785061349, -5.516531573120356136, 11.00000000000008527 ) ) ;
#33824=CARTESIAN_POINT ( 'NONE',  ( -23.85459647502774416, -16.20858856896902367, 20.94377226548378346 ) ) ;
#33851=CARTESIAN_POINT ( 'NONE',  ( 17.42101839920122686, -19.25229542401860527, 20.69868183039781684 ) ) ;
#33856=ORIENTED_EDGE ( 'NONE', *, *, #37498, .F. ) ;
#33873=CARTESIAN_POINT ( 'NONE',  ( -9.762586613238248390, -29.39641002289260285, 11.00000000000000000 ) ) ;
#33877=CARTESIAN_POINT ( 'NONE',  ( 24.20198940123850306, -6.620595927253059010, 20.94377226548378701 ) ) ;
#33883=CARTESIAN_POINT ( 'NONE',  ( -36.50335543116000991, -9.090109797570214312, 14.53008259254010959 ) ) ;
#33893=CARTESIAN_POINT ( 'NONE',  ( -31.94006737154283471, 0.9747213384881107112, 13.92931973827808534 ) ) ;
#33899=EDGE_LOOP ( 'NONE', ( #2930, #13880, #33402, #38636 ) ) ;
#33944=CARTESIAN_POINT ( 'NONE',  ( 13.54525386577604351, 33.99767725470013602, 13.32518128616618469 ) ) ;
#33945=CARTESIAN_POINT ( 'NONE',  ( -6.077490221915047286, -14.56650175400723946, 20.99999999999999645 ) ) ;
#33946=LINE ( 'NONE', #37390, #32534 ) ;
#33948=CARTESIAN_POINT ( 'NONE',  ( -9.535956184589343465, 27.56440042312200589, 19.99202127657105166 ) ) ;
#33968=CARTESIAN_POINT ( 'NONE',  ( -34.55475982899667287, -10.97206003969062849, 17.42190598798472934 ) ) ;
#33970=ADVANCED_FACE ( 'NONE', ( #15517 ), #38245, .F. ) ;
#33994=CARTESIAN_POINT ( 'NONE',  ( 18.97485329855508240, -25.68201384536907383, 17.92354375535252942 ) ) ;
#34007=CARTESIAN_POINT ( 'NONE',  ( 28.36971490933128948, 4.612181732476346774, 13.92931973828039638 ) ) ;
#34018=CARTESIAN_POINT ( 'NONE',  ( -28.21258359973651508, -14.01198379553961537, 20.50957957746028626 ) ) ;
#34029=ORIENTED_EDGE ( 'NONE', *, *, #29059, .T. ) ;
#34043=CARTESIAN_POINT ( 'NONE',  ( -29.22587408525591712, -28.78382723770691243, 11.00000000000000000 ) ) ;
#34044=CARTESIAN_POINT ( 'NONE',  ( 26.76156665933390499, -9.514918190647627227, 20.82122704794079837 ) ) ;
#34076=CARTESIAN_POINT ( 'NONE',  ( -26.00889624226697805, -26.79364542773710767, 15.13084544680213561 ) ) ;
#34087=CARTESIAN_POINT ( 'NONE',  ( -20.66414367076832903, 17.76245163069107491, 10.99999999999809219 ) ) ;
#34116=CARTESIAN_POINT ( 'NONE',  ( 19.26948696230205371, 27.85601271560038938, 22.99999999999999289 ) ) ;
#34147=CARTESIAN_POINT ( 'NONE',  ( -17.15083734909590163, 27.26712758905546252, 12.73282698324853257 ) ) ;
#34151=CARTESIAN_POINT ( 'NONE',  ( -8.129960429723110135E-14, 32.41755745572908864, 20.25080042701565830 ) ) ;
#34157=B_SPLINE_CURVE_WITH_KNOTS ( 'NONE', 3,
 ( #8318, #17477, #27396, #14208, #20720, #21306 ),
 .UNSPECIFIED., .F., .F.,
 ( 4, 2, 4 ),
 ( 0.000000000000000000, 0.5000000000000000000, 1.000000000000000000 ),
 .UNSPECIFIED. ) ;
#34168=CARTESIAN_POINT ( 'NONE',  ( -25.28418022016644429, -25.06680681775936037, 17.42190598798392998 ) ) ;
#34187=EDGE_LOOP ( 'NONE', ( #32039, #17111, #33553, #34821, #18897, #25726, #2458 ) ) ;
#34192=CARTESIAN_POINT ( 'NONE',  ( 23.42865034949090841, -24.48547250943625997, 18.42518152272149479 ) ) ;
#34203=CARTESIAN_POINT ( 'NONE',  ( 18.69515074622676920, 22.45407711375075621, 10.99999999997785771 ) ) ;
#34214=CARTESIAN_POINT ( 'NONE',  ( -25.50184330511921260, -18.07811769911583255, 20.50957957746029336 ) ) ;
#34215=CARTESIAN_POINT ( 'NONE',  ( -19.48557158514998022, -11.24999999999982414, 23.00000000000000000 ) ) ;
#34240=CARTESIAN_POINT ( 'NONE',  ( -22.03614745501234040, -31.14480216356518127, 11.00000000000000000 ) ) ;
#34241=CARTESIAN_POINT ( 'NONE',  ( 23.91569629078776771, -19.26019901638226273, 20.50957957746005889 ) ) ;
#34275=CARTESIAN_POINT ( 'NONE',  ( -33.53883321253935890, -0.1552552779192388210, 12.73282698324824480 ) ) ;
#34287=CARTESIAN_POINT ( 'NONE',  ( -23.18043107539034509, 0.3100950997616090943, 19.99202127657445516 ) ) ;
#34293=CARTESIAN_POINT ( 'NONE',  ( 36.22115687806114437, -16.54570019420276594, 13.92931973827800185 ) ) ;
#34347=CARTESIAN_POINT ( 'NONE',  ( -1.940950748631915967, 40.43805239114131211, 12.14047268033097460 ) ) ;
#34350=CARTESIAN_POINT ( 'NONE',  ( -11.47663208683763614, 27.06976447313135381, 19.27171037444124835 ) ) ;
#34368=CARTESIAN_POINT ( 'NONE',  ( -33.86703583613317647, -12.56047426484087914, 17.92354375535250810 ) ) ;
#34372=VERTEX_POINT ( 'NONE', #35715 ) ;
#34380=CARTESIAN_POINT ( 'NONE',  ( 34.33271597229082772, -24.82403720151193482, 11.00000000000000000 ) ) ;
#34381=ORIENTED_EDGE ( 'NONE', *, *, #38997, .F. ) ;
#34390=CARTESIAN_POINT ( 'NONE',  ( 30.06723386280229704, -23.25956985441296609, 16.30093088680191471 ) ) ;
#34402=CARTESIAN_POINT ( 'NONE',  ( 20.16616670141972278, 17.52816929147979508, 13.92931973827773362 ) ) ;
#34411=CARTESIAN_POINT ( 'NONE',  ( -27.94267546441488648, -5.959640785454821454, 20.25080042701541316 ) ) ;
#34438=CARTESIAN_POINT ( 'NONE',  ( 18.16616693041810748, -20.30807083247596623, 20.50957957746011573 ) ) ;
#34456=CARTESIAN_POINT ( 'NONE',  ( -17.34253826607186966, 27.32041144404028188, 11.00000000000000000 ) ) ;
#34473=CARTESIAN_POINT ( 'NONE',  ( -34.78305373678684731, -20.08200543817108752, 13.32518128616608699 ) ) ;
#34480=CARTESIAN_POINT ( 'NONE',  ( -18.23649648353780961, -16.09146789626143814, 23.00000000000000000 ) ) ;
#34481=CARTESIAN_POINT ( 'NONE',  ( 6.553841457908355927, 36.68830644081927517, 16.87380292611439003 ) ) ;
#34485=CARTESIAN_POINT ( 'NONE',  ( -30.90861030616023086, -0.03770625498002080217, 16.30093088680190760 ) ) ;
#34491=CARTESIAN_POINT ( 'NONE',  ( 16.90387162101912111, -28.96785393638771566, 12.73282698324709372 ) ) ;
#34511=CARTESIAN_POINT ( 'NONE',  ( 17.76739295965463583, 31.93461338995192378, 11.00000000000000000 ) ) ;
#34541=CARTESIAN_POINT ( 'NONE',  ( 17.28285333400958734, 27.30382183500221061, 12.14047268033097460 ) ) ;
#34543=CARTESIAN_POINT ( 'NONE',  ( -15.01937947523880545, 1.539368754276113638, 22.99999999999999289 ) ) ;
#34544=CARTESIAN_POINT ( 'NONE',  ( 11.47663208683638025, 27.06976447313250489, 19.27171037444299984 ) ) ;
#34563=CARTESIAN_POINT ( 'NONE',  ( -25.04152548477492957, -24.48861404543249165, 17.92354375535250810 ) ) ;
#34586=CARTESIAN_POINT ( 'NONE',  ( 34.35058160601991517, -9.363338975648222373, 17.42190598798392642 ) ) ;
#34589=CARTESIAN_POINT ( 'NONE',  ( 1.254079983865269199, 28.18681535329830368, 21.00000000000000355 ) ) ;
#34593=AXIS2_PLACEMENT_3D ( 'NONE', #23512, #27163, #17434 ) ;
#34597=CARTESIAN_POINT ( 'NONE',  ( 18.69515074622073314, 22.45407711374831194, 11.55979286841757414 ) ) ;
#34606=CARTESIAN_POINT ( 'NONE',  ( -24.31339772227793716, -19.97941014234552881, 20.25080042701540961 ) ) ;
#34633=CARTESIAN_POINT ( 'NONE',  ( 16.80389827882015297, -21.64427909825937490, 19.99202127657103389 ) ) ;
#34642=CARTESIAN_POINT ( 'NONE',  ( -75.15099915297791711, 43.38844959084113384, 23.00000000000000000 ) ) ;
#34664=B_SPLINE_SURFACE_WITH_KNOTS ( 'NONE', 3, 3, ( 
 ( #20053, #28785, #7038, #7237, #31830, #960, #558, #22680, #13337, #25731, #10299, #16603, #13542, #1359, #13743, #4202, #7650, #25331, #35083, #32448, #19637, #12940, #29588, #4808, #5605 ),
 ( #39130, #1766, #17623, #17213, #38735, #27148, #8253, #11511, #14553, #30199, #14150, #17822, #32854, #29387, #8662, #5006, #26341, #36096, #39533, #32652, #17419, #14353, #20662, #11110, #26549 ),
 ( #39334, #33061, #11710, #26947, #5210, #38935, #2372, #8049, #10915, #14757, #26743, #29794, #23299, #23896, #35692, #1977, #24097, #36492, #20254, #35891, #21054, #7847, #5410, #23494, #20459 ),
 ( #11314, #23697, #33463, #29993, #2169, #36299, #8461, #1563, #13947, #20860, #33262, #33658, #11907, #28135, #12303, #21838, #30798, #3353, #8861, #34044, #18210, #27543, #21445, #24490, #30991 ),
 ( #33851, #9460, #6203, #15153, #3160, #2760, #5809, #24690, #6395, #39928, #27938, #9060, #12105, #25088, #37087, #12498, #312, #36890, #24890, #22040, #37284, #37485, #36696, #9256, #21641 ),
 ( #30602, #34438, #112, #5999, #27738, #21248, #18406, #34241, #2962, #18802, #15349, #31187, #15745, #9662, #40125, #12694, #15551, #18606, #18013, #30405, #39732, #2570, #14955, #27343, #24298 ),
 ( #19796, #16757, #22833, #16551, #38074, #29138, #4146, #13285, #22228, #32191, #25475, #3551, #7391, #3947, #10049, #15950, #28933, #28330, #22427, #4350, #1311, #37682, #13085, #35233, #510 ),
 ( #34633, #1112, #12894, #34832, #25287, #10656, #706, #28730, #28533, #37874, #13692, #26080, #38481, #22631, #6784, #9850, #23037, #909, #10450, #19387, #6588, #19190, #35038, #31578, #16148 ),
 ( #3744, #6981, #18995, #31784, #38281, #7190, #16346, #19589, #25681, #10246, #31980, #31384, #13489, #25881, #26494, #32600, #2318, #14301, #29939, #17771, #1720, #2119, #39485, #14501, #14707 ),
 ( #26291, #10859, #35643, #26892, #29742, #7999, #38888, #23448, #29541, #35838, #20203, #1924, #4555, #35440, #30147, #39081, #36250, #20001, #39281, #38686, #27096, #11664, #33010, #26692, #23248 ),
 ( #23648, #7802, #36044, #11460, #20808, #7597, #32401, #16958, #20409, #4759, #17166, #29339, #14097, #11063, #23847, #1511, #32804, #17567, #13901, #4962, #17370, #11259, #8206, #20611, #5159 ),
 ( #8414, #5357, #33208, #39684, #17962, #34192, #18353, #27889, #36837, #9407, #14908, #40075, #24246, #33605, #27490, #30553, #37037, #36441, #2711, #30749, #15102, #6345, #11855, #15503, #39875 ),
 ( #12449, #21200, #33994, #12051, #5756, #31142, #2908, #18552, #18752, #24442, #30944, #28084, #3109, #3305, #2519, #15299, #27687, #27296, #18162, #36642, #263, #5952, #8811, #9007, #21397 ),
 ( #9207, #6151, #12251, #24840, #8607, #33803, #61, #30351, #24049, #24641, #21591, #21004, #37238, #21787, #15695, #33410, #5553, #22585, #34586, #31931, #31536, #7141, #13442, #19748, #25238 ),
 ( #12650, #32141, #16099, #9609, #19343, #22783, #15900, #28484, #37826, #31735, #6737, #28287, #19144, #37435, #16297, #6541, #38235, #7341, #29089, #25038, #13040, #37638, #464, #18946, #12848 ),
 ( #28886, #9805, #3702, #28684, #4303, #16706, #25836, #22184, #658, #34390, #21990, #25429, #10000, #10406, #22378, #34785, #31334, #6936, #1062, #859, #3900, #3505, #13239, #35185, #25630 ),
 ( #38028, #10202, #34992, #19541, #4100, #16504, #32553, #23795, #16911, #32955, #20154, #17718, #4711, #20558, #26642, #11412, #5111, #36196, #29889, #23600, #39031, #7949, #11209, #1264, #20359 ),
 ( #19952, #32754, #4909, #32349, #38635, #4508, #5308, #23398, #1464, #29293, #10810, #17317, #1875, #14251, #35997, #29691, #2071, #26035, #13848, #17518, #7550, #13647, #26240, #23196, #38434 ),
 ( #11013, #35594, #8153, #7751, #10607, #39233, #14447, #26842, #8362, #20762, #17115, #33156, #29491, #22988, #35392, #1667, #14047, #26439, #38838, #35793, #33555, #15049, #9509, #11806, #33358 ),
 ( #364, #21889, #12945, #28187, #37338, #5501, #3605, #8759, #27046, #31439, #27987, #9713, #37736, #8556, #34293, #6447, #20951, #27242, #17914, #34686, #12551, #30298, #2469, #39630, #18851 ),
 ( #39431, #30094, #25336, #31241, #16001, #14656, #22093, #14857, #9905, #12745, #2268, #6641, #11612, #161, #24192, #3403, #36589, #23995, #28386, #15798, #25139, #37539, #562, #21148, #19047 ),
 ( #5704, #34491, #36392, #18114, #30502, #22286, #2662, #24942, #6839, #32452, #29392, #35495, #29195, #10504, #1568, #16811, #25933, #34889, #4613, #38130, #16201, #20059, #16606, #22683, #28587 ),
 ( #31635, #19641, #3999, #7041, #13141, #19440, #31834, #38533, #13951, #16399, #1364, #25531, #35087, #759, #23303, #13343, #1164, #963, #25734, #17013, #26346, #38739, #35289, #28789, #37933 ),
 ( #7447, #10302, #10102, #38333, #10920, #22482, #7240, #13546, #32036, #4205, #28989, #35699, #22884, #10709, #19855, #32244, #4409, #13747, #26138, #23093, #7655, #19240, #3803, #39134, #5009 ),
 ( #30201, #33264, #14558, #5413, #7852, #26951, #14957, #17218, #32858, #32657, #21056, #18016, #24100, #17825, #39338, #30409, #2375, #11514, #23498, #33466, #26746, #4812, #8664, #5214, #11318 ) ),
 .UNSPECIFIED., .F., .F., .F.,
 ( 4, 3, 3, 3, 3, 3, 3, 3, 4 ),
 ( 4, 3, 3, 3, 3, 3, 3, 3, 4 ),
 ( 0.000000000000000000, 0.1250000000000000000, 0.2500000000000000000, 0.3750000000000000000, 0.5000000000000000000, 0.6250000000000000000, 0.7500000000000000000, 0.8750000000000000000, 1.000000000000000000 ),
 ( 4.459899766721566294, 4.784821457936500266, 5.109743149151433350, 5.434664840366366434, 5.759586531581300406, 6.084508222796233490, 6.409429914011166574, 6.734351605226100546, 7.059273296441033629 ),
 .UNSPECIFIED. ) ;
#34668=CARTESIAN_POINT ( 'NONE',  ( -18.85268948302541148, -29.14375172063097352, 12.73282698324892692 ) ) ;
#34676=CARTESIAN_POINT ( 'NONE',  ( 14.00263291006742605, 28.07534605034063446, 17.42190598798543633 ) ) ;
#34681=CARTESIAN_POINT ( 'NONE',  ( -15.26743640742121677, 21.18345451744725594, 17.92354375535531830 ) ) ;
#34686=CARTESIAN_POINT ( 'NONE',  ( 36.56052011373606092, -7.179325806536988708, 13.92931973827813330 ) ) ;
#34741=CARTESIAN_POINT ( 'NONE',  ( 10.89111091687317234, 36.83121428896964744, 10.99999999999999822 ) ) ;
#34742=CARTESIAN_POINT ( 'NONE',  ( -1.829593030691901284E-15, 22.50000000000001066, 2.999999999999999112 ) ) ;
#34745=CARTESIAN_POINT ( 'NONE',  ( -1.015221176887233153E-13, 34.78122644969442945, 19.27171037444156454 ) ) ;
#34757=CARTESIAN_POINT ( 'NONE',  ( -1.082972213713691678, 27.41125570341915818, 20.99999999999999645 ) ) ;
#34764=CARTESIAN_POINT ( 'NONE',  ( -17.31264644459998792, -26.16430884515780164, 17.42190598798388379 ) ) ;
#34785=CARTESIAN_POINT ( 'NONE',  ( 35.17699530642156702, -14.40920341950727668, 16.30093088680190760 ) ) ;
#34787=CARTESIAN_POINT ( 'NONE',  ( 14.95773623273977293, 28.45553334945067903, 16.30093088680319369 ) ) ;
#34790=CARTESIAN_POINT ( 'NONE',  ( -0.7155976380802748782, 29.10878045366047928, 20.94377226548378346 ) ) ;
#34796=CARTESIAN_POINT ( 'NONE',  ( 20.57776646309868340, 11.88057900679090473, 17.42190598798392998 ) ) ;
#34803=CARTESIAN_POINT ( 'NONE',  ( -28.87886496472023623, -7.891943102185759784, 20.25080042701591765 ) ) ;
#34821=ORIENTED_EDGE ( 'NONE', *, *, #11909, .T. ) ;
#34832=CARTESIAN_POINT ( 'NONE',  ( 20.26242815737391822, -21.95648885305471865, 19.99202127657103034 ) ) ;
#34871=CARTESIAN_POINT ( 'NONE',  ( -37.28086807198960884, -8.991428209509251701, 12.14047268033097282 ) ) ;
#34877=DIRECTION ( 'NONE',  ( -0.000000000000000000, -0.000000000000000000, -1.000000000000000000 ) ) ;
#34878=CARTESIAN_POINT ( 'NONE',  ( -14.52022913577126317, 28.28138333486104017, 16.87380292611391042 ) ) ;
#34883=CARTESIAN_POINT ( 'NONE',  ( -14.67741354589487734, 20.96472719010613872, 18.42518152272275955 ) ) ;
#34889=CARTESIAN_POINT ( 'NONE',  ( 37.38745755834691664, -10.91949489986236799, 12.73282698324846862 ) ) ;
#34894=PLANE ( 'NONE',  #3909 ) ;
#34943=CARTESIAN_POINT ( 'NONE',  ( 7.591957726968737497, 38.93640765974105733, 11.55979286843916576 ) ) ;
#34947=CARTESIAN_POINT ( 'NONE',  ( -4.864422697792210926, 33.03032433378080412, 19.66345542862530849 ) ) ;
#34954=ADVANCED_FACE ( 'NONE', ( #1946 ), #9019, .F. ) ;
#34968=CARTESIAN_POINT ( 'NONE',  ( -17.09641143070615499, -27.64751350299154353, 15.72805884748921379 ) ) ;
#34992=CARTESIAN_POINT ( 'NONE',  ( 18.89973329987769901, -27.81027420697393993, 15.72805884748954064 ) ) ;
#34994=CARTESIAN_POINT ( 'NONE',  ( 6.751265526280336715, 37.11581529111865763, 16.30093088680186497 ) ) ;
#34997=CARTESIAN_POINT ( 'NONE',  ( -5.870940266647052930, 25.61771140527362434, 20.94377226548378701 ) ) ;
#34998=VECTOR ( 'NONE', #39499, 1000.000000000000000 ) ;
#35005=CARTESIAN_POINT ( 'NONE',  ( 27.91036560780102604, 4.231346453961702281, 15.13084544680861221 ) ) ;
#35013=CARTESIAN_POINT ( 'NONE',  ( -31.03731131718960157, -12.30244853585585041, 19.66345542862529783 ) ) ;
#35034=CARTESIAN_POINT ( 'NONE',  ( -23.74914942275209384, -8.582573258223623824, 23.00000000000000000 ) ) ;
#35038=CARTESIAN_POINT ( 'NONE',  ( 28.63944909880341072, -5.523819906327855911, 19.99202127657133232 ) ) ;
#35057=DIRECTION ( 'NONE',  ( 1.000000000000000000, 0.000000000000000000, 0.000000000000000000 ) ) ;
#35068=CARTESIAN_POINT ( 'NONE',  ( -22.67025966227462419, -28.72937007811335874, 13.32518128616567132 ) ) ;
#35076=CARTESIAN_POINT ( 'NONE',  ( 15.33540831873581212, 35.51988610398912272, 11.00000000000000000 ) ) ;
#35078=CARTESIAN_POINT ( 'NONE',  ( 9.066401385853238182, 34.43014579340820092, 17.42190598798392998 ) ) ;
#35081=CARTESIAN_POINT ( 'NONE',  ( -24.07200259734583270, 7.872448391864142359, 16.30093088680252578 ) ) ;
#35083=CARTESIAN_POINT ( 'NONE',  ( 24.44578022397283945, -10.62045233751072004, 20.99999999999999645 ) ) ;
#35087=CARTESIAN_POINT ( 'NONE',  ( 35.02038065029451275, -20.21902619557050684, 12.14047268033097460 ) ) ;
#35099=CARTESIAN_POINT ( 'NONE',  ( 3.863783140547853712E-14, -86.77689918168233874, 2.999999999999999112 ) ) ;
#35108=CARTESIAN_POINT ( 'NONE',  ( -18.68934290552931543, 29.94321432092452895, 22.99999999999905853 ) ) ;
#35112=CIRCLE ( 'NONE', #26027, 60.00000000000007816 ) ;
#35115=CARTESIAN_POINT ( 'NONE',  ( -23.20062861290008627, -14.64054034232861135, 22.99999999999999645 ) ) ;
#35141=CARTESIAN_POINT ( 'NONE',  ( 14.89626057892312616, 32.60452476689637535, 11.00000000000000000 ) ) ;
#35144=CARTESIAN_POINT ( 'NONE',  ( 2.660873612011785294, 34.56296969693364218, 19.27171037444156454 ) ) ;
#35148=LINE ( 'NONE', #16667, #2710 ) ;
#35153=AXIS2_PLACEMENT_3D ( 'NONE', #12758, #3617, #16013 ) ;
#35162=CARTESIAN_POINT ( 'NONE',  ( -22.28718831901767317, -26.62569216358780011, 16.87380292611400989 ) ) ;
#35185=CARTESIAN_POINT ( 'NONE',  ( 32.12208287522988570, -1.273987114062791859, 16.30093088680380120 ) ) ;
#35187=CARTESIAN_POINT ( 'NONE',  ( 15.42165057838460029, 26.78649484830278027, 16.30093088680190050 ) ) ;
#35189=CARTESIAN_POINT ( 'NONE',  ( 0.7155976380801669645, 29.10878045366049349, 20.94377226548378346 ) ) ;
#35197=CARTESIAN_POINT ( 'NONE',  ( 16.37862447359607287, 21.59537890659658288, 16.87380292610781396 ) ) ;
#35200=DIRECTION ( 'NONE',  ( -0.000000000000000000, -0.000000000000000000, -1.000000000000000000 ) ) ;
#35204=ADVANCED_FACE ( 'NONE', ( #3974 ), #28760, .F. ) ;
#35205=CARTESIAN_POINT ( 'NONE',  ( -28.84864528223463864, -18.09713003384587182, 19.66345542862496387 ) ) ;
#35233=CARTESIAN_POINT ( 'NONE',  ( 27.31543141964077037, -5.069059863653875730, 20.25080042701695859 ) ) ;
#35244=DIRECTION ( 'NONE',  ( -0.000000000000000000, -0.000000000000000000, -1.000000000000000000 ) ) ;
#35260=CARTESIAN_POINT ( 'NONE',  ( -23.19735768193461567, -14.64350930037788068, 21.00000000000000000 ) ) ;
#35270=CARTESIAN_POINT ( 'NONE',  ( -26.42723928173377246, -27.79046472072431584, 12.14047268033097460 ) ) ;
#35279=CARTESIAN_POINT ( 'NONE',  ( 4.783493507397931666, 36.70021839994227975, 17.42190598798392998 ) ) ;
#35283=CARTESIAN_POINT ( 'NONE',  ( -8.859192577249674017, 12.20922670551869516, 20.99999999999999645 ) ) ;
#35289=CARTESIAN_POINT ( 'NONE',  ( 34.78242786800331743, -1.681962577801997760, 12.14047268033102966 ) ) ;
#35292=ORIENTED_EDGE ( 'NONE', *, *, #4049, .T. ) ;
#35309=CARTESIAN_POINT ( 'NONE',  ( -18.23649648353780961, -16.09146789626143814, 23.00000000000000000 ) ) ;
#35315=CARTESIAN_POINT ( 'NONE',  ( -21.92386325230624067, -15.64910744109602625, 23.00000000000000355 ) ) ;
#35343=CARTESIAN_POINT ( 'NONE',  ( 9.340438144417252175, 38.00965938232027952, 11.55979286843940024 ) ) ;
#35348=CARTESIAN_POINT ( 'NONE',  ( -12.19686730905342209, 28.97781536196876928, 18.42518152272111109 ) ) ;
#35368=CARTESIAN_POINT ( 'NONE',  ( -31.24272016125062024, 0.2902395683499273682, 15.72805884748940031 ) ) ;
#35392=CARTESIAN_POINT ( 'NONE',  ( 35.93605200993547300, -16.45551934609908429, 14.53008259254004386 ) ) ;
#35394=CARTESIAN_POINT ( 'NONE',  ( 12.92636675529317891, 33.47246997465054363, 15.13084544680219423 ) ) ;
#35395=CARTESIAN_POINT ( 'NONE',  ( 5.594491472542083343, -20.30912387778604966, 19.66345542862528717 ) ) ;
#35397=CARTESIAN_POINT ( 'NONE',  ( -1.431596709943599777, 28.99142433710769495, 20.94377226548377990 ) ) ;
#35404=CARTESIAN_POINT ( 'NONE',  ( 24.45776404695103778, 8.140618660892668501, 15.72805884748940386 ) ) ;
#35413=CARTESIAN_POINT ( 'NONE',  ( -23.63966112704447298, -21.14828014214127805, 19.99202127657103389 ) ) ;
#35440=CARTESIAN_POINT ( 'NONE',  ( 30.78606151651052159, -16.23943018785194781, 19.27171037444156454 ) ) ;
#35465=CARTESIAN_POINT ( 'NONE',  ( -24.22138565352714323, -9.557272464391497024, 20.99999999999999645 ) ) ;
#35476=CARTESIAN_POINT ( 'NONE',  ( -35.02038065029437774, -20.21902619557053526, 12.14047268033097282 ) ) ;
#35488=CARTESIAN_POINT ( 'NONE',  ( -11.08993573050815939, 19.63476728485979095, 20.25080042701544514 ) ) ;
#35495=CARTESIAN_POINT ( 'NONE',  ( 33.93864557196972243, -21.81860479675949804, 12.73282698324848461 ) ) ;
#35506=CARTESIAN_POINT ( 'NONE',  ( 33.75875814100317029, 2.759858869446390361, 11.00000000000000000 ) ) ;
#35543=CARTESIAN_POINT ( 'NONE',  ( -14.89626057892323630, 32.60452476689623325, 11.55979286843934872 ) ) ;
#35547=CARTESIAN_POINT ( 'NONE',  ( 9.490716042091355220, 32.53254263376074817, 18.42518152272108622 ) ) ;
#35567=CARTESIAN_POINT ( 'NONE',  ( -34.83511892542295385, -16.10726664691095067, 16.30093088680195024 ) ) ;
#35594=CARTESIAN_POINT ( 'NONE',  ( 16.99774364072579758, -28.32416636927767328, 14.53008259253903489 ) ) ;
#35597=CARTESIAN_POINT ( 'NONE',  ( -8.548670570953216696, 36.69528512485481997, 15.72805884748861693 ) ) ;
#35599=CARTESIAN_POINT ( 'NONE',  ( 5.468510220371463504, -21.80712738496724157, 18.87996532025784902 ) ) ;
#35601=CARTESIAN_POINT ( 'NONE',  ( 6.154269285972487680, 26.67460248448178461, 20.82122704794080192 ) ) ;
#35608=CARTESIAN_POINT ( 'NONE',  ( 17.61963632522081369, 22.05541241827695842, 15.13084544678993559 ) ) ;
#35619=CARTESIAN_POINT ( 'NONE',  ( -29.98847540738097806, -8.745685015165189924, 19.99202127657046191 ) ) ;
#35632=CARTESIAN_POINT ( 'NONE',  ( 18.77248997590692170, -31.35432035706033105, 22.99999999999999289 ) ) ;
#35643=CARTESIAN_POINT ( 'NONE',  ( 19.04856739887212669, -23.59522229971750917, 19.27171037444155388 ) ) ;
#35647=ADVANCED_FACE ( 'NONE', ( #24865 ), #37259, .T. ) ;
#35668=CARTESIAN_POINT ( 'NONE',  ( -24.18603102892831913, -14.68777056910904832, 20.99999999999995026 ) ) ;
#35679=CARTESIAN_POINT ( 'NONE',  ( -36.74707368630860316, -16.71203845619708517, 11.55979286843963649 ) ) ;
#35690=CARTESIAN_POINT ( 'NONE',  ( -19.36000459727014444, -2.857032334443094790, 21.00000000000056133 ) ) ;
#35692=CARTESIAN_POINT ( 'NONE',  ( 25.82310832280103341, -13.25591304976875939, 20.94377226548379767 ) ) ;
#35699=CARTESIAN_POINT ( 'NONE',  ( 34.10020663062367419, -21.93670956716277587, 11.55979286843929366 ) ) ;
#35706=ORIENTED_EDGE ( 'NONE', *, *, #6558, .T. ) ;
#35715=CARTESIAN_POINT ( 'NONE',  ( -39.48531003256149319, -11.24999992065011156, 11.00000000000000000 ) ) ;
#35746=EDGE_CURVE ( 'NONE', #28188, #4088, #36710, .T. ) ;
#35753=CARTESIAN_POINT ( 'NONE',  ( 4.583318357746482441, 36.10598097934258277, 17.92354375535250810 ) ) ;
#35763=CARTESIAN_POINT ( 'NONE',  ( -6.143904198944369455, -13.77689918168226413, 20.99999999999999645 ) ) ;
#35772=CARTESIAN_POINT ( 'NONE',  ( -15.48695972777900742, -26.74878859331914072, 16.30093088680190405 ) ) ;
#35787=CARTESIAN_POINT ( 'NONE',  ( -31.59094081668067844, -24.64165453824189100, 11.00000000000001776 ) ) ;
#35793=CARTESIAN_POINT ( 'NONE',  ( 36.26963650278469231, -7.248637393400325202, 14.53008259254015044 ) ) ;
#35795=CARTESIAN_POINT ( 'NONE',  ( 14.44241962112810285, 32.29667252612951245, 13.92931973827809600 ) ) ;
#35797=CARTESIAN_POINT ( 'NONE',  ( 10.35515495761407756, -25.90830221531241406, 15.72805884748740546 ) ) ;
#35799=CARTESIAN_POINT ( 'NONE',  ( -7.962467718762158420, 24.71319220551421481, 20.69868183039781329 ) ) ;
#35806=CARTESIAN_POINT ( 'NONE',  ( 18.38177052346872387, 3.916595739918349750, 20.50957957746022586 ) ) ;
#35815=CARTESIAN_POINT ( 'NONE',  ( -30.54456991890724638, -14.74984208377938621, 19.66345542862526230 ) ) ;
#35831=ORIENTED_EDGE ( 'NONE', *, *, #2684, .T. ) ;
#35834=CARTESIAN_POINT ( 'NONE',  ( -23.09341953181386131, -31.04079623447002234, 22.99999999999905853 ) ) ;
#35838=CARTESIAN_POINT ( 'NONE',  ( 27.60461630348735440, -20.46464247653215551, 19.27171037444157875 ) ) ;
#35863=CARTESIAN_POINT ( 'NONE',  ( -24.69586183797187218, -8.725643957992190280, 20.99999999999999645 ) ) ;
#35876=CARTESIAN_POINT ( 'NONE',  ( -36.04785107591563786, -18.56329043283760072, 10.99999999999982592 ) ) ;
#35889=CARTESIAN_POINT ( 'NONE',  ( -4.817371740575532080, 23.83900317890012843, 20.99999999999999645 ) ) ;
#35891=CARTESIAN_POINT ( 'NONE',  ( 25.95165700074904080, -9.707988825433883306, 20.94377226548378346 ) ) ;
#35922=CARTESIAN_POINT ( 'NONE',  ( -20.91708001959888108, -16.07177359997633559, 23.00000000000000000 ) ) ;
#35929=COLOUR_RGB ( '', 0.66274510, 0.83137255, 0.94901961) ;
#35950=CARTESIAN_POINT ( 'NONE',  ( 18.74997338759060028, -3.362744936764432868, 21.00000000000000000 ) ) ;
#35952=CARTESIAN_POINT ( 'NONE',  ( 11.36267260525735878, 30.20759924275323982, 18.42518152272109333 ) ) ;
#35959=CARTESIAN_POINT ( 'NONE',  ( -0.5459530983554620187, 27.50006522574757284, 23.00000000000000355 ) ) ;
#35974=CARTESIAN_POINT ( 'NONE',  ( -33.26300037445958679, -0.3730773600921533650, 13.92931973827787573 ) ) ;
#35997=CARTESIAN_POINT ( 'NONE',  ( 35.65094714180980162, -16.36533849799540263, 15.13084544680208765 ) ) ;
#36000=CARTESIAN_POINT ( 'NONE',  ( -7.110004120643877989, 37.89265721834145495, 15.13084544680205923 ) ) ;
#36001=CARTESIAN_POINT ( 'NONE',  ( -11.18737074829503797, -21.01894785647694519, 19.66345542862620732 ) ) ;
#36003=CARTESIAN_POINT ( 'NONE',  ( 6.606253895085748340, 26.00827916197615863, 20.82122704794080548 ) ) ;
#36011=CARTESIAN_POINT ( 'NONE',  ( 23.05386822411319159, -7.747535282638377652, 21.00000000000000000 ) ) ;
#36022=CARTESIAN_POINT ( 'NONE',  ( -31.21198460772095018, -5.568619476415831215, 18.87996532025784902 ) ) ;
#36039=CARTESIAN_POINT ( 'NONE',  ( -33.75875814100331951, 2.759858869446534246, 11.00000000000000000 ) ) ;
#36044=CARTESIAN_POINT ( 'NONE',  ( 19.02196449790080024, -24.34812345384549914, 18.87996532025784546 ) ) ;
#36052=CARTESIAN_POINT ( 'NONE',  ( -18.23649648353780961, -16.09146789626143814, 20.99999999999999645 ) ) ;
#36056=EDGE_LOOP ( 'NONE', ( #30924, #27381, #34381, #837, #1430 ) ) ;
#36062=CARTESIAN_POINT ( 'NONE',  ( 14.48927117870126757, -30.61587158504672246, 23.00000000000000355 ) ) ;
#36064=CARTESIAN_POINT ( 'NONE',  ( 5.067385705950949948, -26.57793081542402547, 12.73282698324853257 ) ) ;
#36067=CARTESIAN_POINT ( 'NONE',  ( -24.44578022397290695, -10.62045233751050866, 20.99999999999999645 ) ) ;
#36071=ORIENTED_EDGE ( 'NONE', *, *, #20103, .T. ) ;
#36078=CARTESIAN_POINT ( 'NONE',  ( -37.09709568333393293, -7.051483854460517620, 11.55979286843891529 ) ) ;
#36096=CARTESIAN_POINT ( 'NONE',  ( 25.30804003627885024, -11.14301119665278783, 20.99999999999999645 ) ) ;
#36120=CARTESIAN_POINT ( 'NONE',  ( -19.26948696230207858, 27.85601271560029701, 3.000000000000000000 ) ) ;
#36153=SURFACE_SIDE_STYLE ('',( #36549 ) ) ;
#36172=CARTESIAN_POINT ( 'NONE',  ( -36.73707435953562594, -10.93158220173930673, 14.53008259254087875 ) ) ;
#36187=CARTESIAN_POINT ( 'NONE',  ( -20.41099665934841312, -29.27811314928202080, 11.00000000000014211 ) ) ;
#36196=CARTESIAN_POINT ( 'NONE',  ( 36.05338440271408018, -10.94427667939843651, 15.72805884748937011 ) ) ;
#36198=CARTESIAN_POINT ( 'NONE',  ( 7.360725290688645117, 38.43561981343065526, 13.92931973827796632 ) ) ;
#36201=CARTESIAN_POINT ( 'NONE',  ( 15.48695972778119945, -26.74878859331994718, 16.30093088680190405 ) ) ;
#36205=CARTESIAN_POINT ( 'NONE',  ( -1.610977985363139187, 29.80447555512211011, 20.82122704794079482 ) ) ;
#36213=CARTESIAN_POINT ( 'NONE',  ( 28.25018339771033027, -2.647087534805522946, 19.27171037444156454 ) ) ;
#36215=CARTESIAN_POINT ( 'NONE',  ( 1.947644445291253357, 40.50000000000005684, 11.00000000000000178 ) ) ;
#36225=CARTESIAN_POINT ( 'NONE',  ( -31.19396690150113471, -3.926129315323696467, 18.42518152272069898 ) ) ;
#36229=VERTEX_POINT ( 'NONE', #22763 ) ;
#36232=AXIS2_PLACEMENT_3D ( 'NONE', #15304, #27691, #39689 ) ;
#36250=CARTESIAN_POINT ( 'NONE',  ( 31.78757023779201774, -12.37085478034622454, 19.27171037444154678 ) ) ;
#36257=CARTESIAN_POINT ( 'NONE',  ( -37.37248716976025520, -8.922526051835991012, 10.99999999999990941 ) ) ;
#36270=CARTESIAN_POINT ( 'NONE',  ( 10.15481549915635640, -27.08512292515340647, 13.32518128616567310 ) ) ;
#36273=CARTESIAN_POINT ( 'NONE',  ( -23.79772124597074523, -17.36195373897575678, 20.82122704794079482 ) ) ;
#36283=CARTESIAN_POINT ( 'NONE',  ( -18.84564290660895836, -29.34375446593489656, 11.00000000000029132 ) ) ;
#36292=CARTESIAN_POINT ( 'NONE',  ( 6.471564538981485981, 17.88766432731502931, 23.00000000000000355 ) ) ;
#36299=CARTESIAN_POINT ( 'NONE',  ( 21.62094419769710285, -18.41873747673067641, 20.82122704794092627 ) ) ;
#36310=CARTESIAN_POINT ( 'NONE',  ( 14.97058623676931255, 26.66112013780996648, 16.87380292611441135 ) ) ;
#36321=CARTESIAN_POINT ( 'NONE',  ( 9.762586613238328326, -29.39641002289260285, 10.99999999999999822 ) ) ;
#36337=CARTESIAN_POINT ( 'NONE',  ( -19.62624412895475245, 17.27415994119605003, 15.13084544680118704 ) ) ;
#36366=CARTESIAN_POINT ( 'NONE',  ( 16.23042486173695309, -23.86708630543283505, 18.87996532025784546 ) ) ;
#36392=CARTESIAN_POINT ( 'NONE',  ( 18.85272453233919165, -29.14374917747379357, 12.73282698324887896 ) ) ;
#36394=CARTESIAN_POINT ( 'NONE',  ( -16.30840571581334686, 28.99314201041626404, 13.92931973827731618 ) ) ;
#36399=CARTESIAN_POINT ( 'NONE',  ( -7.341573453990910991, 26.39883817588575354, 20.69868183039782394 ) ) ;
#36406=CARTESIAN_POINT ( 'NONE',  ( 23.61737546510196850, -7.194424252577104717, 21.00000000000000000 ) ) ;
#36416=CARTESIAN_POINT ( 'NONE',  ( -17.70478766477605248, -23.47393717365530108, 19.27171037444159296 ) ) ;
#36435=CARTESIAN_POINT ( 'NONE',  ( -36.53988293556027145, -0.5802930328939031046, 11.00000000000000000 ) ) ;
#36441=CARTESIAN_POINT ( 'NONE',  ( 33.29356883319506721, -10.99541271083377403, 18.42518152272108622 ) ) ;
#36457=DIRECTION ( 'NONE',  ( -0.000000000000000000, -0.000000000000000000, -1.000000000000000000 ) ) ;
#36462=CARTESIAN_POINT ( 'NONE',  ( 4.262995805457294793E-14, -26.57793081542402547, 12.73282698324853257 ) ) ;
#36465=CARTESIAN_POINT ( 'NONE',  ( -25.56674216509407671, -13.93466449336376023, 20.94377226548387583 ) ) ;
#36479=CARTESIAN_POINT ( 'NONE',  ( -22.38472516250436328, -15.35952186208485593, 21.00000000000000000 ) ) ;
#36492=CARTESIAN_POINT ( 'NONE',  ( 26.13185812888305293, -11.12779425996326133, 20.94377226548378346 ) ) ;
#36509=CARTESIAN_POINT ( 'NONE',  ( 9.762440214479946476, -29.39637225272704057, 11.00000000000000000 ) ) ;
#36532=CARTESIAN_POINT ( 'NONE',  ( -23.18947492591163240, 13.38844959084118535, 11.00000000000000000 ) ) ;
#36549=SURFACE_STYLE_FILL_AREA ( #39593 ) ;
#36589=CARTESIAN_POINT ( 'NONE',  ( 37.17935095643323962, -12.86265498539263064, 13.32518128616619357 ) ) ;
#36591=CARTESIAN_POINT ( 'NONE',  ( -16.81416712651214596, 27.17354907310119572, 13.92931973827808889 ) ) ;
#36592=CARTESIAN_POINT ( 'NONE',  ( 17.62780868050938565, -18.45076755199376706, 20.82122704794079837 ) ) ;
#36594=CARTESIAN_POINT ( 'NONE',  ( -8.207473342610091649, 28.06734471880738369, 20.25080042701566541 ) ) ;
#36606=CARTESIAN_POINT ( 'NONE',  ( 19.72827082054694259, 4.852702923338547691, 19.99202127657091665 ) ) ;
#36616=CARTESIAN_POINT ( 'NONE',  ( -17.49459433713212064, -24.91609123032629469, 18.42518152272109333 ) ) ;
#36642=CARTESIAN_POINT ( 'NONE',  ( 33.53288488731369910, -7.900844017966136335, 17.92354375535250810 ) ) ;
#36648=CARTESIAN_POINT ( 'NONE',  ( -14.98890121934590347, -28.67928442654175569, 11.55979286843935050 ) ) ;
#36662=CARTESIAN_POINT ( 'NONE',  ( -10.13173764377114239, -27.22067640326290672, 12.73282698326143425 ) ) ;
#36665=CARTESIAN_POINT ( 'NONE',  ( -24.39151161285703040, -15.73551128733878102, 20.94377226548378701 ) ) ;
#36696=CARTESIAN_POINT ( 'NONE',  ( 26.53285121770567301, -6.841429973034632184, 20.69868183039801224 ) ) ;
#36702=EDGE_CURVE ( 'NONE', #34372, #8296, #6252, .T. ) ;
#36710=CIRCLE ( 'NONE', #5556, 17.99999999999993250 ) ;
#36713=CARTESIAN_POINT ( 'NONE',  ( 12.28720923547795429, -14.55658080553756406, 23.00000000000000000 ) ) ;
#36723=CARTESIAN_POINT ( 'NONE',  ( 32.09165771328607519, 1.123514972292635861, 13.32518128616608521 ) ) ;
#36738=CARTESIAN_POINT ( 'NONE',  ( -18.37899676825032103, 22.33688965561464812, 13.32518128618448650 ) ) ;
#36754=( LENGTH_UNIT ( ) NAMED_UNIT ( * ) SI_UNIT ( .MILLI., .METRE. ) );
#36756=CARTESIAN_POINT ( 'NONE',  ( -37.48531001978128074, -11.24999991186452775, 11.00000000000002309 ) ) ;
#36757=CARTESIAN_POINT ( 'NONE',  ( 3.459945280434955972, 26.15050560728434448, 23.00000000000000355 ) ) ;
#36788=CARTESIAN_POINT ( 'NONE',  ( 1.926143243141009931, 40.30103163374183595, 12.73282698324853435 ) ) ;
#36789=CARTESIAN_POINT ( 'NONE',  ( -17.83459896180957927, -17.64923967996706367, 20.94377226548378346 ) ) ;
#36791=CARTESIAN_POINT ( 'NONE',  ( -7.531283639252405848, 27.60866748444384555, 20.50957957746029692 ) ) ;
#36798=AXIS2_PLACEMENT_3D ( 'NONE', #32033, #23090, #7443 ) ;
#36804=EDGE_CURVE ( 'NONE', #21291, #30744, #14434, .T. ) ;
#36812=CARTESIAN_POINT ( 'NONE',  ( -26.16909114927327451, -23.33537003677659527, 18.42518152272073095 ) ) ;
#36825=CARTESIAN_POINT ( 'NONE',  ( 33.75875814100314187, 2.759858869446414786, 11.00000000000000000 ) ) ;
#36829=CARTESIAN_POINT ( 'NONE',  ( 23.05386822411318803, -7.747535282638377652, 23.00000000000000000 ) ) ;
#36837=CARTESIAN_POINT ( 'NONE',  ( 27.44755207257203367, -22.53416897284666121, 18.42518152272072385 ) ) ;
#36860=CARTESIAN_POINT ( 'NONE',  ( -15.20016916873736079, -27.86040092368267551, 14.53008259254011136 ) ) ;
#36863=CARTESIAN_POINT ( 'NONE',  ( -19.22069824708770014, -18.72532366025136596, 20.82122704794093337 ) ) ;
#36890=CARTESIAN_POINT ( 'NONE',  ( 27.79678266235291773, -11.09703717633714426, 20.69868183039781329 ) ) ;
#36926=CARTESIAN_POINT ( 'NONE',  ( -31.94006737154538200, 0.9747213384856526774, 13.92931973827809067 ) ) ;
#36936=CARTESIAN_POINT ( 'NONE',  ( -18.69515074623005901, 22.45407711376556747, 11.55979286846285703 ) ) ;
#36950=EDGE_CURVE ( 'NONE', #32321, #17014, #32894, .T. ) ;
#36964=CARTESIAN_POINT ( 'NONE',  ( 4.672335726382788046, 24.36080358023179571, 23.00000000000000000 ) ) ;
#36991=CARTESIAN_POINT ( 'NONE',  ( -17.01882136418224789, 27.23043334310857233, 13.32518128616608877 ) ) ;
#36992=CARTESIAN_POINT ( 'NONE',  ( -6.008588623656293315, -15.38567963534269900, 20.94377226548378701 ) ) ;
#36995=CARTESIAN_POINT ( 'NONE',  ( 4.183427099969757812, 31.55590659971980472, 20.25080042701566185 ) ) ;
#37012=CARTESIAN_POINT ( 'NONE',  ( -33.46894051142380277, -4.475137156698075991, 16.87380292611441490 ) ) ;
#37036=CARTESIAN_POINT ( 'NONE',  ( 23.43324262027548599, -8.134040356058108046, 20.99999999999999645 ) ) ;
#37037=CARTESIAN_POINT ( 'NONE',  ( 33.23893881994253263, -12.50319288011949936, 18.42518152272107912 ) ) ;
#37047=CARTESIAN_POINT ( 'NONE',  ( 32.09165771328606809, 1.123514972292636083, 13.32518128616608877 ) ) ;
#37059=CARTESIAN_POINT ( 'NONE',  ( -19.90456025098508164, -17.02442174103788020, 20.99999999999999645 ) ) ;
#37085=CARTESIAN_POINT ( 'NONE',  ( -26.46527715132802783, -30.05405011173883167, 10.99999999999999822 ) ) ;
#37087=CARTESIAN_POINT ( 'NONE',  ( 27.41073561697711369, -13.75826678482997423, 20.69868183039782750 ) ) ;
#37096=CARTESIAN_POINT ( 'NONE',  ( -19.26948696230206082, 27.85601271560033965, 22.99999999999999645 ) ) ;
#37107=SURFACE_SIDE_STYLE ('',( #14970 ) ) ;
#37122=CARTESIAN_POINT ( 'NONE',  ( -36.26963650278440099, -7.248637393401118345, 14.53008259253934220 ) ) ;
#37132=CARTESIAN_POINT ( 'NONE',  ( -18.50792845154007438, 22.38468038563317108, 12.73282698326878304 ) ) ;
#37135=CARTESIAN_POINT ( 'NONE',  ( 23.20071485358947783, -14.64063822049746477, 23.00000000000000711 ) ) ;
#37143=CARTESIAN_POINT ( 'NONE',  ( 22.48079666814720667, 18.61591633950847324, 11.00000000000000000 ) ) ;
#37145=DIRECTION ( 'NONE',  ( -0.000000000000000000, -0.000000000000000000, -1.000000000000000000 ) ) ;
#37158=CARTESIAN_POINT ( 'NONE',  ( -4.817371740575545402, 23.83900317890010001, 23.00000000000000000 ) ) ;
#37190=CARTESIAN_POINT ( 'NONE',  ( -5.682704777077058900, 39.36960561607953935, 12.73282698324852902 ) ) ;
#37191=CARTESIAN_POINT ( 'NONE',  ( -11.87696897075269042, -16.96707895830268598, 20.82122704794084456 ) ) ;
#37193=CARTESIAN_POINT ( 'NONE',  ( -2.325696902088870921, 33.04389473401317900, 19.99202127657102679 ) ) ;
#37213=CARTESIAN_POINT ( 'NONE',  ( -31.65150718622412995, -20.14649908112938803, 17.42190598798354628 ) ) ;
#37238=CARTESIAN_POINT ( 'NONE',  ( 32.46232039045683138, -18.74212941594987214, 17.42190598798392642 ) ) ;
#37242=CARTESIAN_POINT ( 'NONE',  ( 4.817371740575538297, 23.83900317890011067, 20.99999999999999645 ) ) ;
#37258=CARTESIAN_POINT ( 'NONE',  ( -28.60147806546170202, -12.08038679647151348, 20.50957957746030758 ) ) ;
#37259=CYLINDRICAL_SURFACE ( 'NONE', #39940, 19.99999999999993250 ) ;
#37268=ORIENTED_EDGE ( 'NONE', *, *, #29419, .F. ) ;
#37283=CARTESIAN_POINT ( 'NONE',  ( -34.03019007953001562, -25.06168574969261797, 11.00000000000000000 ) ) ;
#37284=CARTESIAN_POINT ( 'NONE',  ( 27.31307666897629360, -8.451821295062190487, 20.69868183039763565 ) ) ;
#37292=CARTESIAN_POINT ( 'NONE',  ( -30.33922525721619223, 6.243664897686377557, 11.00000000000000000 ) ) ;
#37301=( NAMED_UNIT ( * ) PLANE_ANGLE_UNIT ( ) SI_UNIT ( $, .RADIAN. ) );
#37319=CARTESIAN_POINT ( 'NONE',  ( -35.97875289183299685, -7.317948980264791459, 15.13084544680133270 ) ) ;
#37329=CARTESIAN_POINT ( 'NONE',  ( -27.14644468510207531, -3.730463242937111179, 19.99202127657103389 ) ) ;
#37333=CARTESIAN_POINT ( 'NONE',  ( 18.23649648353767461, -16.09146789626181118, 23.00000000000000000 ) ) ;
#37338=CARTESIAN_POINT ( 'NONE',  ( 22.63195743522303260, -28.51917808483202066, 13.92931973827781711 ) ) ;
#37357=CARTESIAN_POINT ( 'NONE',  ( 10.37659644360199707, 39.73422260060728206, 23.00000000000000000 ) ) ;
#37380=CARTESIAN_POINT ( 'NONE',  ( 75.15099915297797395, 43.38844959084117647, 23.00000000000000000 ) ) ;
#37388=CARTESIAN_POINT ( 'NONE',  ( -16.63496159152044385, 29.12310921430476185, 12.73282698324768880 ) ) ;
#37390=CARTESIAN_POINT ( 'NONE',  ( -32.33143948541797386, 1.358872982501901472, 23.00000000000000000 ) ) ;
#37391=CARTESIAN_POINT ( 'NONE',  ( -10.90978760418654758, 28.29414058874172255, 19.27171037444159296 ) ) ;
#37410=CARTESIAN_POINT ( 'NONE',  ( -30.60828605274471670, -21.42068866018134088, 17.42190598798391221 ) ) ;
#37435=CARTESIAN_POINT ( 'NONE',  ( 33.78274305024982738, -17.56282548559263290, 16.87380292611442556 ) ) ;
#37439=CARTESIAN_POINT ( 'NONE',  ( 3.456468065139975732, 26.15323006594241306, 20.99999999999999645 ) ) ;
#37443=( BOUNDED_SURFACE ( )  B_SPLINE_SURFACE ( 2, 3, ( 
 ( #17161, #6976, #35034, #29536, #903, #26488, #4140, #13485, #13687, #1711, #38477, #38276, #13280, #32184, #19997, #4346, #16752, #29132 ),
 ( #1305, #26076, #7592, #32394, #4550, #16952, #11254, #30141, #20404, #29738, #8199, #5750, #7993, #32799, #35834, #2514, #17765, #4956 ),
 ( #36039, #39076, #36435, #5352, #14295, #11850, #23841, #15093, #21194, #30343, #2115, #17362, #20998, #1917, #14495, #24239, #8806, #26687 ) ),
 .UNSPECIFIED., .F., .F., .T. ) 
 B_SPLINE_SURFACE_WITH_KNOTS ( ( 3, 3 ),
 ( 4, 2, 2, 2, 2, 2, 2, 2, 4 ),
 ( 0.000000000000000000, 1.000000000000000000 ),
 ( 2.365504664328351048, 2.690426355543287240, 3.015348046758223433, 3.340269737973159181, 3.665191429188095373, 3.990113120403031566, 4.315034811617967314, 4.639956502832903951, 4.964878194047839699 ),
 .UNSPECIFIED. ) 
 GEOMETRIC_REPRESENTATION_ITEM ( )  RATIONAL_B_SPLINE_SURFACE ( (
 ( 1.000000000000000000, 1.000000000000000000, 1.000000000000000000, 1.000000000000000000, 1.000000000000000000, 1.000000000000000000, 1.000000000000000000, 1.000000000000000000, 1.000000000000000000, 1.000000000000000000, 1.000000000000000000, 1.000000000000000000, 1.000000000000000000, 1.000000000000000000, 1.000000000000000000, 1.000000000000000000, 1.000000000000000000, 1.000000000000000000),
 ( 0.7071067811865475727, 0.7071067811865475727, 0.7071067811865474617, 0.7071067811865474617, 0.7071067811865474617, 0.7071067811865474617, 0.7071067811865474617, 0.7071067811865474617, 0.7071067811865476838, 0.7071067811865476838, 0.7071067811865475727, 0.7071067811865475727, 0.7071067811865475727, 0.7071067811865475727, 0.7071067811865474617, 0.7071067811865474617, 0.7071067811865474617, 0.7071067811865474617),
 ( 1.000000000000000000, 1.000000000000000000, 1.000000000000000000, 1.000000000000000000, 1.000000000000000000, 1.000000000000000000, 1.000000000000000000, 1.000000000000000000, 1.000000000000000000, 1.000000000000000000, 1.000000000000000000, 1.000000000000000000, 1.000000000000000000, 1.000000000000000000, 1.000000000000000000, 1.000000000000000000, 1.000000000000000000, 1.000000000000000000) ) ) 
 REPRESENTATION_ITEM ( '' )  SURFACE ( )  );
#37447=CARTESIAN_POINT ( 'NONE',  ( 25.01795332078024359, 8.530037020299428008, 14.53008259254034407 ) ) ;
#37459=CARTESIAN_POINT ( 'NONE',  ( -19.16156146161704399, -20.39791387780022092, 20.50957957746050653 ) ) ;
#37485=CARTESIAN_POINT ( 'NONE',  ( 26.92296394334098153, -7.646625634048409559, 20.69868183039782394 ) ) ;
#37495=CARTESIAN_POINT ( 'NONE',  ( -15.00309677617818771, 1.567672476163657125, 23.00000000000000000 ) ) ;
#37498=EDGE_CURVE ( 'NONE', #8563, #12781, #29733, .T. ) ;
#37518=CARTESIAN_POINT ( 'NONE',  ( -36.80210562958730236, -14.73639196410522345, 13.32518128616608699 ) ) ;
#37531=CARTESIAN_POINT ( 'NONE',  ( -29.73172958077111971, -1.192874570362842057, 17.92354375535250810 ) ) ;
#37535=CARTESIAN_POINT ( 'NONE',  ( 24.22334197529778521, -9.561459978639769375, 22.99999999999999645 ) ) ;
#37536=ADVANCED_FACE ( 'NONE', ( #14290 ), #2919, .T. ) ;
#37539=CARTESIAN_POINT ( 'NONE',  ( 35.38210723591825513, -3.548218742174890750, 13.32518128616608344 ) ) ;
#37548=CARTESIAN_POINT ( 'NONE',  ( 3.863783140547853712E-14, -86.77689918168233874, 23.00000000000000000 ) ) ;
#37559=CARTESIAN_POINT ( 'NONE',  ( 15.33540832684151134, 35.51988609203956315, 11.00000000000000000 ) ) ;
#37586=ORIENTED_EDGE ( 'NONE', *, *, #12511, .F. ) ;
#37594=CARTESIAN_POINT ( 'NONE',  ( -1.450054154221040505E-13, 40.30103163374182174, 12.73282698324853257 ) ) ;
#37598=CARTESIAN_POINT ( 'NONE',  ( 2.823200210931128940, 35.29864485453420286, 18.87996532025784902 ) ) ;
#37611=CARTESIAN_POINT ( 'NONE',  ( -3.833852081710639848, 25.75497152300896886, 20.99999999999999645 ) ) ;
#37616=CARTESIAN_POINT ( 'NONE',  ( -32.46232039045670348, -18.74212941594990767, 17.42190598798392642 ) ) ;
#37637=CARTESIAN_POINT ( 'NONE',  ( 23.54493052986452284, -14.21898406159493966, 20.99999999999999645 ) ) ;
#37638=CARTESIAN_POINT ( 'NONE',  ( 33.46894051142319881, -4.475137156697218899, 16.87380292611441845 ) ) ;
#37640=AXIS2_PLACEMENT_3D ( 'NONE', #34642, #35244, #10057 ) ;
#37642=CARTESIAN_POINT ( 'NONE',  ( -0.6269669233417689558, 28.28960257232501974, 20.99999999999998934 ) ) ;
#37647=CARTESIAN_POINT ( 'NONE',  ( 20.66414367075948277, 17.76245163070629829, 10.99999999999897859 ) ) ;
#37655=CARTESIAN_POINT ( 'NONE',  ( -28.63766977552542770, -11.08150102882335375, 20.50957957746073390 ) ) ;
#37659=CARTESIAN_POINT ( 'NONE',  ( -32.33143948541797386, 1.358872982501901472, 2.999999999999999112 ) ) ;
#37682=CARTESIAN_POINT ( 'NONE',  ( 28.41077021456689522, -6.925791943819275431, 20.25080042701566541 ) ) ;
#37708=CARTESIAN_POINT ( 'NONE',  ( 34.83525826321754693, -1.648928274806292116, 10.99999999999991829 ) ) ;
#37718=CARTESIAN_POINT ( 'NONE',  ( -32.69891748962417921, -23.33280782878161830, 12.73282698324838691 ) ) ;
#37725=CARTESIAN_POINT ( 'NONE',  ( -12.75386240996836484, 29.27369326522011050, 17.92354375535251876 ) ) ;
#37729=CARTESIAN_POINT ( 'NONE',  ( -30.57450045107345460, -0.3656520783135125963, 16.87380292611441845 ) ) ;
#37732=CARTESIAN_POINT ( 'NONE',  ( 19.26948696230199687, 27.85601271560034675, 11.00000000000000000 ) ) ;
#37736=CARTESIAN_POINT ( 'NONE',  ( 34.59909889755208923, -19.97579906221994506, 13.92931973827808712 ) ) ;
#37768=CARTESIAN_POINT ( 'NONE',  ( 75.15099915297797395, 43.38844959084117647, 2.999999999999999112 ) ) ;
#37784=CARTESIAN_POINT ( 'NONE',  ( -10.89111091687340682, 36.83121428896946981, 11.55979286843934339 ) ) ;
#37787=CARTESIAN_POINT ( 'NONE',  ( -11.83264664767379948, 25.78892025138465272, 19.27171037444156454 ) ) ;
#37805=CARTESIAN_POINT ( 'NONE',  ( -31.72870305971091298, -3.591698066951732216, 17.92354375535209954 ) ) ;
#37811=ORIENTED_EDGE ( 'NONE', *, *, #30745, .F. ) ;
#37826=CARTESIAN_POINT ( 'NONE',  ( 28.49608467062326156, -24.01994641533507036, 16.87380292611404897 ) ) ;
#37832=CARTESIAN_POINT ( 'NONE',  ( -5.578133564216450679, 24.05045924978193739, 20.99999999999999645 ) ) ;
#37838=CARTESIAN_POINT ( 'NONE',  ( 20.60789226802129548, 17.73598670052725623, 12.14047268033019300 ) ) ;
#37846=CARTESIAN_POINT ( 'NONE',  ( -21.85869495254141270, -19.21667513322701382, 20.69868183039799447 ) ) ;
#37860=ORIENTED_EDGE ( 'NONE', *, *, #4683, .F. ) ;
#37874=CARTESIAN_POINT ( 'NONE',  ( 26.58217467610746354, -19.30423083005467078, 19.99202127657103389 ) ) ;
#37908=PRODUCT ( 'Protective Travel Cap', 'Protective Travel Cap', '', ( #13191 ) ) ;
#37912=CARTESIAN_POINT ( 'NONE',  ( -36.47501240582165849, -5.175470059597266470, 12.14047268033136362 ) ) ;
#37920=CARTESIAN_POINT ( 'NONE',  ( 19.26948696230199687, 27.85601271560034675, 11.00000000000000000 ) ) ;
#37921=CARTESIAN_POINT ( 'NONE',  ( -6.553841457909052259, 36.68830644081907622, 16.87380292611438648 ) ) ;
#37925=CARTESIAN_POINT ( 'NONE',  ( -16.81914744117433003, 21.75867863388409873, 16.30093088680929370 ) ) ;
#37933=CARTESIAN_POINT ( 'NONE',  ( 32.28722999652137560, 1.315479119631175697, 12.14047268033097460 ) ) ;
#37955=CARTESIAN_POINT ( 'NONE',  ( -10.37659644360344835, 39.73422260060537781, 22.99999999999811351 ) ) ;
#37967=CARTESIAN_POINT ( 'NONE',  ( -34.66483173867272427, 1.836754817265617623, 11.00000000000000000 ) ) ;
#37987=CARTESIAN_POINT ( 'NONE',  ( 10.89111091687315813, 36.83121428896965455, 11.55979286843934695 ) ) ;
#37990=CARTESIAN_POINT ( 'NONE',  ( 5.496198527381090493, 34.39821714758473803, 18.87996532025784902 ) ) ;
#37995=CARTESIAN_POINT ( 'NONE',  ( 4.817371740575539185, 23.83900317890011422, 23.00000000000000000 ) ) ;
#38008=CARTESIAN_POINT ( 'NONE',  ( -20.64393337882609103, -27.21432092515239631, 16.30093088680190405 ) ) ;
#38028=CARTESIAN_POINT ( 'NONE',  ( 15.37000524124839274, -27.20210912714561857, 15.72805884748939498 ) ) ;
#38031=CARTESIAN_POINT ( 'NONE',  ( 1.824109939551872506, 39.35700678546974274, 15.13084544680213916 ) ) ;
#38034=CARTESIAN_POINT ( 'NONE',  ( -5.410216727984581198, 24.65457866814584165, 20.99999999999995026 ) ) ;
#38042=CARTESIAN_POINT ( 'NONE',  ( 26.46356280838283936, 3.031871643931095317, 17.42190598799536616 ) ) ;
#38049=CARTESIAN_POINT ( 'NONE',  ( -28.40703083259910855, -13.04618529600556442, 20.50957957746029692 ) ) ;
#38067=ORIENTED_EDGE ( 'NONE', *, *, #19596, .T. ) ;
#38074=CARTESIAN_POINT ( 'NONE',  ( 21.27405569407545372, -21.06385914081313970, 20.25080042701566896 ) ) ;
#38111=CARTESIAN_POINT ( 'NONE',  ( -22.63199090478729403, -28.51917565629995721, 13.92931973827765901 ) ) ;
#38118=CARTESIAN_POINT ( 'NONE',  ( 11.49020332972282432, 32.25361022348394613, 17.42190598798394774 ) ) ;
#38123=CARTESIAN_POINT ( 'NONE',  ( -20.38546294303667139, 5.309590202434897321, 19.66345542862530138 ) ) ;
#38130=CARTESIAN_POINT ( 'NONE',  ( 36.90241796781165107, -7.097865958169077061, 12.73282698324860007 ) ) ;
#38152=CARTESIAN_POINT ( 'NONE',  ( -17.76739295965093390, 31.93461338995377830, 22.99999999999999289 ) ) ;
#38166=CARTESIAN_POINT ( 'NONE',  ( -19.48557158514998022, -11.24999999999982414, 2.999999999999999112 ) ) ;
#38186=CARTESIAN_POINT ( 'NONE',  ( -17.34253826607193361, 27.32041144404004385, 11.55979286843934872 ) ) ;
#38190=CARTESIAN_POINT ( 'NONE',  ( 9.417371715876635463, 30.49428522466168090, 19.27171037444157875 ) ) ;
#38193=DIRECTION ( 'NONE',  ( 1.000000000000000000, 0.000000000000000000, 0.000000000000000000 ) ) ;
#38205=CARTESIAN_POINT ( 'NONE',  ( 15.12590024503159292, -28.14827041158713072, 13.92931973827808712 ) ) ;
#38213=CARTESIAN_POINT ( 'NONE',  ( -35.17699530642141781, -14.40920341950810268, 16.30093088680190050 ) ) ;
#38235=CARTESIAN_POINT ( 'NONE',  ( 35.04992612853292400, -12.66836002548405382, 16.87380292611442201 ) ) ;
#38238=CARTESIAN_POINT ( 'NONE',  ( 5.381339405376090568, 38.47497618056186042, 15.13084544680213561 ) ) ;
#38240=CARTESIAN_POINT ( 'NONE',  ( -3.428976547227685856, 28.19475011768389905, 20.94377226548358450 ) ) ;
#38245=B_SPLINE_SURFACE_WITH_KNOTS ( 'NONE', 3, 3, ( 
 ( #5961, #34203, #37647, #12858, #16111, #9817, #28497 ),
 ( #22194, #34597, #9623, #6750, #19154, #670, #75 ),
 ( #25439, #31546, #37838, #18366, #3710, #27899, #15708 ),
 ( #24852, #6165, #10013, #30761, #2922, #15310, #27696 ),
 ( #12265, #12459, #18764, #40088, #22003, #24653, #37047 ),
 ( #31153, #9217, #34402, #21602, #3317, #34007, #18567 ),
 ( #28096, #275, #30952, #12660, #37447, #10211, #7766 ),
 ( #31750, #35608, #32156, #3912, #31944, #35005, #26047 ),
 ( #20169, #1077, #38447, #4316, #35404, #16922, #23001 ),
 ( #25846, #10620, #26453, #38853, #32565, #4110, #38247 ),
 ( #11029, #35197, #10415, #4724, #13453, #16517, #1683 ),
 ( #7563, #22797, #13252, #34796, #7355, #38042, #16311 ),
 ( #26254, #28900, #28694, #17131, #19758, #38650, #16719 ),
 ( #29103, #873, #22596, #1276, #23211, #13658, #4523 ),
 ( #19964, #14060, #32364, #29306, #29506, #1478, #6946 ),
 ( #13865, #10822, #25644, #19353, #7154, #19553, #36213 ),
 ( #5126, #23413, #33373, #39247, #11427, #23811, #24011 ),
 ( #14465, #27062, #15065, #27455, #36606, #20575, #26858 ),
 ( #39841, #8378, #20776, #8772, #29906, #32971, #30518 ),
 ( #11819, #39447, #2085, #1888, #35806, #33171, #26656 ),
 ( #18129, #14873, #17532, #32768, #21164, #5322, #27258 ),
 ( #8170, #11628, #33569, #7962, #17734, #2484, #8568 ),
 ( #39646, #5719, #24207, #5516, #20968, #30111, #17930 ),
 ( #29706, #11224, #20375, #2282, #2678, #14672, #36406 ),
 ( #30314, #4926, #17332, #14267, #39046, #23615, #36011 ) ),
 .UNSPECIFIED., .F., .F., .F.,
 ( 4, 3, 3, 3, 3, 3, 3, 3, 4 ),
 ( 4, 3, 4 ),
 ( 0.000000000000000000, 0.1250000000000000000, 0.2500000000000000000, 0.3750000000000000000, 0.5000000000000000000, 0.6250000000000000000, 0.7500000000000000000, 0.8750000000000000000, 1.000000000000000000 ),
 ( 3.412702215524944904, 3.665191429188091377, 3.917680642851237405 ),
 .UNSPECIFIED. ) ;
#38247=CARTESIAN_POINT ( 'NONE',  ( 30.90861030616866856, -0.03770625498867555270, 16.30093088680190405 ) ) ;
#38255=CARTESIAN_POINT ( 'NONE',  ( -27.71565130972494728, -3.171757977841499709, 19.66345542862529072 ) ) ;
#38276=CARTESIAN_POINT ( 'NONE',  ( -22.38472516250435973, -15.35952186208485593, 23.00000000000000000 ) ) ;
#38281=CARTESIAN_POINT ( 'NONE',  ( 21.56512766274792625, -22.66165129494964958, 19.66345542862529072 ) ) ;
#38291=EDGE_LOOP ( 'NONE', ( #3876, #2250, #28065, #33352 ) ) ;
#38313=CARTESIAN_POINT ( 'NONE',  ( -33.43067318719309355, -0.2406684815417533818, 13.32518128616583475 ) ) ;
#38324=CARTESIAN_POINT ( 'NONE',  ( 13.80282919548806575, 29.83094698618029028, 16.87380292611440424 ) ) ;
#38327=CARTESIAN_POINT ( 'NONE',  ( -18.74997338764005050, -3.362744936731938417, 20.99999999999999645 ) ) ;
#38333=CARTESIAN_POINT ( 'NONE',  ( 20.78821643698954347, -29.20280246618839115, 11.55979286843934872 ) ) ;
#38360=CARTESIAN_POINT ( 'NONE',  ( -23.05386822411323422, -7.747535282638357224, 23.00000000000000000 ) ) ;
#38385=CARTESIAN_POINT ( 'NONE',  ( 15.98959510862164457, 30.99271259066415496, 10.99999999999987566 ) ) ;
#38389=CARTESIAN_POINT ( 'NONE',  ( 11.88159808435121789, 30.55960002361340955, 17.92354375535251165 ) ) ;
#38402=CARTESIAN_POINT ( 'NONE',  ( 2.109373541296217347, 27.06550157850341876, 20.99999999999999645 ) ) ;
#38407=CARTESIAN_POINT ( 'NONE',  ( -25.67968615518532971, -26.00921032235747887, 16.30093088680191116 ) ) ;
#38434=CARTESIAN_POINT ( 'NONE',  ( 31.51573171626510117, 0.5582143012859381859, 15.13084544680214094 ) ) ;
#38436=CARTESIAN_POINT ( 'NONE',  ( -1.782755275186030275, 38.97445513318768207, 15.72805884748939143 ) ) ;
#38438=CARTESIAN_POINT ( 'NONE',  ( 5.218261001347106465, -24.78318996519343997, 16.30093088680190760 ) ) ;
#38442=CARTESIAN_POINT ( 'NONE',  ( 5.143257298371474384, 25.23120666211534413, 21.00000000000000355 ) ) ;
#38447=CARTESIAN_POINT ( 'NONE',  ( 19.27886458632777789, 17.11073565397641616, 15.72805884748938432 ) ) ;
#38455=CARTESIAN_POINT ( 'NONE',  ( -29.18141975161403678, -3.595827299476843208, 19.27171037444158230 ) ) ;
#38477=CARTESIAN_POINT ( 'NONE',  ( -23.19735768193461567, -14.64350930037788068, 23.00000000000000000 ) ) ;
#38481=CARTESIAN_POINT ( 'NONE',  ( 28.78203904708371397, -16.61731799165995227, 19.99202127657103389 ) ) ;
#38494=( GEOMETRIC_REPRESENTATION_CONTEXT ( 3 ) GLOBAL_UNCERTAINTY_ASSIGNED_CONTEXT ( ( #7942 ) ) GLOBAL_UNIT_ASSIGNED_CONTEXT ( ( #36754, #17681, #30056 ) ) REPRESENTATION_CONTEXT ( 'NONE', 'WORKASPACE' ) );
#38504=CARTESIAN_POINT ( 'NONE',  ( -18.23649648353780961, -16.09146789626144169, 20.99999999999999645 ) ) ;
#38514=CARTESIAN_POINT ( 'NONE',  ( -37.58754968649139983, -10.91577297561634552, 11.00000000000031797 ) ) ;
#38523=CARTESIAN_POINT ( 'NONE',  ( -7.775297188279279403, 35.41132985342461126, 17.42190598798310930 ) ) ;
#38527=CARTESIAN_POINT ( 'NONE',  ( -7.962467718763332591, 24.71319220550997642, 20.69868183039781329 ) ) ;
#38528=VERTEX_POINT ( 'NONE', #23540 ) ;
#38533=CARTESIAN_POINT ( 'NONE',  ( 28.21696687770567280, -27.03935558029786534, 12.14047268033092841 ) ) ;
#38539=CARTESIAN_POINT ( 'NONE',  ( -9.742785792574970571, -49.01344959084108410, 23.00000000000000000 ) ) ;
#38561=CARTESIAN_POINT ( 'NONE',  ( -18.23649648353780961, -16.09146789626143814, 23.00000000000000000 ) ) ;
#38585=CARTESIAN_POINT ( 'NONE',  ( -12.44178368932704259, 35.65276919562052882, 11.00000000000005329 ) ) ;
#38590=CARTESIAN_POINT ( 'NONE',  ( 7.124477683919607784, 34.33078274761139426, 18.42518152272109333 ) ) ;
#38608=CARTESIAN_POINT ( 'NONE',  ( -35.51887168741988887, -12.71114019210525647, 16.30093088680185076 ) ) ;
#38635=CARTESIAN_POINT ( 'NONE',  ( 22.52482594781217529, -27.93079697604290246, 15.13084544680195265 ) ) ;
#38636=ORIENTED_EDGE ( 'NONE', *, *, #21322, .T. ) ;
#38637=CARTESIAN_POINT ( 'NONE',  ( -15.87271491999997863, 26.91186955879525300, 15.72805884748939498 ) ) ;
#38638=CARTESIAN_POINT ( 'NONE',  ( -10.71169154829944681, -23.81371503818770918, 17.92354375535594357 ) ) ;
#38641=CARTESIAN_POINT ( 'NONE',  ( 7.722840163546785597, 25.57530741998005652, 20.69868183039857712 ) ) ;
#38650=CARTESIAN_POINT ( 'NONE',  ( 25.97912795563643584, 2.630260520701592775, 17.92354375536424627 ) ) ;
#38659=CARTESIAN_POINT ( 'NONE',  ( -29.31961554340469078, -5.098421488388908074, 19.66345542862496742 ) ) ;
#38674=CARTESIAN_POINT ( 'NONE',  ( 24.08646667827958154, -13.28101593840524330, 23.00000000000000000 ) ) ;
#38686=CARTESIAN_POINT ( 'NONE',  ( 31.50169271651470737, -8.384983552473938673, 19.27171037444156099 ) ) ;
#38691=ADVANCED_FACE ( 'NONE', ( #3005 ), #3850, .F. ) ;
#38710=CARTESIAN_POINT ( 'NONE',  ( -22.38472516250435973, -15.35952186208485593, 21.00000000000000000 ) ) ;
#38721=CARTESIAN_POINT ( 'NONE',  ( -36.04785107591552418, -18.56329043283772151, 11.55979286843925102 ) ) ;
#38733=CARTESIAN_POINT ( 'NONE',  ( -23.05386822411323422, -7.747535282638357224, 20.99999999999999645 ) ) ;
#38735=CARTESIAN_POINT ( 'NONE',  ( 20.52988321362932922, -16.97904867242824523, 20.99999999999999645 ) ) ;
#38739=CARTESIAN_POINT ( 'NONE',  ( 35.62872793493669832, -3.428732413881706798, 12.14047268033096927 ) ) ;
#38750=DIRECTION ( 'NONE',  ( -0.000000000000000000, -0.000000000000000000, -1.000000000000000000 ) ) ;
#38763=CARTESIAN_POINT ( 'NONE',  ( -19.30269652822713056, -16.27647962203388943, 23.00000000000001066 ) ) ;
#38792=CARTESIAN_POINT ( 'NONE',  ( 12.75384976115305236, 29.27371191231734571, 17.92354375535250455 ) ) ;
#38800=CARTESIAN_POINT ( 'NONE',  ( -20.66414367076832193, 17.76245163069108557, 10.99999999999809397 ) ) ;
#38812=CARTESIAN_POINT ( 'NONE',  ( -31.51573171626422010, 0.5582143012871293442, 15.13084544680214094 ) ) ;
#38838=CARTESIAN_POINT ( 'NONE',  ( 36.50335543115979675, -9.090109797569423833, 14.53008259254010959 ) ) ;
#38840=CARTESIAN_POINT ( 'NONE',  ( 16.81416712651216017, 27.17354907310114243, 13.92931973827808889 ) ) ;
#38841=CARTESIAN_POINT ( 'NONE',  ( 15.74227866054390290, -25.75916161678440375, 17.42190598798392998 ) ) ;
#38843=CARTESIAN_POINT ( 'NONE',  ( -5.712781365377792575, 28.53852268908977052, 20.69868183039818277 ) ) ;
#38853=CARTESIAN_POINT ( 'NONE',  ( 21.46287209667334039, 12.39159498259634695, 16.30093088680190405 ) ) ;
#38863=CARTESIAN_POINT ( 'NONE',  ( -30.00904163739982167, -13.36872314231684733, 19.99202127657103389 ) ) ;
#38866=ORIENTED_EDGE ( 'NONE', *, *, #6558, .F. ) ;
#38888=CARTESIAN_POINT ( 'NONE',  ( 24.23816072143611677, -22.57437281311106858, 19.27171037444157875 ) ) ;
#38910=CARTESIAN_POINT ( 'NONE',  ( -22.30415078909513227, -16.34589999308528618, 20.99999999999995026 ) ) ;
#38921=CARTESIAN_POINT ( 'NONE',  ( -26.45121176803934304, -27.84758587393085350, 11.55979286843934872 ) ) ;
#38934=CARTESIAN_POINT ( 'NONE',  ( -17.01074486384391449, 2.963432112732212520, 20.82122704794078771 ) ) ;
#38935=CARTESIAN_POINT ( 'NONE',  ( 21.38319344285460843, -17.62079982023265501, 20.94377226548386517 ) ) ;
#38951=CARTESIAN_POINT ( 'NONE',  ( 16.81416712651216017, 27.17354907310113887, 13.92931973827808712 ) ) ;
#38966=CARTESIAN_POINT ( 'NONE',  ( -23.54277854204216069, -14.22284186533119410, 22.99999999999999645 ) ) ;
#38992=CARTESIAN_POINT ( 'NONE',  ( -10.78342637327578224, 29.81468131102269936, 18.87996532025784546 ) ) ;
#38997=EDGE_CURVE ( 'NONE', #8563, #34372, #29847, .T. ) ;
#38999=CARTESIAN_POINT ( 'NONE',  ( 4.817371740575539185, 23.83900317890011422, 23.00000000000000000 ) ) ;
#39009=CARTESIAN_POINT ( 'NONE',  ( -15.27443809246124218, -27.57253143578281041, 15.13084544680213561 ) ) ;
#39031=CARTESIAN_POINT ( 'NONE',  ( 35.08890111189684546, -5.671281373296992001, 15.72805884748904681 ) ) ;
#39033=CARTESIAN_POINT ( 'NONE',  ( 8.901509289502147482, 37.28103075694621538, 14.53008259254014689 ) ) ;
#39034=CARTESIAN_POINT ( 'NONE',  ( 10.81727955709540723, -23.19337658755338083, 18.42518152271931697 ) ) ;
#39036=CARTESIAN_POINT ( 'NONE',  ( 7.341569467741936528, 26.39884405248101373, 20.69868183039782039 ) ) ;
#39046=CARTESIAN_POINT ( 'NONE',  ( 15.00309677617812554, 1.567672476142359939, 20.99999999999999645 ) ) ;
#39057=CARTESIAN_POINT ( 'NONE',  ( -32.41210168510392009, -9.609370058585097851, 18.87996532025784546 ) ) ;
#39076=CARTESIAN_POINT ( 'NONE',  ( -35.27625572565260370, 1.213838575766586603, 11.00000000000000000 ) ) ;
#39081=CARTESIAN_POINT ( 'NONE',  ( 31.52520841578668254, -13.67397774227536367, 19.27171037444156099 ) ) ;
#39104=CARTESIAN_POINT ( 'NONE',  ( -18.76090689389218014, -16.22676322417297001, 20.99999999999999645 ) ) ;
#39114=CARTESIAN_POINT ( 'NONE',  ( -32.80061120326500657, -23.42582577749657347, 12.14047268033081295 ) ) ;
#39129=CARTESIAN_POINT ( 'NONE',  ( -17.69280599717042080, 3.437614796744613344, 20.69868183039779908 ) ) ;
#39130=CARTESIAN_POINT ( 'NONE',  ( 18.03924190088524782, -16.85603499720511067, 20.99999999999999645 ) ) ;
#39134=CARTESIAN_POINT ( 'NONE',  ( 33.69589222704781406, -0.03122585499636791606, 11.55979286843971465 ) ) ;
#39146=CYLINDRICAL_SURFACE ( 'NONE', #34593, 58.00000000000007816 ) ;
#39208=CARTESIAN_POINT ( 'NONE',  ( -1.829593030691901284E-15, 22.50000000000001066, 23.00000000000000000 ) ) ;
#39211=CARTESIAN_POINT ( 'NONE',  ( -31.72789954390480105, 0.7664678198863910108, 14.53008259254011492 ) ) ;
#39226=CARTESIAN_POINT ( 'NONE',  ( -36.24879720996644039, -17.94626546700501635, 10.99999999999997691 ) ) ;
#39233=CARTESIAN_POINT ( 'NONE',  ( 24.41232237689766293, -27.78610790073912895, 14.53008259254038670 ) ) ;
#39235=CARTESIAN_POINT ( 'NONE',  ( 15.50248524335058065, 30.73390593357087397, 13.92931973827802317 ) ) ;
#39236=CARTESIAN_POINT ( 'NONE',  ( 5.531500846456773424, -21.05812563137664739, 19.27171037444156809 ) ) ;
#39238=CARTESIAN_POINT ( 'NONE',  ( 3.838817179443445138, 30.80979998870935788, 20.50957957746028981 ) ) ;
#39247=CARTESIAN_POINT ( 'NONE',  ( 17.58821720676783329, 10.15456193889309411, 19.66345542862528717 ) ) ;
#39258=CARTESIAN_POINT ( 'NONE',  ( -30.77008022630320738, -17.76511410164224003, 18.87996532025785257 ) ) ;
#39281=CARTESIAN_POINT ( 'NONE',  ( 31.66906069137291624, -9.703676519218381813, 19.27171037444156099 ) ) ;
#39298=CARTESIAN_POINT ( 'NONE',  ( -23.05386822411323422, -7.747535282638357224, 20.99999999999999645 ) ) ;
#39303=CARTESIAN_POINT ( 'NONE',  ( -10.29072928254728403, -26.28675887230140162, 15.13084544681106536 ) ) ;
#39306=CARTESIAN_POINT ( 'NONE',  ( -18.40750778688453337, -18.65192611823525581, 20.82122704794080548 ) ) ;
#39316=CARTESIAN_POINT ( 'NONE',  ( -28.21696687770289813, -27.03935558029874286, 12.14047268033091598 ) ) ;
#39334=CARTESIAN_POINT ( 'NONE',  ( 17.83459896181130944, -17.64923967996766052, 20.94377226548378701 ) ) ;
#39338=CARTESIAN_POINT ( 'NONE',  ( 36.74707368630886606, -16.71203845619553974, 10.99999999999982769 ) ) ;
#39376=CARTESIAN_POINT ( 'NONE',  ( -17.61963632530846979, 22.05541241832616706, 15.13084544681368548 ) ) ;
#39392=CARTESIAN_POINT ( 'NONE',  ( -4.444496572746359675, 24.85486536600718921, 23.00000000000000711 ) ) ;
#39423=VERTEX_POINT ( 'NONE', #27638 ) ;
#39431=CARTESIAN_POINT ( 'NONE',  ( 15.07283634909883929, -28.35394831540531158, 13.32518128616608877 ) ) ;
#39433=CARTESIAN_POINT ( 'NONE',  ( -14.44241962112810285, 32.29667252612950534, 13.92931973827808889 ) ) ;
#39435=CARTESIAN_POINT ( 'NONE',  ( -18.03924190088443424, -16.85603499720474119, 20.99999999999999645 ) ) ;
#39437=CARTESIAN_POINT ( 'NONE',  ( -6.154269285972598702, 26.67460248448161764, 20.82122704794079837 ) ) ;
#39443=EDGE_CURVE ( 'NONE', #3967, #24813, #21936, .T. ) ;
#39447=CARTESIAN_POINT ( 'NONE',  ( 10.32110568910150228, 19.34973993754613986, 20.50957957746029336 ) ) ;
#39452=ORIENTED_EDGE ( 'NONE', *, *, #17127, .T. ) ;
#39458=CARTESIAN_POINT ( 'NONE',  ( -32.53782915839244083, -12.43926102483660578, 18.87996532025785967 ) ) ;
#39475=CARTESIAN_POINT ( 'NONE',  ( 16.58691282011993806, -31.15705289668494871, 22.99999999999905853 ) ) ;
#39485=CARTESIAN_POINT ( 'NONE',  ( 29.31960910815444521, -5.098408205982018160, 19.66345542862562468 ) ) ;
#39499=DIRECTION ( 'NONE',  ( -0.000000000000000000, -0.000000000000000000, -1.000000000000000000 ) ) ;
#39504=CARTESIAN_POINT ( 'NONE',  ( -15.07283634909299685, -28.35394831540364180, 13.32518128616608877 ) ) ;
#39507=CARTESIAN_POINT ( 'NONE',  ( -27.58732789242640138, -12.88115193908558354, 20.69868183039781329 ) ) ;
#39533=CARTESIAN_POINT ( 'NONE',  ( 25.22909892406947918, -10.52103384677014120, 20.99999999999999645 ) ) ;
#39535=DIRECTION ( 'NONE',  ( 1.000000000000000000, 0.000000000000000000, 0.000000000000000000 ) ) ;
#39561=CARTESIAN_POINT ( 'NONE',  ( 30.57450045108191006, -0.3656520783221838267, 16.87380292611441490 ) ) ;
#39575=CARTESIAN_POINT ( 'NONE',  ( -28.79337657216576574, 4.963436916929316212, 11.55979286844546472 ) ) ;
#39593=FILL_AREA_STYLE ('',( #23756 ) ) ;
#39630=CARTESIAN_POINT ( 'NONE',  ( 33.26300037445852098, -0.3730773600908409704, 13.92931973827949221 ) ) ;
#39632=CARTESIAN_POINT ( 'NONE',  ( -15.23843103912111019, 30.59358247944625120, 14.53008259253998169 ) ) ;
#39634=CARTESIAN_POINT ( 'NONE',  ( -11.73759695149396620, -17.78600041308340707, 20.69868183039790566 ) ) ;
#39636=CARTESIAN_POINT ( 'NONE',  ( 6.495117285921949701, 31.04668714394701823, 19.99202127657103745 ) ) ;
#39646=CARTESIAN_POINT ( 'NONE',  ( 6.367390439425446580, 24.26983560722391786, 20.94377226548378346 ) ) ;
#39657=CARTESIAN_POINT ( 'NONE',  ( -20.47921202893386194, -24.94416275241482950, 18.42518152272108978 ) ) ;
#39684=CARTESIAN_POINT ( 'NONE',  ( 20.47921202893403247, -24.94416275241516701, 18.42518152272108622 ) ) ;
#39689=DIRECTION ( 'NONE',  ( -1.000000000000000000, 0.000000000000000000, 0.000000000000000000 ) ) ;
#39690=CARTESIAN_POINT ( 'NONE',  ( -15.60391421430763614, -26.29546805949255628, 16.87380292611442201 ) ) ;
#39699=CARTESIAN_POINT ( 'NONE',  ( -18.74997338764006471, -3.362744936731947298, 20.99999999999999645 ) ) ;
#39703=CARTESIAN_POINT ( 'NONE',  ( 4.250072516143177381E-14, -26.77689918168226058, 11.00000000000000000 ) ) ;
#39706=CARTESIAN_POINT ( 'NONE',  ( -25.00594398452541967, -16.29738563782265004, 20.82122704794080192 ) ) ;
#39730=AXIS2_PLACEMENT_3D ( 'NONE', #37768, #399, #16435 ) ;
#39732=CARTESIAN_POINT ( 'NONE',  ( 28.10500611839371743, -8.168659512009874391, 20.50957957746006599 ) ) ;
#39742=CARTESIAN_POINT ( 'NONE',  ( 11.11100267139550013, 25.58833710557466290, 19.66345542862528717 ) ) ;
#39759=ORIENTED_EDGE ( 'NONE', *, *, #10366, .T. ) ;
#39761=CARTESIAN_POINT ( 'NONE',  ( 38.42882786495224678, -4.479089870562107834, 10.99999999999999822 ) ) ;
#39772=CARTESIAN_POINT ( 'NONE',  ( -23.18947492591177095, 13.38844959084094555, 11.55979286843934872 ) ) ;
#39821=ORIENTED_EDGE ( 'NONE', *, *, #3553, .T. ) ;
#39829=CARTESIAN_POINT ( 'NONE',  ( 12.39897218486625796, 35.60749793648125205, 12.14047268033093196 ) ) ;
#39830=CARTESIAN_POINT ( 'NONE',  ( 5.869341256201768608, -17.04122685614420263, 20.69868183039781684 ) ) ;
#39832=CARTESIAN_POINT ( 'NONE',  ( -6.495117285923170947, 31.04668714394608031, 19.99202127657103389 ) ) ;
#39834=LINE ( 'NONE', #17726, #29790 ) ;
#39839=CARTESIAN_POINT ( 'NONE',  ( -17.34253826607186966, 27.32041144404028188, 11.00000000000000000 ) ) ;
#39841=CARTESIAN_POINT ( 'NONE',  ( 9.555312204549732513, 25.15592819203938291, 20.25080042701566541 ) ) ;
#39852=CARTESIAN_POINT ( 'NONE',  ( -28.78471548569087091, -2.122417091764221109, 18.87996532025785257 ) ) ;
#39862=ORIENTED_EDGE ( 'NONE', *, *, #19596, .F. ) ;
#39869=CARTESIAN_POINT ( 'NONE',  ( 33.75875814100317029, 2.759858869446390361, 11.00000000000000000 ) ) ;
#39873=EDGE_LOOP ( 'NONE', ( #13315, #13080, #16376, #23426 ) ) ;
#39875=CARTESIAN_POINT ( 'NONE',  ( 29.28423149095714351, -1.632116715644855054, 18.42518152272108978 ) ) ;
#39896=CARTESIAN_POINT ( 'NONE',  ( -15.00437666250803836, -28.61930095463306500, 12.14047268033097460 ) ) ;
#39899=CARTESIAN_POINT ( 'NONE',  ( -25.12106050720013073, -7.724475404461035311, 20.94377226548368753 ) ) ;
#39914=VERTEX_POINT ( 'NONE', #37659 ) ;
#39928=CARTESIAN_POINT ( 'NONE',  ( 24.94906875546882219, -17.45075080782927301, 20.69868183039781329 ) ) ;
#39934=CARTESIAN_POINT ( 'NONE',  ( -18.74997338763903798, -3.362744936732933176, 23.00000000000000000 ) ) ;
#39940=AXIS2_PLACEMENT_3D ( 'NONE', #34215, #6369, #28109 ) ;
#39944=CARTESIAN_POINT ( 'NONE',  ( -4.881458130668121953, -28.77689918168226058, 11.00000000000000000 ) ) ;
#39961=CARTESIAN_POINT ( 'NONE',  ( -35.26975574857812745, -18.21959598282740345, 14.53008259254033696 ) ) ;
#39971=CARTESIAN_POINT ( 'NONE',  ( -32.28722999652026715, 1.315479119632480876, 12.14047268033097282 ) ) ;
#40023=CARTESIAN_POINT ( 'NONE',  ( -1.464931600276310347E-13, 40.43805239114132632, 12.14047268033097637 ) ) ;
#40025=CARTESIAN_POINT ( 'NONE',  ( 17.83459896181356541, -17.64923967996807264, 20.94377226548378346 ) ) ;
#40027=CARTESIAN_POINT ( 'NONE',  ( 5.145977874758831838, 31.04572515098157481, 20.25080042701566896 ) ) ;
#40048=CARTESIAN_POINT ( 'NONE',  ( -33.27313359468927700, -17.33775975077042375, 17.42190598798430301 ) ) ;
#40063=CARTESIAN_POINT ( 'NONE',  ( 39.51968005975079734, -13.07391886567386763, 11.00000000000000000 ) ) ;
#40075=CARTESIAN_POINT ( 'NONE',  ( 30.63324413334751029, -19.40199358733793744, 18.42518152272108622 ) ) ;
#40081=CARTESIAN_POINT ( 'NONE',  ( 4.817371740575539185, 23.83900317890011422, 23.00000000000000000 ) ) ;
#40088=CARTESIAN_POINT ( 'NONE',  ( 22.89849980942894092, 13.22045502901191405, 13.32518128616608877 ) ) ;
#40100=CARTESIAN_POINT ( 'NONE',  ( -18.64638308222451357, -17.01267446048745668, 20.99999999999999645 ) ) ;
#40125=CARTESIAN_POINT ( 'NONE',  ( 28.21258359973596797, -14.01198379553896167, 20.50957957746030047 ) ) ;
#40142=CARTESIAN_POINT ( 'NONE',  ( -17.34253826607186966, 27.32041144404028188, 2.999999999999999112 ) ) ;
#40149=EDGE_LOOP ( 'NONE', ( #98, #17616, #22380, #5539 ) ) ;
#40162=CARTESIAN_POINT ( 'NONE',  ( -24.41232237690015339, -27.78610790073776471, 14.53008259254036716 ) ) ;
#40172=CARTESIAN_POINT ( 'NONE',  ( -16.52773037516168486, 27.09393310378289854, 14.53008259254011136 ) ) ;
#40175=CARTESIAN_POINT ( 'NONE',  ( 22.38136799084939810, -15.36239294196588290, 23.00000000000000355 ) ) ;
ENDSEC;
END-ISO-10303-21;
